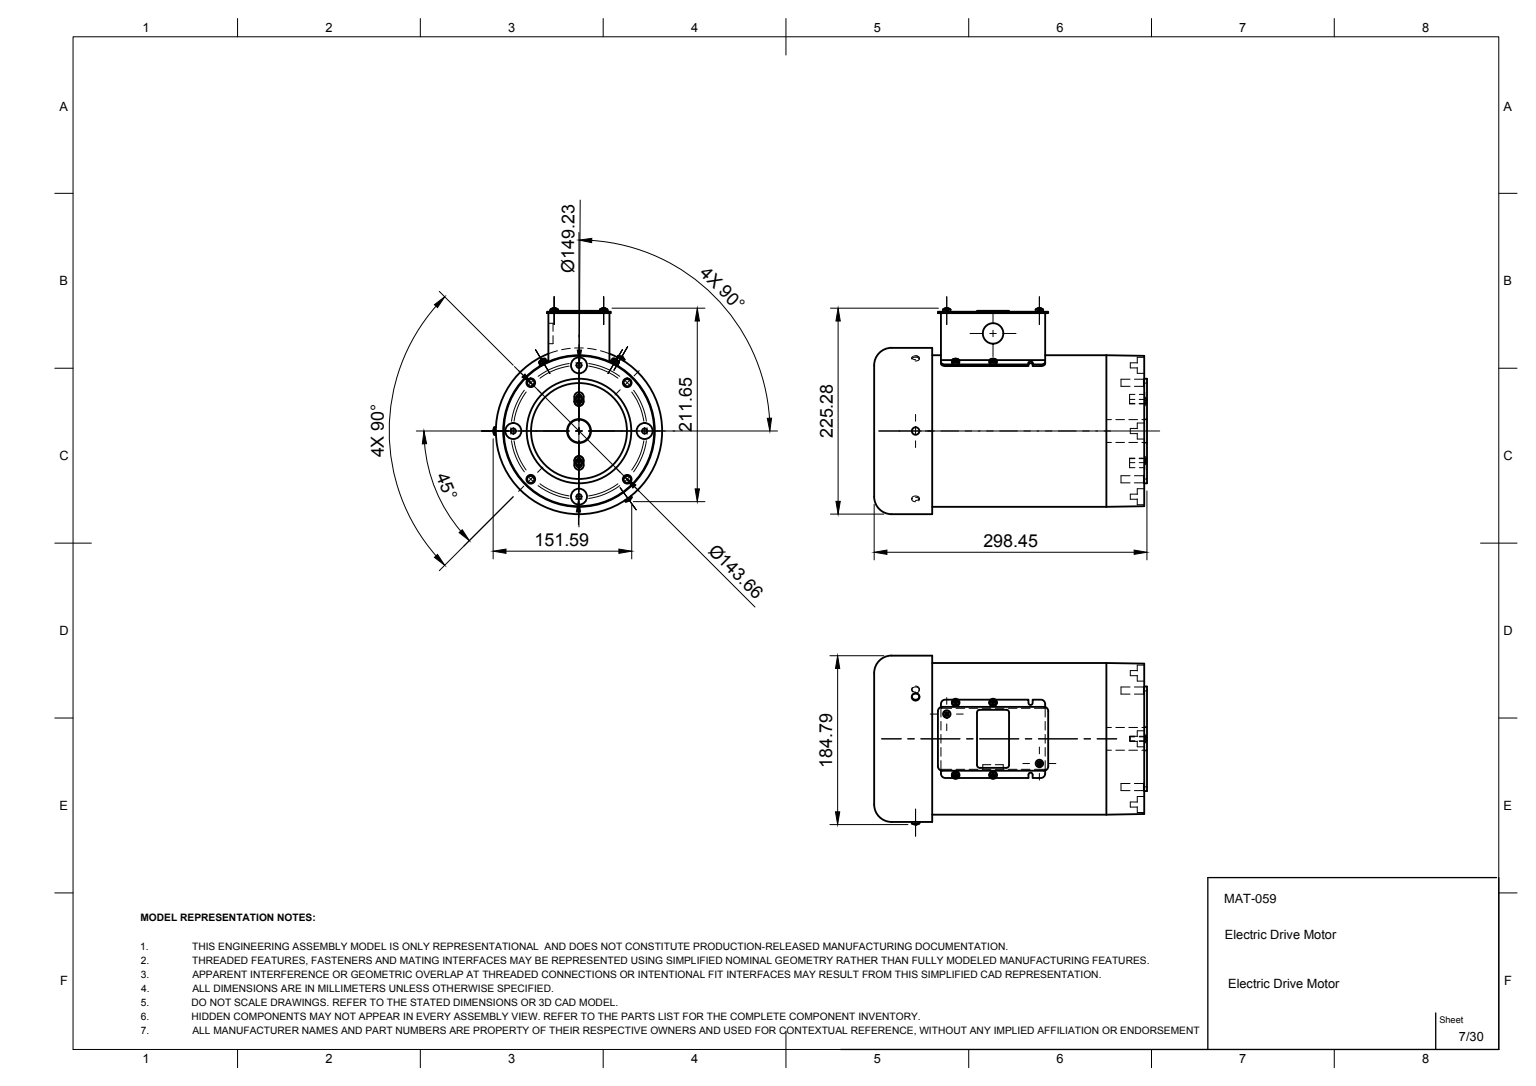
ISO-10303-21;
HEADER;
/* Generated by software containing ST-Developer
 * from STEP Tools, Inc. (www.steptools.com) 
 */

FILE_DESCRIPTION(
/* description */ ('', 'CAx-IF Rec.Pracs.---Representation and Presentation of Product Manufa
cturing Information (PMI)---4.0---2014-10-13'),
/* implementation_level */ '2;1');

FILE_NAME(
/* name */ 'Electric Drive Motor.step',
/* time_stamp */ '2026-10-28T23:00:48+01:00',
/* author */ (''),
/* organization */ (''),
/* preprocessor_version */ 'ST-DEVELOPER v20.2',
/* originating_system */ 'Autodesk Translation Framework v15.17.0.0',
/* authorisation */ '');

FILE_SCHEMA (('AP242_MANAGED_MODEL_BASED_3D_ENGINEERING_MIM_LF { 1 0 10303 442 2 1 4 }'));
ENDSEC;

DATA;
#10=MECHANICAL_DESIGN_GEOMETRIC_PRESENTATION_REPRESENTATION('',(#969),#61811);
#509=(
BOUNDED_CURVE()
B_SPLINE_CURVE(2,(#51599,#51600,#51601),.UNSPECIFIED.,.F.,.F.)
B_SPLINE_CURVE_WITH_KNOTS((3,3),(-1.09670001953998,-0.838836123214499),
 .UNSPECIFIED.)
CURVE()
GEOMETRIC_REPRESENTATION_ITEM()
RATIONAL_B_SPLINE_CURVE((0.975084512183132,0.979302933905043,1.))
REPRESENTATION_ITEM('')
);
#510=(
BOUNDED_CURVE()
B_SPLINE_CURVE(2,(#52725,#52726,#52727,#52728,#52729),.UNSPECIFIED.,.F.,
 .F.)
B_SPLINE_CURVE_WITH_KNOTS((3,2,3),(4.71238779043687,5.49778654880823,6.28318530717959),
 .UNSPECIFIED.)
CURVE()
GEOMETRIC_REPRESENTATION_ITEM()
RATIONAL_B_SPLINE_CURVE((1.,0.923879418659198,1.,0.923879418650411,1.))
REPRESENTATION_ITEM('')
);
#578=CONICAL_SURFACE('',#34877,3.98868900000005,0.78539816339748);
#579=CONICAL_SURFACE('',#34884,3.98868900000002,0.785398163397457);
#580=CONICAL_SURFACE('',#34891,3.98868900000004,0.785398163397464);
#581=CONICAL_SURFACE('',#34898,3.98868900000001,0.785398163397455);
#582=CONICAL_SURFACE('',#34900,82.8587325401841,0.0174532925199438);
#726=SPHERICAL_SURFACE('',#34596,6.41240517241364);
#727=SPHERICAL_SURFACE('',#34645,6.41240517241439);
#728=SPHERICAL_SURFACE('',#34685,6.4992807017556);
#729=SPHERICAL_SURFACE('',#34700,6.49928070175542);
#730=SPHERICAL_SURFACE('',#34786,6.41240517241381);
#731=SPHERICAL_SURFACE('',#34971,5.68734575000013);
#732=SPHERICAL_SURFACE('',#34992,5.68734575000012);
#778=B_SPLINE_CURVE_WITH_KNOTS('',3,(#51594,#51595,#51596,#51597),
 .UNSPECIFIED.,.F.,.F.,(4,4),(3.08084590110894,3.12989709501739),
 .UNSPECIFIED.);
#779=B_SPLINE_CURVE_WITH_KNOTS('',3,(#51606,#51607,#51608,#51609),
 .UNSPECIFIED.,.F.,.F.,(4,4),(3.03179470720155,3.08084590110894),
 .UNSPECIFIED.);
#780=B_SPLINE_CURVE_WITH_KNOTS('',3,(#51611,#51612,#51613,#51614,#51615,
#51616,#51617,#51618),.UNSPECIFIED.,.F.,.F.,(4,2,2,4),(-0.281543316074503,
-0.256347073285161,-0.128173536642581,-0.0492557161192092),
 .UNSPECIFIED.);
#781=B_SPLINE_CURVE_WITH_KNOTS('',3,(#51620,#51621,#51622,#51623,#51624,
#51625,#51626,#51627),.UNSPECIFIED.,.F.,.F.,(4,2,2,4),(-3.44463382971284,
-3.36571600918869,-3.23754247254589,-3.21234622975666),.UNSPECIFIED.);
#782=B_SPLINE_CURVE_WITH_KNOTS('',3,(#51629,#51630,#51631,#51632,#51633,
#51634,#51635),.UNSPECIFIED.,.F.,.F.,(4,3,4),(-0.0490511939078948,0.,0.0490511939079084),
 .UNSPECIFIED.);
#783=B_SPLINE_CURVE_WITH_KNOTS('',3,(#51637,#51638,#51639,#51640,#51641,
#51642,#51643,#51644),.UNSPECIFIED.,.F.,.F.,(4,2,2,4),(-0.281543316073918,
-0.256347073285632,-0.128173536642816,-0.0492557161186468),
 .UNSPECIFIED.);
#784=B_SPLINE_CURVE_WITH_KNOTS('',3,(#51646,#51647,#51648,#51649,#51650,
#51651,#51652,#51653),.UNSPECIFIED.,.F.,.F.,(4,2,2,4),(-3.44463382971226,
-3.36571600918894,-3.23754247254636,-3.21234622975697),.UNSPECIFIED.);
#785=B_SPLINE_CURVE_WITH_KNOTS('',3,(#51655,#51656,#51657,#51658,#51659,
#51660,#51661),.UNSPECIFIED.,.F.,.F.,(4,3,4),(-0.0490511939073931,0.,0.0490511939084528),
 .UNSPECIFIED.);
#786=B_SPLINE_CURVE_WITH_KNOTS('',3,(#51663,#51664,#51665,#51666,#51667,
#51668,#51669,#51670),.UNSPECIFIED.,.F.,.F.,(4,2,2,4),(-0.281543316074568,
-0.256347073286048,-0.128173536643024,-0.0492557161192777),
 .UNSPECIFIED.);
#787=B_SPLINE_CURVE_WITH_KNOTS('',3,(#51672,#51673,#51674,#51675,#51676,
#51677,#51678,#51679),.UNSPECIFIED.,.F.,.F.,(4,2,2,4),(-3.44463382971165,
-3.36571600918866,-3.23754247254584,-3.21234622975546),.UNSPECIFIED.);
#788=B_SPLINE_CURVE_WITH_KNOTS('',3,(#51681,#51682,#51683,#51684,#51685,
#51686,#51687),.UNSPECIFIED.,.F.,.F.,(4,3,4),(-0.0490511939080049,0.,0.0490511939079151),
 .UNSPECIFIED.);
#789=B_SPLINE_CURVE_WITH_KNOTS('',3,(#51689,#51690,#51691,#51692,#51693,
#51694,#51695,#51696),.UNSPECIFIED.,.F.,.F.,(4,2,2,4),(-0.281543316075136,
-0.25634707328559,-0.128173536642795,-0.049255716119827),.UNSPECIFIED.);
#790=B_SPLINE_CURVE_WITH_KNOTS('',3,(#51697,#51698,#51699,#51700,#51701,
#51702,#51703,#51704),.UNSPECIFIED.,.F.,.F.,(4,2,2,4),(-3.44463382971222,
-3.36571600918842,-3.23754247254539,-3.21234622975693),.UNSPECIFIED.);
#791=B_SPLINE_CURVE_WITH_KNOTS('',3,(#51727,#51728,#51729,#51730,#51731,
#51732,#51733,#51734,#51735,#51736),.UNSPECIFIED.,.F.,.F.,(4,2,2,2,4),(-1.23367624376484,
-1.07962569003998,-0.925575136315127,-0.771400514278829,-0.617225892242532),
 .UNSPECIFIED.);
#792=B_SPLINE_CURVE_WITH_KNOTS('',3,(#51737,#51738,#51739,#51740,#51741,
#51742,#51743,#51744,#51745,#51746),.UNSPECIFIED.,.F.,.F.,(4,2,2,2,4),(-1.85012659645245,
-1.69593736206289,-1.54174812767333,-1.38771218571909,-1.23367624376484),
 .UNSPECIFIED.);
#793=B_SPLINE_CURVE_WITH_KNOTS('',3,(#51752,#51753,#51754,#51755,#51756,
#51757,#51758,#51759,#51760,#51761),.UNSPECIFIED.,.F.,.F.,(4,2,2,2,4),(2.30953959739069,
2.51054404549657,2.71154849360245,2.89942800416522,3.08730751472799),
 .UNSPECIFIED.);
#794=B_SPLINE_CURVE_WITH_KNOTS('',3,(#51767,#51768,#51769,#51770,#51771,
#51772,#51773,#51774,#51775,#51776,#51777,#51778,#51779,#51780,#51781,#51782,
#51783,#51784),.UNSPECIFIED.,.F.,.F.,(4,2,2,2,2,2,2,2,4),(0.368633646558617,
0.466000906670528,0.563368166782438,0.648915734055293,0.734463301328148,
0.820010868601003,0.905558435873858,1.00292569598577,1.10029295609768),
 .UNSPECIFIED.);
#795=B_SPLINE_CURVE_WITH_KNOTS('',3,(#51790,#51791,#51792,#51793,#51794,
#51795,#51796,#51797,#51798,#51799),.UNSPECIFIED.,.F.,.F.,(4,2,2,2,4),(-1.77635683940028E-15,
0.181238959345487,0.362477918690977,0.570076776395974,0.777675634100972),
 .UNSPECIFIED.);
#796=B_SPLINE_CURVE_WITH_KNOTS('',3,(#51805,#51806,#51807,#51808,#51809,
#51810,#51811,#51812,#51813,#51814),.UNSPECIFIED.,.F.,.F.,(4,2,2,2,4),(0.617225892242314,
0.771400514278674,0.925575136315034,1.07962569003995,1.23367624376487),
 .UNSPECIFIED.);
#797=B_SPLINE_CURVE_WITH_KNOTS('',3,(#51817,#51818,#51819,#51820,#51821,
#51822,#51823,#51824,#51825,#51826),.UNSPECIFIED.,.F.,.F.,(4,2,2,2,4),(1.23367624376487,
1.38771218571906,1.54174812767325,1.69593736206276,1.85012659645227),
 .UNSPECIFIED.);
#798=B_SPLINE_CURVE_WITH_KNOTS('',3,(#51832,#51833,#51834,#51835,#51836,
#51837,#51838,#51839,#51840,#51841,#51842,#51843,#51844,#51845,#51846,#51847,
#51848,#51849,#51850),.UNSPECIFIED.,.F.,.F.,(4,2,2,2,3,2,2,2,4),(-0.366794796562496,
-0.268922616838031,-0.171050437113567,-0.0855252185567822,2.33146835171283E-15,
0.0855252185567869,0.171050437113571,0.268922616838036,0.366794796562501),
 .UNSPECIFIED.);
#799=B_SPLINE_CURVE_WITH_KNOTS('',3,(#51854,#51855,#51856,#51857,#51858,
#51859,#51860,#51861,#51862,#51863,#51864,#51865,#51866,#51867,#51868,#51869,
#51870,#51871,#51872),.UNSPECIFIED.,.F.,.F.,(4,2,2,2,3,2,2,2,4),(-0.365829654769541,
-0.268462394657629,-0.171095134545717,-0.0855475672728611,-5.21804821573824E-15,
0.0882774493987044,0.176554898797414,0.271203483898993,0.365852069000572),
 .UNSPECIFIED.);
#800=B_SPLINE_CURVE_WITH_KNOTS('',3,(#51876,#51877,#51878,#51879,#51880,
#51881,#51882,#51883,#51884,#51885,#51886,#51887,#51888,#51889,#51890,#51891,
#51892,#51893),.UNSPECIFIED.,.F.,.F.,(4,2,2,2,2,2,2,2,4),(-1.10334360967883,
-1.00547142995437,-0.907599250229903,-0.822074031673119,-0.736548813116335,
-0.651023594559552,-0.565498376002768,-0.467626196278304,-0.369754016553839),
 .UNSPECIFIED.);
#801=B_SPLINE_CURVE_WITH_KNOTS('',3,(#51900,#51901,#51902,#51903,#51904,
#51905,#51906,#51907,#51908,#51909),.UNSPECIFIED.,.F.,.F.,(4,2,2,2,4),(0.,
0.181230618131972,0.362461236263944,0.571238472910728,0.780015709557511),
 .UNSPECIFIED.);
#802=B_SPLINE_CURVE_WITH_KNOTS('',3,(#51912,#51913,#51914,#51915,#51916,
#51917,#51918,#51919,#51920,#51921),.UNSPECIFIED.,.F.,.F.,(4,2,2,2,4),(-2.32129720255586,
-2.11369834485087,-1.90609948714587,-1.72486052780038,-1.54362156845489),
 .UNSPECIFIED.);
#803=B_SPLINE_CURVE_WITH_KNOTS('',3,(#51939,#51940,#51941,#51942,#51943,
#51944,#51945,#51946,#51947,#51948),.UNSPECIFIED.,.F.,.F.,(4,2,2,2,4),(-1.85012659645253,
-1.69593736206296,-1.54174812767339,-1.38771218571914,-1.23367624376489),
 .UNSPECIFIED.);
#804=B_SPLINE_CURVE_WITH_KNOTS('',3,(#51952,#51953,#51954,#51955,#51956,
#51957,#51958,#51959,#51960,#51961),.UNSPECIFIED.,.F.,.F.,(4,2,2,2,4),(-1.23367624376489,
-1.07962569004007,-0.925575136315257,-0.771400514279,-0.617225892242743),
 .UNSPECIFIED.);
#805=B_SPLINE_CURVE_WITH_KNOTS('',3,(#51971,#51972,#51973,#51974,#51975,
#51976,#51977,#51978,#51979,#51980),.UNSPECIFIED.,.F.,.F.,(4,2,2,2,4),(1.54359366303678,
1.73147317359955,1.91935268416232,2.1203571322682,2.32136158037408),
 .UNSPECIFIED.);
#806=B_SPLINE_CURVE_WITH_KNOTS('',3,(#51989,#51990,#51991,#51992,#51993,
#51994,#51995,#51996,#51997,#51998),.UNSPECIFIED.,.F.,.F.,(4,2,2,2,4),(1.23367624376487,
1.38771218571901,1.54174812767315,1.69593736206261,1.85012659645207),
 .UNSPECIFIED.);
#807=B_SPLINE_CURVE_WITH_KNOTS('',3,(#51999,#52000,#52001,#52002,#52003,
#52004,#52005,#52006,#52007,#52008),.UNSPECIFIED.,.F.,.F.,(4,2,2,2,4),(0.617225892242314,
0.771400514278675,0.925575136315035,1.07962569003995,1.23367624376487),
 .UNSPECIFIED.);
#808=B_SPLINE_CURVE_WITH_KNOTS('',3,(#52138,#52139,#52140,#52141,#52142,
#52143,#52144,#52145,#52146,#52147),.UNSPECIFIED.,.F.,.F.,(4,2,2,2,4),(1.54763785217733,
1.73581526281001,1.92399267344269,2.12587396957551,2.32775526570834),
 .UNSPECIFIED.);
#809=B_SPLINE_CURVE_WITH_KNOTS('',3,(#52454,#52455,#52456,#52457,#52458,
#52459,#52460,#52461,#52462,#52463),.UNSPECIFIED.,.F.,.F.,(4,2,2,2,4),(0.767622142619809,
0.976399379266592,1.18517661591337,1.36640723404535,1.54763785217732),
 .UNSPECIFIED.);
#810=B_SPLINE_CURVE_WITH_KNOTS('',3,(#52478,#52479,#52480,#52481,#52482,
#52483,#52484,#52485,#52486,#52487),.UNSPECIFIED.,.F.,.F.,(4,2,2,2,4),(2.31525999479713,
2.52403723144391,2.73281446809069,2.91404508622267,3.09527570435464),
 .UNSPECIFIED.);
#811=B_SPLINE_CURVE_WITH_KNOTS('',3,(#52630,#52631,#52632,#52633,#52634,
#52635,#52636,#52637,#52638,#52639,#52640,#52641,#52642,#52643,#52644,#52645,
#52646,#52647),.UNSPECIFIED.,.F.,.F.,(4,2,2,2,2,2,2,2,4),(-1.24400278846932,
-1.08850242875974,-0.933002069050166,-0.777501731642414,-0.622001394234663,
-0.46650105682691,-0.311000719419158,-0.155500359709579,0.),
 .UNSPECIFIED.);
#812=B_SPLINE_CURVE_WITH_KNOTS('',3,(#52653,#52654,#52655,#52656,#52657,
#52658,#52659,#52660,#52661,#52662,#52663,#52664,#52665,#52666,#52667,#52668,
#52669,#52670),.UNSPECIFIED.,.F.,.F.,(4,2,2,2,2,2,2,2,4),(0.,0.155500359709579,
0.311000719419159,0.46650105682691,0.622001394234662,0.777501731642413,
0.933002069050164,1.08850242875974,1.24400278846933),.UNSPECIFIED.);
#813=B_SPLINE_CURVE_WITH_KNOTS('',3,(#52679,#52680,#52681,#52682,#52683,
#52684,#52685,#52686,#52687,#52688,#52689,#52690,#52691,#52692,#52693,#52694,
#52695,#52696),.UNSPECIFIED.,.F.,.F.,(4,2,2,2,2,2,2,2,4),(-1.24400278846934,
-1.08850242875976,-0.933002069050176,-0.777501731642423,-0.622001394234669,
-0.466501056826915,-0.311000719419162,-0.155500359709581,0.),
 .UNSPECIFIED.);
#814=B_SPLINE_CURVE_WITH_KNOTS('',3,(#52702,#52703,#52704,#52705,#52706,
#52707,#52708,#52709,#52710,#52711,#52712,#52713,#52714,#52715,#52716,#52717,
#52718,#52719),.UNSPECIFIED.,.F.,.F.,(4,2,2,2,2,2,2,2,4),(0.,0.155500359709582,
0.311000719419163,0.466501056826916,0.622001394234669,0.777501731642423,
0.933002069050176,1.08850242875976,1.24400278846934),.UNSPECIFIED.);
#815=B_SPLINE_CURVE_WITH_KNOTS('',3,(#52734,#52735,#52736,#52737,#52738,
#52739,#52740,#52741,#52742,#52743,#52744,#52745,#52746,#52747,#52748,#52749,
#52750,#52751),.UNSPECIFIED.,.F.,.F.,(4,2,2,2,2,2,2,2,4),(-1.24400278846932,
-1.08850242875974,-0.933002069050164,-0.777501731642413,-0.622001394234661,
-0.46650105682691,-0.311000719419158,-0.155500359709579,0.),
 .UNSPECIFIED.);
#816=B_SPLINE_CURVE_WITH_KNOTS('',3,(#52755,#52756,#52757,#52758,#52759,
#52760,#52761,#52762,#52763,#52764,#52765,#52766,#52767,#52768,#52769,#52770,
#52771,#52772),.UNSPECIFIED.,.F.,.F.,(4,2,2,2,2,2,2,2,4),(0.,0.15550035970958,
0.311000719419159,0.466501056826911,0.622001394234662,0.777501731642413,
0.933002069050165,1.08850242875974,1.24400278846932),.UNSPECIFIED.);
#870=(
BOUNDED_SURFACE()
B_SPLINE_SURFACE(2,2,((#51565,#51566,#51567,#51568,#51569,#51570,#51571,
#51572,#51573),(#51574,#51575,#51576,#51577,#51578,#51579,#51580,#51581,
#51582),(#51583,#51584,#51585,#51586,#51587,#51588,#51589,#51590,#51591)),
 .UNSPECIFIED.,.F.,.T.,.F.)
B_SPLINE_SURFACE_WITH_KNOTS((3,3),(3,2,2,2,3),(-1.48658674941058,-0.838836123214499),
(-3.14159265358979,-1.5707963267949,0.,1.5707963267949,3.14159265358979),
 .UNSPECIFIED.)
GEOMETRIC_REPRESENTATION_ITEM()
RATIONAL_B_SPLINE_SURFACE(((1.,0.707106781186548,1.,0.707106781186548,1.,
0.707106781186548,1.,0.707106781186548,1.),(0.948009249396791,0.67034376887604,
0.948009249396791,0.67034376887604,0.948009249396791,0.67034376887604,0.948009249396791,
0.67034376887604,0.948009249396791),(1.,0.707106781186548,1.,0.707106781186548,
1.,0.707106781186548,1.,0.707106781186548,1.)))
REPRESENTATION_ITEM('')
SURFACE()
);
#871=(
BOUNDED_SURFACE()
B_SPLINE_SURFACE(2,2,((#52773,#52774,#52775,#52776,#52777,#52778,#52779,
#52780,#52781),(#52782,#52783,#52784,#52785,#52786,#52787,#52788,#52789,
#52790),(#52791,#52792,#52793,#52794,#52795,#52796,#52797,#52798,#52799)),
 .UNSPECIFIED.,.F.,.T.,.F.)
B_SPLINE_SURFACE_WITH_KNOTS((3,3),(3,2,2,2,3),(-1.57079634483717,-0.955666854650568),
(-3.14159265358979,-1.5707963267949,0.,1.5707963267949,3.14159265358979),
 .UNSPECIFIED.)
GEOMETRIC_REPRESENTATION_ITEM()
RATIONAL_B_SPLINE_SURFACE(((1.,0.707106781186548,1.,0.707106781186548,1.,
0.707106781186548,1.,0.707106781186548,1.),(0.953073640802859,0.673924834381854,
0.953073640802859,0.673924834381854,0.953073640802859,0.673924834381854,
0.953073640802859,0.673924834381854,0.953073640802859),(1.,0.707106781186548,
1.,0.707106781186548,1.,0.707106781186548,1.,0.707106781186548,1.)))
REPRESENTATION_ITEM('')
SURFACE()
);
#872=(
BOUNDED_SURFACE()
B_SPLINE_SURFACE(2,2,((#52806,#52807,#52808,#52809,#52810,#52811,#52812,
#52813,#52814),(#52815,#52816,#52817,#52818,#52819,#52820,#52821,#52822,
#52823),(#52824,#52825,#52826,#52827,#52828,#52829,#52830,#52831,#52832)),
 .UNSPECIFIED.,.F.,.T.,.F.)
B_SPLINE_SURFACE_WITH_KNOTS((3,3),(3,2,2,2,3),(-1.57079630698122,-0.955666850767325),
(-3.14159265358979,-1.5707963267949,0.,1.5707963267949,3.14159265358979),
 .UNSPECIFIED.)
GEOMETRIC_REPRESENTATION_ITEM()
RATIONAL_B_SPLINE_SURFACE(((1.,0.707106781186548,1.,0.707106781186548,1.,
0.707106781186548,1.,0.707106781186548,1.),(0.953073645945215,0.673924838018048,
0.953073645945215,0.673924838018048,0.953073645945215,0.673924838018048,
0.953073645945215,0.673924838018048,0.953073645945215),(1.,0.707106781186548,
1.,0.707106781186548,1.,0.707106781186548,1.,0.707106781186548,1.)))
REPRESENTATION_ITEM('')
SURFACE()
);
#873=(
BOUNDED_SURFACE()
B_SPLINE_SURFACE(2,2,((#52834,#52835,#52836,#52837,#52838,#52839,#52840,
#52841,#52842),(#52843,#52844,#52845,#52846,#52847,#52848,#52849,#52850,
#52851),(#52852,#52853,#52854,#52855,#52856,#52857,#52858,#52859,#52860)),
 .UNSPECIFIED.,.F.,.T.,.F.)
B_SPLINE_SURFACE_WITH_KNOTS((3,3),(3,2,2,2,3),(-1.57079632708437,-0.955666871754965),
(-3.14159265358979,-1.5707963267949,0.,1.5707963267949,3.14159265358979),
 .UNSPECIFIED.)
GEOMETRIC_REPRESENTATION_ITEM()
RATIONAL_B_SPLINE_SURFACE(((1.,0.707106781186548,1.,0.707106781186548,1.,
0.707106781186548,1.,0.707106781186548,1.),(0.953073646079135,0.673924838112744,
0.953073646079135,0.673924838112744,0.953073646079135,0.673924838112744,
0.953073646079135,0.673924838112744,0.953073646079135),(1.,0.707106781186548,
1.,0.707106781186548,1.,0.707106781186548,1.,0.707106781186548,1.)))
REPRESENTATION_ITEM('')
SURFACE()
);
#895=TOROIDAL_SURFACE('',#34831,71.8820000000001,19.0499999999999);
#919=SHAPE_REPRESENTATION_RELATIONSHIP('SRR','None',#61977,#944);
#944=ADVANCED_BREP_SHAPE_REPRESENTATION('',(#1008),#61790);
#969=STYLED_ITEM('',(#62142),#1008);
#1008=MANIFOLD_SOLID_BREP('Body1',#33799);
#1107=CYLINDRICAL_SURFACE('',#34576,4.08939999999975);
#1108=CYLINDRICAL_SURFACE('',#34577,84.4550000000046);
#1109=CYLINDRICAL_SURFACE('',#34582,2.286);
#1110=CYLINDRICAL_SURFACE('',#34583,2.286);
#1111=CYLINDRICAL_SURFACE('',#34584,4.82600000000001);
#1112=CYLINDRICAL_SURFACE('',#34587,4.08939999999991);
#1113=CYLINDRICAL_SURFACE('',#34590,84.455000000012);
#1114=CYLINDRICAL_SURFACE('',#34615,4.08939999999986);
#1115=CYLINDRICAL_SURFACE('',#34617,4.08939999999985);
#1116=CYLINDRICAL_SURFACE('',#34647,4.82600000000001);
#1117=CYLINDRICAL_SURFACE('',#34648,4.826);
#1118=CYLINDRICAL_SURFACE('',#34652,4.82599999999999);
#1119=CYLINDRICAL_SURFACE('',#34656,4.82600000000005);
#1120=CYLINDRICAL_SURFACE('',#34660,4.82600000000005);
#1121=CYLINDRICAL_SURFACE('',#34672,3.04799999999982);
#1122=CYLINDRICAL_SURFACE('',#34675,3.04799999999992);
#1123=CYLINDRICAL_SURFACE('',#34678,3.048);
#1124=CYLINDRICAL_SURFACE('',#34681,3.04800000000001);
#1125=CYLINDRICAL_SURFACE('',#34699,4.08940000000001);
#1126=CYLINDRICAL_SURFACE('',#34714,4.0894);
#1127=CYLINDRICAL_SURFACE('',#34751,4.826);
#1128=CYLINDRICAL_SURFACE('',#34757,4.826);
#1129=CYLINDRICAL_SURFACE('',#34781,11.1759999999998);
#1130=CYLINDRICAL_SURFACE('',#34811,4.12749999999997);
#1131=CYLINDRICAL_SURFACE('',#34817,4.12750000000001);
#1132=CYLINDRICAL_SURFACE('',#34823,4.12749999999996);
#1133=CYLINDRICAL_SURFACE('',#34836,90.9319999999999);
#1134=CYLINDRICAL_SURFACE('',#34840,82.931);
#1135=CYLINDRICAL_SURFACE('',#34855,5.08000000000016);
#1136=CYLINDRICAL_SURFACE('',#34858,5.08000000000021);
#1137=CYLINDRICAL_SURFACE('',#34866,5.08);
#1138=CYLINDRICAL_SURFACE('',#34869,5.08000000000001);
#1139=CYLINDRICAL_SURFACE('',#34874,3.90270999999991);
#1140=CYLINDRICAL_SURFACE('',#34881,3.90270999999999);
#1141=CYLINDRICAL_SURFACE('',#34888,3.90271000000012);
#1142=CYLINDRICAL_SURFACE('',#34895,3.90271);
#1143=CYLINDRICAL_SURFACE('',#34908,57.15);
#1144=CYLINDRICAL_SURFACE('',#34912,52.451);
#1145=CYLINDRICAL_SURFACE('',#34916,13.081);
#1146=CYLINDRICAL_SURFACE('',#34920,12.446);
#1147=CYLINDRICAL_SURFACE('',#34924,8.76299999999995);
#1148=CYLINDRICAL_SURFACE('',#34925,2.794);
#1149=CYLINDRICAL_SURFACE('',#34928,8.76299999999997);
#1150=CYLINDRICAL_SURFACE('',#34932,2.794);
#1151=CYLINDRICAL_SURFACE('',#34937,2.79400000000002);
#1152=CYLINDRICAL_SURFACE('',#34941,8.76300000000001);
#1153=CYLINDRICAL_SURFACE('',#34942,8.763);
#1154=CYLINDRICAL_SURFACE('',#34946,2.79399999999998);
#1155=CYLINDRICAL_SURFACE('',#34950,2.76860000000046);
#1156=CYLINDRICAL_SURFACE('',#34958,2.7686);
#1157=CYLINDRICAL_SURFACE('',#34960,2.76860000000001);
#1158=CYLINDRICAL_SURFACE('',#34961,2.76860000000061);
#1159=CYLINDRICAL_SURFACE('',#34965,4.73709999999997);
#1160=CYLINDRICAL_SURFACE('',#34968,2.18439999999999);
#1161=CYLINDRICAL_SURFACE('',#34989,2.18440000000006);
#1162=CYLINDRICAL_SURFACE('',#34990,4.73710000000002);
#1923=FACE_BOUND('',#6409,.T.);
#1924=FACE_BOUND('',#6410,.T.);
#1925=FACE_BOUND('',#6418,.T.);
#1926=FACE_BOUND('',#6419,.T.);
#1927=FACE_BOUND('',#6422,.T.);
#1928=FACE_BOUND('',#6442,.T.);
#1929=FACE_BOUND('',#6454,.T.);
#1930=FACE_BOUND('',#6456,.T.);
#1931=FACE_BOUND('',#6457,.T.);
#1932=FACE_BOUND('',#6458,.T.);
#1933=FACE_BOUND('',#6469,.T.);
#1934=FACE_BOUND('',#6472,.T.);
#1935=FACE_BOUND('',#6521,.T.);
#1936=FACE_BOUND('',#6539,.T.);
#1937=FACE_BOUND('',#6552,.T.);
#1938=FACE_BOUND('',#6564,.T.);
#1939=FACE_BOUND('',#6565,.T.);
#1940=FACE_BOUND('',#6566,.T.);
#1941=FACE_BOUND('',#6570,.T.);
#1942=FACE_BOUND('',#6577,.T.);
#1943=FACE_BOUND('',#6583,.T.);
#1944=FACE_BOUND('',#6602,.T.);
#1945=FACE_BOUND('',#6603,.T.);
#1946=FACE_BOUND('',#6604,.T.);
#1947=FACE_BOUND('',#6605,.T.);
#1948=FACE_BOUND('',#6606,.T.);
#1949=FACE_BOUND('',#6607,.T.);
#1950=FACE_BOUND('',#6608,.T.);
#1951=FACE_BOUND('',#6609,.T.);
#1952=FACE_BOUND('',#6610,.T.);
#1953=FACE_BOUND('',#6613,.T.);
#1954=FACE_BOUND('',#6616,.T.);
#1955=FACE_BOUND('',#6617,.T.);
#1956=FACE_BOUND('',#6618,.T.);
#1957=FACE_BOUND('',#6621,.T.);
#1958=FACE_BOUND('',#6624,.T.);
#1959=FACE_BOUND('',#6630,.T.);
#1960=FACE_BOUND('',#6636,.T.);
#1961=FACE_BOUND('',#6640,.T.);
#1962=FACE_BOUND('',#6647,.T.);
#1963=FACE_BOUND('',#6652,.T.);
#1964=FACE_BOUND('',#6656,.T.);
#1965=FACE_BOUND('',#6658,.T.);
#1966=FACE_BOUND('',#6660,.T.);
#1967=FACE_BOUND('',#6664,.T.);
#2448=CIRCLE('',#34569,4.08939999999988);
#2449=CIRCLE('',#34570,4.08939999999988);
#2450=CIRCLE('',#34575,4.0893999999995);
#2451=CIRCLE('',#34578,84.4550000000159);
#2452=CIRCLE('',#34579,84.4549999999612);
#2453=CIRCLE('',#34580,84.4549999999434);
#2454=CIRCLE('',#34581,84.4550000000244);
#2455=CIRCLE('',#34588,4.08940000000003);
#2456=CIRCLE('',#34589,4.08939999999987);
#2457=CIRCLE('',#34591,84.4549999999862);
#2458=CIRCLE('',#34592,84.4550000001664);
#2459=CIRCLE('',#34593,84.4550000000658);
#2460=CIRCLE('',#34594,84.4549999999639);
#2461=CIRCLE('',#34597,5.73418625921224);
#2462=CIRCLE('',#34598,6.39225125407266);
#2463=CIRCLE('',#34599,6.39225125407329);
#2464=CIRCLE('',#34600,5.73418625920595);
#2465=CIRCLE('',#34601,6.39225125407447);
#2466=CIRCLE('',#34602,6.39225125407165);
#2467=CIRCLE('',#34603,5.73418625919979);
#2468=CIRCLE('',#34604,6.39225125407114);
#2469=CIRCLE('',#34605,6.39225125407334);
#2470=CIRCLE('',#34606,5.73418625920593);
#2471=CIRCLE('',#34607,6.3922512540724);
#2472=CIRCLE('',#34608,6.39225125407298);
#2473=CIRCLE('',#34610,6.3922512540739);
#2474=CIRCLE('',#34612,5.73418625919449);
#2475=CIRCLE('',#34614,4.08939999999995);
#2476=CIRCLE('',#34616,4.08939999999987);
#2477=CIRCLE('',#34618,4.08939999999931);
#2478=CIRCLE('',#34619,4.08939999999987);
#2479=CIRCLE('',#34621,6.39225125406976);
#2480=CIRCLE('',#34623,5.7341862591997);
#2481=CIRCLE('',#34625,6.39225125407312);
#2482=CIRCLE('',#34627,6.39225125407987);
#2483=CIRCLE('',#34629,5.73418625919762);
#2484=CIRCLE('',#34631,6.39225125407758);
#2485=CIRCLE('',#34633,6.39225125407361);
#2486=CIRCLE('',#34635,5.73418625916851);
#2487=CIRCLE('',#34637,6.39225125407298);
#2488=CIRCLE('',#34639,6.39225125407049);
#2489=CIRCLE('',#34641,5.73418625919762);
#2490=CIRCLE('',#34643,6.3922512540717);
#2491=CIRCLE('',#34649,4.82600000000001);
#2492=CIRCLE('',#34650,4.82600000000001);
#2493=CIRCLE('',#34653,4.82600000000004);
#2494=CIRCLE('',#34654,4.82599999999999);
#2495=CIRCLE('',#34657,4.82600000000005);
#2496=CIRCLE('',#34658,4.82600000000005);
#2497=CIRCLE('',#34661,4.82600000000003);
#2498=CIRCLE('',#34662,4.82599999999998);
#2499=CIRCLE('',#34666,4.0894);
#2500=CIRCLE('',#34667,4.08940000000001);
#2501=CIRCLE('',#34668,3.04799999999999);
#2502=CIRCLE('',#34669,3.04799999999999);
#2503=CIRCLE('',#34670,3.04800000000004);
#2504=CIRCLE('',#34671,3.04800000000004);
#2505=CIRCLE('',#34673,3.04799999999999);
#2506=CIRCLE('',#34676,3.04799999999999);
#2507=CIRCLE('',#34679,3.04800000000004);
#2508=CIRCLE('',#34682,3.04800000000004);
#2509=CIRCLE('',#34686,4.08940000000001);
#2510=CIRCLE('',#34687,6.47939701209842);
#2511=CIRCLE('',#34688,5.83117497592219);
#2512=CIRCLE('',#34689,6.47939701210061);
#2513=CIRCLE('',#34690,6.47939701209921);
#2514=CIRCLE('',#34691,5.83117497591494);
#2515=CIRCLE('',#34692,6.4793970120992);
#2516=CIRCLE('',#34693,6.47939701210015);
#2517=CIRCLE('',#34694,5.83117497591959);
#2518=CIRCLE('',#34695,6.47939701209921);
#2519=CIRCLE('',#34696,6.47939701209916);
#2520=CIRCLE('',#34697,5.83117497592765);
#2521=CIRCLE('',#34698,6.479397012098);
#2522=CIRCLE('',#34701,4.0894);
#2523=CIRCLE('',#34702,6.47939701209688);
#2524=CIRCLE('',#34703,5.83117497592362);
#2525=CIRCLE('',#34704,6.47939701209502);
#2526=CIRCLE('',#34705,6.47939701209653);
#2527=CIRCLE('',#34706,5.83117497590882);
#2528=CIRCLE('',#34707,6.47939701209738);
#2529=CIRCLE('',#34708,6.47939701209747);
#2530=CIRCLE('',#34709,5.83117497591427);
#2531=CIRCLE('',#34710,6.47939701209745);
#2532=CIRCLE('',#34711,6.47939701209746);
#2533=CIRCLE('',#34712,5.83117497591896);
#2534=CIRCLE('',#34713,6.47939701209731);
#2535=CIRCLE('',#34754,82.9309999999989);
#2536=CIRCLE('',#34756,82.9310000000032);
#2537=CIRCLE('',#34759,82.931);
#2538=CIRCLE('',#34761,82.9309999999999);
#2539=CIRCLE('',#34763,82.931000000047);
#2540=CIRCLE('',#34765,82.9310000000546);
#2541=CIRCLE('',#34768,11.1760000000001);
#2542=CIRCLE('',#34782,11.1760000000001);
#2543=CIRCLE('',#34787,6.39225125407378);
#2544=CIRCLE('',#34788,5.73418625920022);
#2545=CIRCLE('',#34789,6.39225125407387);
#2546=CIRCLE('',#34790,6.39225125407349);
#2547=CIRCLE('',#34791,5.73418625919864);
#2548=CIRCLE('',#34792,6.39225125407317);
#2549=CIRCLE('',#34793,6.39225125407526);
#2550=CIRCLE('',#34794,5.73418625919519);
#2551=CIRCLE('',#34795,6.39225125407178);
#2552=CIRCLE('',#34796,6.39225125407384);
#2553=CIRCLE('',#34809,90.932);
#2554=CIRCLE('',#34810,82.931);
#2555=CIRCLE('',#34812,4.12750000000046);
#2556=CIRCLE('',#34813,4.12750000000046);
#2557=CIRCLE('',#34815,0.0083587400462651);
#2558=CIRCLE('',#34816,0.0083587400462651);
#2559=CIRCLE('',#34818,4.1275);
#2560=CIRCLE('',#34819,4.1275);
#2561=CIRCLE('',#34821,0.00835874004620744);
#2562=CIRCLE('',#34822,0.00835874004620744);
#2563=CIRCLE('',#34824,4.12750000000005);
#2564=CIRCLE('',#34825,7.13809812492437);
#2565=CIRCLE('',#34827,0.00835888222172394);
#2566=CIRCLE('',#34828,0.00835888222172394);
#2567=CIRCLE('',#34829,7.13809812641026);
#2568=CIRCLE('',#34830,7.13809812562023);
#2569=CIRCLE('',#34832,90.932);
#2570=CIRCLE('',#34833,90.932);
#2571=CIRCLE('',#34834,19.0499999999999);
#2572=CIRCLE('',#34835,71.882);
#2573=CIRCLE('',#34839,12.446);
#2574=CIRCLE('',#34841,82.931);
#2575=CIRCLE('',#34842,82.931);
#2576=CIRCLE('',#34844,5.64270291970328);
#2577=CIRCLE('',#34847,5.47861854669138);
#2578=CIRCLE('',#34851,5.08000000000016);
#2579=CIRCLE('',#34852,5.08000000000016);
#2580=CIRCLE('',#34853,4.7371);
#2581=CIRCLE('',#34854,2.76860000000045);
#2582=CIRCLE('',#34856,5.08000000000016);
#2583=CIRCLE('',#34859,5.08000000000016);
#2584=CIRCLE('',#34862,5.08);
#2585=CIRCLE('',#34863,5.08);
#2586=CIRCLE('',#34864,4.73709999999994);
#2587=CIRCLE('',#34865,2.7686);
#2588=CIRCLE('',#34867,5.08);
#2589=CIRCLE('',#34870,5.08);
#2590=CIRCLE('',#34873,3.90271);
#2591=CIRCLE('',#34875,3.90271);
#2592=CIRCLE('',#34876,3.90271);
#2593=CIRCLE('',#34878,4.7625);
#2594=CIRCLE('',#34880,3.90271);
#2595=CIRCLE('',#34882,3.90271);
#2596=CIRCLE('',#34883,3.90271);
#2597=CIRCLE('',#34885,4.7625);
#2598=CIRCLE('',#34887,3.90271000000005);
#2599=CIRCLE('',#34889,3.90271000000005);
#2600=CIRCLE('',#34890,3.90271000000005);
#2601=CIRCLE('',#34892,4.7625);
#2602=CIRCLE('',#34894,3.90271);
#2603=CIRCLE('',#34896,3.90271);
#2604=CIRCLE('',#34897,3.90271);
#2605=CIRCLE('',#34899,4.7625);
#2606=CIRCLE('',#34901,82.2083254018421);
#2607=CIRCLE('',#34903,8.76300000000001);
#2608=CIRCLE('',#34904,8.76300000000001);
#2609=CIRCLE('',#34905,8.76300000000001);
#2610=CIRCLE('',#34906,8.76299999999998);
#2611=CIRCLE('',#34907,57.15);
#2612=CIRCLE('',#34909,57.15);
#2613=CIRCLE('',#34911,52.451);
#2614=CIRCLE('',#34913,52.451);
#2615=CIRCLE('',#34915,13.081);
#2616=CIRCLE('',#34917,13.081);
#2617=CIRCLE('',#34919,12.446);
#2618=CIRCLE('',#34922,8.76300000000001);
#2619=CIRCLE('',#34923,2.794);
#2620=CIRCLE('',#34926,2.794);
#2621=CIRCLE('',#34929,8.76299999999998);
#2622=CIRCLE('',#34931,2.794);
#2623=CIRCLE('',#34933,2.794);
#2624=CIRCLE('',#34936,2.79400000000001);
#2625=CIRCLE('',#34938,2.79400000000001);
#2626=CIRCLE('',#34940,8.76300000000001);
#2627=CIRCLE('',#34943,8.76300000000001);
#2628=CIRCLE('',#34945,2.794);
#2629=CIRCLE('',#34947,2.794);
#2630=CIRCLE('',#34951,2.76860000000046);
#2631=CIRCLE('',#34952,2.76860000000045);
#2632=CIRCLE('',#34955,2.7686);
#2633=CIRCLE('',#34956,2.7686);
#2634=CIRCLE('',#34957,2.18440000000005);
#2635=CIRCLE('',#34959,2.7686);
#2636=CIRCLE('',#34962,2.76860000000046);
#2637=CIRCLE('',#34964,2.1844);
#2638=CIRCLE('',#34966,4.73709999999989);
#2639=CIRCLE('',#34967,4.73709999999993);
#2640=CIRCLE('',#34969,2.1844);
#2641=CIRCLE('',#34972,4.9247349817135);
#2642=CIRCLE('',#34973,5.64270291970351);
#2643=CIRCLE('',#34974,5.47861854669129);
#2644=CIRCLE('',#34975,5.64270291970121);
#2645=CIRCLE('',#34976,4.92473498170593);
#2646=CIRCLE('',#34977,5.64270291970139);
#2647=CIRCLE('',#34978,5.47861854669133);
#2648=CIRCLE('',#34979,5.64270291970326);
#2649=CIRCLE('',#34980,4.92473498170479);
#2650=CIRCLE('',#34981,5.64270291970299);
#2651=CIRCLE('',#34982,4.92473498170593);
#2652=CIRCLE('',#34983,5.64270291970284);
#2653=CIRCLE('',#34984,5.47861854669129);
#2654=CIRCLE('',#34985,5.64270291970352);
#2655=CIRCLE('',#34987,4.73710000000003);
#2656=CIRCLE('',#34988,2.1844);
#2657=CIRCLE('',#34991,4.73710000000006);
#2658=CIRCLE('',#34993,4.92473498170677);
#2659=CIRCLE('',#34994,5.64270291970129);
#2660=CIRCLE('',#34995,5.47861854668747);
#2661=CIRCLE('',#34996,5.64270291969926);
#2662=CIRCLE('',#34997,4.9247349817059);
#2663=CIRCLE('',#34998,5.64270291970433);
#2664=CIRCLE('',#34999,5.47861854667958);
#2665=CIRCLE('',#35000,5.64270291970706);
#2666=CIRCLE('',#35001,4.92473498170641);
#2667=CIRCLE('',#35002,5.64270291970507);
#2668=CIRCLE('',#35003,5.47861854667962);
#2669=CIRCLE('',#35004,5.64270291970448);
#2670=CIRCLE('',#35005,4.9247349817059);
#2671=CIRCLE('',#35006,5.64270291970619);
#2672=CIRCLE('',#35007,5.47861854669134);
#2673=CIRCLE('',#35008,5.64270291969768);
#4479=FACE_OUTER_BOUND('',#6402,.T.);
#4480=FACE_OUTER_BOUND('',#6403,.T.);
#4481=FACE_OUTER_BOUND('',#6404,.T.);
#4482=FACE_OUTER_BOUND('',#6405,.T.);
#4483=FACE_OUTER_BOUND('',#6406,.T.);
#4484=FACE_OUTER_BOUND('',#6407,.T.);
#4485=FACE_OUTER_BOUND('',#6408,.T.);
#4486=FACE_OUTER_BOUND('',#6411,.T.);
#4487=FACE_OUTER_BOUND('',#6412,.T.);
#4488=FACE_OUTER_BOUND('',#6413,.T.);
#4489=FACE_OUTER_BOUND('',#6414,.T.);
#4490=FACE_OUTER_BOUND('',#6415,.T.);
#4491=FACE_OUTER_BOUND('',#6416,.T.);
#4492=FACE_OUTER_BOUND('',#6417,.T.);
#4493=FACE_OUTER_BOUND('',#6420,.T.);
#4494=FACE_OUTER_BOUND('',#6421,.T.);
#4495=FACE_OUTER_BOUND('',#6423,.T.);
#4496=FACE_OUTER_BOUND('',#6424,.T.);
#4497=FACE_OUTER_BOUND('',#6425,.T.);
#4498=FACE_OUTER_BOUND('',#6426,.T.);
#4499=FACE_OUTER_BOUND('',#6427,.T.);
#4500=FACE_OUTER_BOUND('',#6428,.T.);
#4501=FACE_OUTER_BOUND('',#6429,.T.);
#4502=FACE_OUTER_BOUND('',#6430,.T.);
#4503=FACE_OUTER_BOUND('',#6431,.T.);
#4504=FACE_OUTER_BOUND('',#6432,.T.);
#4505=FACE_OUTER_BOUND('',#6433,.T.);
#4506=FACE_OUTER_BOUND('',#6434,.T.);
#4507=FACE_OUTER_BOUND('',#6435,.T.);
#4508=FACE_OUTER_BOUND('',#6436,.T.);
#4509=FACE_OUTER_BOUND('',#6437,.T.);
#4510=FACE_OUTER_BOUND('',#6438,.T.);
#4511=FACE_OUTER_BOUND('',#6439,.T.);
#4512=FACE_OUTER_BOUND('',#6440,.T.);
#4513=FACE_OUTER_BOUND('',#6441,.T.);
#4514=FACE_OUTER_BOUND('',#6443,.T.);
#4515=FACE_OUTER_BOUND('',#6444,.T.);
#4516=FACE_OUTER_BOUND('',#6445,.T.);
#4517=FACE_OUTER_BOUND('',#6446,.T.);
#4518=FACE_OUTER_BOUND('',#6447,.T.);
#4519=FACE_OUTER_BOUND('',#6448,.T.);
#4520=FACE_OUTER_BOUND('',#6449,.T.);
#4521=FACE_OUTER_BOUND('',#6450,.T.);
#4522=FACE_OUTER_BOUND('',#6451,.T.);
#4523=FACE_OUTER_BOUND('',#6452,.T.);
#4524=FACE_OUTER_BOUND('',#6453,.T.);
#4525=FACE_OUTER_BOUND('',#6455,.T.);
#4526=FACE_OUTER_BOUND('',#6459,.T.);
#4527=FACE_OUTER_BOUND('',#6460,.T.);
#4528=FACE_OUTER_BOUND('',#6461,.T.);
#4529=FACE_OUTER_BOUND('',#6462,.T.);
#4530=FACE_OUTER_BOUND('',#6463,.T.);
#4531=FACE_OUTER_BOUND('',#6464,.T.);
#4532=FACE_OUTER_BOUND('',#6465,.T.);
#4533=FACE_OUTER_BOUND('',#6466,.T.);
#4534=FACE_OUTER_BOUND('',#6467,.T.);
#4535=FACE_OUTER_BOUND('',#6468,.T.);
#4536=FACE_OUTER_BOUND('',#6470,.T.);
#4537=FACE_OUTER_BOUND('',#6471,.T.);
#4538=FACE_OUTER_BOUND('',#6473,.T.);
#4539=FACE_OUTER_BOUND('',#6474,.T.);
#4540=FACE_OUTER_BOUND('',#6475,.T.);
#4541=FACE_OUTER_BOUND('',#6476,.T.);
#4542=FACE_OUTER_BOUND('',#6477,.T.);
#4543=FACE_OUTER_BOUND('',#6478,.T.);
#4544=FACE_OUTER_BOUND('',#6479,.T.);
#4545=FACE_OUTER_BOUND('',#6480,.T.);
#4546=FACE_OUTER_BOUND('',#6481,.T.);
#4547=FACE_OUTER_BOUND('',#6482,.T.);
#4548=FACE_OUTER_BOUND('',#6483,.T.);
#4549=FACE_OUTER_BOUND('',#6484,.T.);
#4550=FACE_OUTER_BOUND('',#6485,.T.);
#4551=FACE_OUTER_BOUND('',#6486,.T.);
#4552=FACE_OUTER_BOUND('',#6487,.T.);
#4553=FACE_OUTER_BOUND('',#6488,.T.);
#4554=FACE_OUTER_BOUND('',#6489,.T.);
#4555=FACE_OUTER_BOUND('',#6490,.T.);
#4556=FACE_OUTER_BOUND('',#6491,.T.);
#4557=FACE_OUTER_BOUND('',#6492,.T.);
#4558=FACE_OUTER_BOUND('',#6493,.T.);
#4559=FACE_OUTER_BOUND('',#6494,.T.);
#4560=FACE_OUTER_BOUND('',#6495,.T.);
#4561=FACE_OUTER_BOUND('',#6496,.T.);
#4562=FACE_OUTER_BOUND('',#6497,.T.);
#4563=FACE_OUTER_BOUND('',#6498,.T.);
#4564=FACE_OUTER_BOUND('',#6499,.T.);
#4565=FACE_OUTER_BOUND('',#6500,.T.);
#4566=FACE_OUTER_BOUND('',#6501,.T.);
#4567=FACE_OUTER_BOUND('',#6502,.T.);
#4568=FACE_OUTER_BOUND('',#6503,.T.);
#4569=FACE_OUTER_BOUND('',#6504,.T.);
#4570=FACE_OUTER_BOUND('',#6505,.T.);
#4571=FACE_OUTER_BOUND('',#6506,.T.);
#4572=FACE_OUTER_BOUND('',#6507,.T.);
#4573=FACE_OUTER_BOUND('',#6508,.T.);
#4574=FACE_OUTER_BOUND('',#6509,.T.);
#4575=FACE_OUTER_BOUND('',#6510,.T.);
#4576=FACE_OUTER_BOUND('',#6511,.T.);
#4577=FACE_OUTER_BOUND('',#6512,.T.);
#4578=FACE_OUTER_BOUND('',#6513,.T.);
#4579=FACE_OUTER_BOUND('',#6514,.T.);
#4580=FACE_OUTER_BOUND('',#6515,.T.);
#4581=FACE_OUTER_BOUND('',#6516,.T.);
#4582=FACE_OUTER_BOUND('',#6517,.T.);
#4583=FACE_OUTER_BOUND('',#6518,.T.);
#4584=FACE_OUTER_BOUND('',#6519,.T.);
#4585=FACE_OUTER_BOUND('',#6520,.T.);
#4586=FACE_OUTER_BOUND('',#6522,.T.);
#4587=FACE_OUTER_BOUND('',#6523,.T.);
#4588=FACE_OUTER_BOUND('',#6524,.T.);
#4589=FACE_OUTER_BOUND('',#6525,.T.);
#4590=FACE_OUTER_BOUND('',#6526,.T.);
#4591=FACE_OUTER_BOUND('',#6527,.T.);
#4592=FACE_OUTER_BOUND('',#6528,.T.);
#4593=FACE_OUTER_BOUND('',#6529,.T.);
#4594=FACE_OUTER_BOUND('',#6530,.T.);
#4595=FACE_OUTER_BOUND('',#6531,.T.);
#4596=FACE_OUTER_BOUND('',#6532,.T.);
#4597=FACE_OUTER_BOUND('',#6533,.T.);
#4598=FACE_OUTER_BOUND('',#6534,.T.);
#4599=FACE_OUTER_BOUND('',#6535,.T.);
#4600=FACE_OUTER_BOUND('',#6536,.T.);
#4601=FACE_OUTER_BOUND('',#6537,.T.);
#4602=FACE_OUTER_BOUND('',#6538,.T.);
#4603=FACE_OUTER_BOUND('',#6540,.T.);
#4604=FACE_OUTER_BOUND('',#6541,.T.);
#4605=FACE_OUTER_BOUND('',#6542,.T.);
#4606=FACE_OUTER_BOUND('',#6543,.T.);
#4607=FACE_OUTER_BOUND('',#6544,.T.);
#4608=FACE_OUTER_BOUND('',#6545,.T.);
#4609=FACE_OUTER_BOUND('',#6546,.T.);
#4610=FACE_OUTER_BOUND('',#6547,.T.);
#4611=FACE_OUTER_BOUND('',#6548,.T.);
#4612=FACE_OUTER_BOUND('',#6549,.T.);
#4613=FACE_OUTER_BOUND('',#6550,.T.);
#4614=FACE_OUTER_BOUND('',#6551,.T.);
#4615=FACE_OUTER_BOUND('',#6553,.T.);
#4616=FACE_OUTER_BOUND('',#6554,.T.);
#4617=FACE_OUTER_BOUND('',#6555,.T.);
#4618=FACE_OUTER_BOUND('',#6556,.T.);
#4619=FACE_OUTER_BOUND('',#6557,.T.);
#4620=FACE_OUTER_BOUND('',#6558,.T.);
#4621=FACE_OUTER_BOUND('',#6559,.T.);
#4622=FACE_OUTER_BOUND('',#6560,.T.);
#4623=FACE_OUTER_BOUND('',#6561,.T.);
#4624=FACE_OUTER_BOUND('',#6562,.T.);
#4625=FACE_OUTER_BOUND('',#6563,.T.);
#4626=FACE_OUTER_BOUND('',#6567,.T.);
#4627=FACE_OUTER_BOUND('',#6568,.T.);
#4628=FACE_OUTER_BOUND('',#6569,.T.);
#4629=FACE_OUTER_BOUND('',#6571,.T.);
#4630=FACE_OUTER_BOUND('',#6572,.T.);
#4631=FACE_OUTER_BOUND('',#6573,.T.);
#4632=FACE_OUTER_BOUND('',#6574,.T.);
#4633=FACE_OUTER_BOUND('',#6575,.T.);
#4634=FACE_OUTER_BOUND('',#6576,.T.);
#4635=FACE_OUTER_BOUND('',#6578,.T.);
#4636=FACE_OUTER_BOUND('',#6579,.T.);
#4637=FACE_OUTER_BOUND('',#6580,.T.);
#4638=FACE_OUTER_BOUND('',#6581,.T.);
#4639=FACE_OUTER_BOUND('',#6582,.T.);
#4640=FACE_OUTER_BOUND('',#6584,.T.);
#4641=FACE_OUTER_BOUND('',#6585,.T.);
#4642=FACE_OUTER_BOUND('',#6586,.T.);
#4643=FACE_OUTER_BOUND('',#6587,.T.);
#4644=FACE_OUTER_BOUND('',#6588,.T.);
#4645=FACE_OUTER_BOUND('',#6589,.T.);
#4646=FACE_OUTER_BOUND('',#6590,.T.);
#4647=FACE_OUTER_BOUND('',#6591,.T.);
#4648=FACE_OUTER_BOUND('',#6592,.T.);
#4649=FACE_OUTER_BOUND('',#6593,.T.);
#4650=FACE_OUTER_BOUND('',#6594,.T.);
#4651=FACE_OUTER_BOUND('',#6595,.T.);
#4652=FACE_OUTER_BOUND('',#6596,.T.);
#4653=FACE_OUTER_BOUND('',#6597,.T.);
#4654=FACE_OUTER_BOUND('',#6598,.T.);
#4655=FACE_OUTER_BOUND('',#6599,.T.);
#4656=FACE_OUTER_BOUND('',#6600,.T.);
#4657=FACE_OUTER_BOUND('',#6601,.T.);
#4658=FACE_OUTER_BOUND('',#6611,.T.);
#4659=FACE_OUTER_BOUND('',#6612,.T.);
#4660=FACE_OUTER_BOUND('',#6614,.T.);
#4661=FACE_OUTER_BOUND('',#6615,.T.);
#4662=FACE_OUTER_BOUND('',#6619,.T.);
#4663=FACE_OUTER_BOUND('',#6620,.T.);
#4664=FACE_OUTER_BOUND('',#6622,.T.);
#4665=FACE_OUTER_BOUND('',#6623,.T.);
#4666=FACE_OUTER_BOUND('',#6625,.T.);
#4667=FACE_OUTER_BOUND('',#6626,.T.);
#4668=FACE_OUTER_BOUND('',#6627,.T.);
#4669=FACE_OUTER_BOUND('',#6628,.T.);
#4670=FACE_OUTER_BOUND('',#6629,.T.);
#4671=FACE_OUTER_BOUND('',#6631,.T.);
#4672=FACE_OUTER_BOUND('',#6632,.T.);
#4673=FACE_OUTER_BOUND('',#6633,.T.);
#4674=FACE_OUTER_BOUND('',#6634,.T.);
#4675=FACE_OUTER_BOUND('',#6635,.T.);
#4676=FACE_OUTER_BOUND('',#6637,.T.);
#4677=FACE_OUTER_BOUND('',#6638,.T.);
#4678=FACE_OUTER_BOUND('',#6639,.T.);
#4679=FACE_OUTER_BOUND('',#6641,.T.);
#4680=FACE_OUTER_BOUND('',#6642,.T.);
#4681=FACE_OUTER_BOUND('',#6643,.T.);
#4682=FACE_OUTER_BOUND('',#6644,.T.);
#4683=FACE_OUTER_BOUND('',#6645,.T.);
#4684=FACE_OUTER_BOUND('',#6646,.T.);
#4685=FACE_OUTER_BOUND('',#6648,.T.);
#4686=FACE_OUTER_BOUND('',#6649,.T.);
#4687=FACE_OUTER_BOUND('',#6650,.T.);
#4688=FACE_OUTER_BOUND('',#6651,.T.);
#4689=FACE_OUTER_BOUND('',#6653,.T.);
#4690=FACE_OUTER_BOUND('',#6654,.T.);
#4691=FACE_OUTER_BOUND('',#6655,.T.);
#4692=FACE_OUTER_BOUND('',#6657,.T.);
#4693=FACE_OUTER_BOUND('',#6659,.T.);
#4694=FACE_OUTER_BOUND('',#6661,.T.);
#4695=FACE_OUTER_BOUND('',#6662,.T.);
#4696=FACE_OUTER_BOUND('',#6663,.T.);
#4697=FACE_OUTER_BOUND('',#6665,.T.);
#4698=FACE_OUTER_BOUND('',#6666,.T.);
#4699=FACE_OUTER_BOUND('',#6667,.T.);
#4700=FACE_OUTER_BOUND('',#6668,.T.);
#4701=FACE_OUTER_BOUND('',#6669,.T.);
#4702=FACE_OUTER_BOUND('',#6670,.T.);
#4703=FACE_OUTER_BOUND('',#6671,.T.);
#4704=FACE_OUTER_BOUND('',#6672,.T.);
#4705=FACE_OUTER_BOUND('',#6673,.T.);
#4706=FACE_OUTER_BOUND('',#6674,.T.);
#4707=FACE_OUTER_BOUND('',#6675,.T.);
#4708=FACE_OUTER_BOUND('',#6676,.T.);
#4709=FACE_OUTER_BOUND('',#6677,.T.);
#4710=FACE_OUTER_BOUND('',#6678,.T.);
#4711=FACE_OUTER_BOUND('',#6679,.T.);
#4712=FACE_OUTER_BOUND('',#6680,.T.);
#4713=FACE_OUTER_BOUND('',#6681,.T.);
#4714=FACE_OUTER_BOUND('',#6682,.T.);
#4715=FACE_OUTER_BOUND('',#6683,.T.);
#4716=FACE_OUTER_BOUND('',#6684,.T.);
#4717=FACE_OUTER_BOUND('',#6685,.T.);
#4718=FACE_OUTER_BOUND('',#6686,.T.);
#4719=FACE_OUTER_BOUND('',#6687,.T.);
#4720=FACE_OUTER_BOUND('',#6688,.T.);
#4721=FACE_OUTER_BOUND('',#6689,.T.);
#4722=FACE_OUTER_BOUND('',#6690,.T.);
#4723=FACE_OUTER_BOUND('',#6691,.T.);
#4724=FACE_OUTER_BOUND('',#6692,.T.);
#4725=FACE_OUTER_BOUND('',#6693,.T.);
#4726=FACE_OUTER_BOUND('',#6694,.T.);
#4727=FACE_OUTER_BOUND('',#6695,.T.);
#6402=EDGE_LOOP('',(#22598,#22599,#22600,#22601,#22602,#22603,#22604,#22605,
#22606,#22607,#22608,#22609,#22610,#22611,#22612,#22613,#22614));
#6403=EDGE_LOOP('',(#22615,#22616,#22617,#22618));
#6404=EDGE_LOOP('',(#22619,#22620,#22621,#22622));
#6405=EDGE_LOOP('',(#22623,#22624,#22625,#22626));
#6406=EDGE_LOOP('',(#22627,#22628));
#6407=EDGE_LOOP('',(#22629,#22630,#22631,#22632,#22633,#22634,#22635));
#6408=EDGE_LOOP('',(#22636,#22637,#22638,#22639,#22640,#22641,#22642,#22643,
#22644,#22645));
#6409=EDGE_LOOP('',(#22646,#22647,#22648));
#6410=EDGE_LOOP('',(#22649,#22650,#22651));
#6411=EDGE_LOOP('',(#22652,#22653,#22654,#22655));
#6412=EDGE_LOOP('',(#22656,#22657,#22658,#22659));
#6413=EDGE_LOOP('',(#22660,#22661,#22662,#22663));
#6414=EDGE_LOOP('',(#22664,#22665,#22666,#22667));
#6415=EDGE_LOOP('',(#22668,#22669,#22670,#22671));
#6416=EDGE_LOOP('',(#22672,#22673,#22674,#22675,#22676,#22677));
#6417=EDGE_LOOP('',(#22678,#22679,#22680,#22681,#22682,#22683,#22684,#22685,
#22686,#22687));
#6418=EDGE_LOOP('',(#22688,#22689,#22690));
#6419=EDGE_LOOP('',(#22691,#22692,#22693));
#6420=EDGE_LOOP('',(#22694,#22695));
#6421=EDGE_LOOP('',(#22696));
#6422=EDGE_LOOP('',(#22697,#22698,#22699,#22700,#22701,#22702,#22703,#22704,
#22705,#22706,#22707,#22708));
#6423=EDGE_LOOP('',(#22709,#22710,#22711,#22712));
#6424=EDGE_LOOP('',(#22713,#22714,#22715,#22716));
#6425=EDGE_LOOP('',(#22717,#22718));
#6426=EDGE_LOOP('',(#22719,#22720,#22721,#22722,#22723,#22724));
#6427=EDGE_LOOP('',(#22725,#22726,#22727,#22728,#22729,#22730));
#6428=EDGE_LOOP('',(#22731,#22732,#22733,#22734));
#6429=EDGE_LOOP('',(#22735,#22736,#22737,#22738));
#6430=EDGE_LOOP('',(#22739,#22740,#22741,#22742));
#6431=EDGE_LOOP('',(#22743,#22744,#22745,#22746));
#6432=EDGE_LOOP('',(#22747,#22748,#22749,#22750));
#6433=EDGE_LOOP('',(#22751,#22752,#22753,#22754));
#6434=EDGE_LOOP('',(#22755,#22756,#22757,#22758));
#6435=EDGE_LOOP('',(#22759,#22760,#22761,#22762));
#6436=EDGE_LOOP('',(#22763,#22764,#22765,#22766));
#6437=EDGE_LOOP('',(#22767,#22768,#22769,#22770));
#6438=EDGE_LOOP('',(#22771,#22772,#22773,#22774));
#6439=EDGE_LOOP('',(#22775,#22776,#22777,#22778));
#6440=EDGE_LOOP('',(#22779,#22780,#22781,#22782,#22783,#22784,#22785,#22786,
#22787,#22788,#22789,#22790));
#6441=EDGE_LOOP('',(#22791));
#6442=EDGE_LOOP('',(#22792,#22793,#22794,#22795,#22796,#22797,#22798,#22799,
#22800,#22801,#22802,#22803));
#6443=EDGE_LOOP('',(#22804,#22805));
#6444=EDGE_LOOP('',(#22806,#22807,#22808,#22809));
#6445=EDGE_LOOP('',(#22810,#22811,#22812,#22813));
#6446=EDGE_LOOP('',(#22814,#22815,#22816,#22817));
#6447=EDGE_LOOP('',(#22818,#22819,#22820,#22821));
#6448=EDGE_LOOP('',(#22822,#22823,#22824,#22825));
#6449=EDGE_LOOP('',(#22826,#22827,#22828,#22829));
#6450=EDGE_LOOP('',(#22830,#22831,#22832,#22833));
#6451=EDGE_LOOP('',(#22834,#22835,#22836,#22837));
#6452=EDGE_LOOP('',(#22838,#22839,#22840,#22841));
#6453=EDGE_LOOP('',(#22842,#22843,#22844,#22845,#22846,#22847,#22848,#22849));
#6454=EDGE_LOOP('',(#22850,#22851,#22852,#22853));
#6455=EDGE_LOOP('',(#22854,#22855,#22856,#22857,#22858,#22859,#22860,#22861));
#6456=EDGE_LOOP('',(#22862));
#6457=EDGE_LOOP('',(#22863));
#6458=EDGE_LOOP('',(#22864,#22865,#22866,#22867,#22868,#22869,#22870,#22871));
#6459=EDGE_LOOP('',(#22872,#22873,#22874,#22875));
#6460=EDGE_LOOP('',(#22876,#22877,#22878,#22879));
#6461=EDGE_LOOP('',(#22880,#22881,#22882,#22883));
#6462=EDGE_LOOP('',(#22884,#22885,#22886,#22887));
#6463=EDGE_LOOP('',(#22888,#22889,#22890,#22891));
#6464=EDGE_LOOP('',(#22892,#22893,#22894,#22895));
#6465=EDGE_LOOP('',(#22896,#22897,#22898,#22899));
#6466=EDGE_LOOP('',(#22900,#22901,#22902,#22903));
#6467=EDGE_LOOP('',(#22904,#22905,#22906,#22907,#22908,#22909,#22910,#22911));
#6468=EDGE_LOOP('',(#22912));
#6469=EDGE_LOOP('',(#22913,#22914,#22915,#22916,#22917,#22918,#22919,#22920,
#22921,#22922,#22923,#22924));
#6470=EDGE_LOOP('',(#22925,#22926,#22927,#22928));
#6471=EDGE_LOOP('',(#22929));
#6472=EDGE_LOOP('',(#22930,#22931,#22932,#22933,#22934,#22935,#22936,#22937,
#22938,#22939,#22940,#22941));
#6473=EDGE_LOOP('',(#22942,#22943,#22944,#22945));
#6474=EDGE_LOOP('',(#22946,#22947,#22948,#22949));
#6475=EDGE_LOOP('',(#22950,#22951,#22952,#22953));
#6476=EDGE_LOOP('',(#22954,#22955,#22956,#22957));
#6477=EDGE_LOOP('',(#22958,#22959,#22960,#22961));
#6478=EDGE_LOOP('',(#22962,#22963,#22964,#22965));
#6479=EDGE_LOOP('',(#22966,#22967,#22968,#22969));
#6480=EDGE_LOOP('',(#22970,#22971,#22972,#22973));
#6481=EDGE_LOOP('',(#22974,#22975,#22976,#22977));
#6482=EDGE_LOOP('',(#22978,#22979,#22980,#22981));
#6483=EDGE_LOOP('',(#22982,#22983,#22984,#22985));
#6484=EDGE_LOOP('',(#22986,#22987,#22988,#22989));
#6485=EDGE_LOOP('',(#22990,#22991,#22992,#22993));
#6486=EDGE_LOOP('',(#22994,#22995,#22996,#22997,#22998,#22999,#23000,#23001,
#23002,#23003,#23004,#23005));
#6487=EDGE_LOOP('',(#23006,#23007,#23008,#23009));
#6488=EDGE_LOOP('',(#23010,#23011,#23012,#23013));
#6489=EDGE_LOOP('',(#23014,#23015,#23016,#23017));
#6490=EDGE_LOOP('',(#23018,#23019,#23020,#23021));
#6491=EDGE_LOOP('',(#23022,#23023,#23024,#23025));
#6492=EDGE_LOOP('',(#23026,#23027,#23028,#23029));
#6493=EDGE_LOOP('',(#23030,#23031,#23032,#23033));
#6494=EDGE_LOOP('',(#23034,#23035,#23036,#23037));
#6495=EDGE_LOOP('',(#23038,#23039,#23040,#23041));
#6496=EDGE_LOOP('',(#23042,#23043,#23044,#23045));
#6497=EDGE_LOOP('',(#23046,#23047,#23048,#23049));
#6498=EDGE_LOOP('',(#23050,#23051,#23052,#23053));
#6499=EDGE_LOOP('',(#23054,#23055,#23056,#23057,#23058,#23059,#23060,#23061,
#23062,#23063,#23064,#23065));
#6500=EDGE_LOOP('',(#23066,#23067,#23068,#23069,#23070,#23071,#23072,#23073,
#23074,#23075,#23076,#23077));
#6501=EDGE_LOOP('',(#23078,#23079,#23080,#23081));
#6502=EDGE_LOOP('',(#23082,#23083,#23084,#23085));
#6503=EDGE_LOOP('',(#23086,#23087,#23088,#23089));
#6504=EDGE_LOOP('',(#23090,#23091,#23092,#23093));
#6505=EDGE_LOOP('',(#23094,#23095,#23096,#23097));
#6506=EDGE_LOOP('',(#23098,#23099,#23100,#23101));
#6507=EDGE_LOOP('',(#23102,#23103,#23104,#23105));
#6508=EDGE_LOOP('',(#23106,#23107,#23108,#23109,#23110));
#6509=EDGE_LOOP('',(#23111,#23112,#23113,#23114));
#6510=EDGE_LOOP('',(#23115,#23116,#23117,#23118));
#6511=EDGE_LOOP('',(#23119,#23120,#23121,#23122));
#6512=EDGE_LOOP('',(#23123,#23124,#23125,#23126));
#6513=EDGE_LOOP('',(#23127,#23128,#23129,#23130));
#6514=EDGE_LOOP('',(#23131,#23132,#23133,#23134));
#6515=EDGE_LOOP('',(#23135,#23136,#23137,#23138,#23139,#23140,#23141,#23142));
#6516=EDGE_LOOP('',(#23143,#23144,#23145,#23146,#23147,#23148,#23149,#23150));
#6517=EDGE_LOOP('',(#23151,#23152,#23153,#23154));
#6518=EDGE_LOOP('',(#23155,#23156,#23157,#23158));
#6519=EDGE_LOOP('',(#23159,#23160,#23161,#23162));
#6520=EDGE_LOOP('',(#23163,#23164,#23165,#23166));
#6521=EDGE_LOOP('',(#23167));
#6522=EDGE_LOOP('',(#23168,#23169,#23170,#23171));
#6523=EDGE_LOOP('',(#23172,#23173,#23174,#23175));
#6524=EDGE_LOOP('',(#23176,#23177,#23178,#23179));
#6525=EDGE_LOOP('',(#23180,#23181,#23182,#23183));
#6526=EDGE_LOOP('',(#23184,#23185,#23186,#23187));
#6527=EDGE_LOOP('',(#23188,#23189,#23190,#23191));
#6528=EDGE_LOOP('',(#23192,#23193,#23194,#23195));
#6529=EDGE_LOOP('',(#23196,#23197,#23198,#23199));
#6530=EDGE_LOOP('',(#23200,#23201,#23202,#23203));
#6531=EDGE_LOOP('',(#23204,#23205,#23206,#23207));
#6532=EDGE_LOOP('',(#23208,#23209,#23210,#23211));
#6533=EDGE_LOOP('',(#23212,#23213,#23214,#23215));
#6534=EDGE_LOOP('',(#23216,#23217,#23218,#23219));
#6535=EDGE_LOOP('',(#23220));
#6536=EDGE_LOOP('',(#23221,#23222,#23223,#23224,#23225,#23226,#23227,#23228,
#23229,#23230,#23231,#23232));
#6537=EDGE_LOOP('',(#23233,#23234,#23235,#23236));
#6538=EDGE_LOOP('',(#23237));
#6539=EDGE_LOOP('',(#23238,#23239,#23240,#23241,#23242,#23243,#23244,#23245,
#23246,#23247,#23248,#23249));
#6540=EDGE_LOOP('',(#23250,#23251,#23252,#23253,#23254,#23255,#23256,#23257,
#23258,#23259,#23260,#23261));
#6541=EDGE_LOOP('',(#23262,#23263,#23264,#23265));
#6542=EDGE_LOOP('',(#23266,#23267,#23268,#23269));
#6543=EDGE_LOOP('',(#23270,#23271,#23272,#23273));
#6544=EDGE_LOOP('',(#23274,#23275,#23276,#23277));
#6545=EDGE_LOOP('',(#23278,#23279,#23280,#23281));
#6546=EDGE_LOOP('',(#23282,#23283,#23284,#23285));
#6547=EDGE_LOOP('',(#23286,#23287,#23288,#23289));
#6548=EDGE_LOOP('',(#23290,#23291,#23292,#23293));
#6549=EDGE_LOOP('',(#23294,#23295,#23296,#23297));
#6550=EDGE_LOOP('',(#23298,#23299,#23300,#23301));
#6551=EDGE_LOOP('',(#23302));
#6552=EDGE_LOOP('',(#23303));
#6553=EDGE_LOOP('',(#23304,#23305,#23306,#23307,#23308,#23309));
#6554=EDGE_LOOP('',(#23310,#23311));
#6555=EDGE_LOOP('',(#23312,#23313,#23314,#23315,#23316,#23317));
#6556=EDGE_LOOP('',(#23318,#23319,#23320));
#6557=EDGE_LOOP('',(#23321,#23322,#23323,#23324,#23325));
#6558=EDGE_LOOP('',(#23326,#23327,#23328,#23329,#23330,#23331));
#6559=EDGE_LOOP('',(#23332,#23333));
#6560=EDGE_LOOP('',(#23334,#23335,#23336,#23337,#23338,#23339));
#6561=EDGE_LOOP('',(#23340,#23341,#23342,#23343,#23344,#23345));
#6562=EDGE_LOOP('',(#23346,#23347,#23348,#23349,#23350));
#6563=EDGE_LOOP('',(#23351,#23352,#23353,#23354,#23355));
#6564=EDGE_LOOP('',(#23356,#23357));
#6565=EDGE_LOOP('',(#23358,#23359));
#6566=EDGE_LOOP('',(#23360,#23361));
#6567=EDGE_LOOP('',(#23362));
#6568=EDGE_LOOP('',(#23363));
#6569=EDGE_LOOP('',(#23364,#23365,#23366,#23367,#23368));
#6570=EDGE_LOOP('',(#23369,#23370,#23371,#23372,#23373,#23374,#23375,#23376,
#23377,#23378,#23379,#23380,#23381,#23382,#23383,#23384));
#6571=EDGE_LOOP('',(#23385,#23386,#23387,#23388));
#6572=EDGE_LOOP('',(#23389,#23390,#23391,#23392,#23393,#23394,#23395,#23396,
#23397,#23398,#23399,#23400,#23401,#23402,#23403,#23404));
#6573=EDGE_LOOP('',(#23405,#23406,#23407,#23408));
#6574=EDGE_LOOP('',(#23409,#23410,#23411,#23412,#23413,#23414));
#6575=EDGE_LOOP('',(#23415,#23416,#23417,#23418,#23419,#23420));
#6576=EDGE_LOOP('',(#23421,#23422,#23423,#23424));
#6577=EDGE_LOOP('',(#23425,#23426,#23427,#23428));
#6578=EDGE_LOOP('',(#23429,#23430,#23431,#23432));
#6579=EDGE_LOOP('',(#23433,#23434,#23435,#23436));
#6580=EDGE_LOOP('',(#23437,#23438,#23439,#23440));
#6581=EDGE_LOOP('',(#23441,#23442,#23443,#23444));
#6582=EDGE_LOOP('',(#23445,#23446,#23447,#23448));
#6583=EDGE_LOOP('',(#23449,#23450,#23451,#23452));
#6584=EDGE_LOOP('',(#23453,#23454,#23455,#23456));
#6585=EDGE_LOOP('',(#23457,#23458,#23459,#23460));
#6586=EDGE_LOOP('',(#23461,#23462,#23463,#23464));
#6587=EDGE_LOOP('',(#23465,#23466,#23467,#23468));
#6588=EDGE_LOOP('',(#23469));
#6589=EDGE_LOOP('',(#23470,#23471,#23472,#23473,#23474));
#6590=EDGE_LOOP('',(#23475,#23476,#23477,#23478,#23479));
#6591=EDGE_LOOP('',(#23480));
#6592=EDGE_LOOP('',(#23481,#23482,#23483,#23484,#23485));
#6593=EDGE_LOOP('',(#23486,#23487,#23488,#23489,#23490));
#6594=EDGE_LOOP('',(#23491));
#6595=EDGE_LOOP('',(#23492,#23493,#23494,#23495,#23496));
#6596=EDGE_LOOP('',(#23497,#23498,#23499,#23500,#23501));
#6597=EDGE_LOOP('',(#23502));
#6598=EDGE_LOOP('',(#23503,#23504,#23505,#23506,#23507));
#6599=EDGE_LOOP('',(#23508,#23509,#23510,#23511,#23512));
#6600=EDGE_LOOP('',(#23513,#23514,#23515,#23516,#23517));
#6601=EDGE_LOOP('',(#23518));
#6602=EDGE_LOOP('',(#23519));
#6603=EDGE_LOOP('',(#23520));
#6604=EDGE_LOOP('',(#23521));
#6605=EDGE_LOOP('',(#23522));
#6606=EDGE_LOOP('',(#23523));
#6607=EDGE_LOOP('',(#23524));
#6608=EDGE_LOOP('',(#23525));
#6609=EDGE_LOOP('',(#23526));
#6610=EDGE_LOOP('',(#23527));
#6611=EDGE_LOOP('',(#23528,#23529,#23530,#23531));
#6612=EDGE_LOOP('',(#23532));
#6613=EDGE_LOOP('',(#23533));
#6614=EDGE_LOOP('',(#23534,#23535,#23536,#23537));
#6615=EDGE_LOOP('',(#23538));
#6616=EDGE_LOOP('',(#23539,#23540,#23541,#23542));
#6617=EDGE_LOOP('',(#23543,#23544,#23545,#23546));
#6618=EDGE_LOOP('',(#23547));
#6619=EDGE_LOOP('',(#23548,#23549,#23550,#23551));
#6620=EDGE_LOOP('',(#23552));
#6621=EDGE_LOOP('',(#23553));
#6622=EDGE_LOOP('',(#23554,#23555,#23556,#23557));
#6623=EDGE_LOOP('',(#23558));
#6624=EDGE_LOOP('',(#23559));
#6625=EDGE_LOOP('',(#23560,#23561,#23562,#23563));
#6626=EDGE_LOOP('',(#23564,#23565,#23566,#23567));
#6627=EDGE_LOOP('',(#23568));
#6628=EDGE_LOOP('',(#23569,#23570,#23571,#23572));
#6629=EDGE_LOOP('',(#23573));
#6630=EDGE_LOOP('',(#23574));
#6631=EDGE_LOOP('',(#23575,#23576,#23577,#23578));
#6632=EDGE_LOOP('',(#23579));
#6633=EDGE_LOOP('',(#23580));
#6634=EDGE_LOOP('',(#23581,#23582,#23583,#23584));
#6635=EDGE_LOOP('',(#23585));
#6636=EDGE_LOOP('',(#23586));
#6637=EDGE_LOOP('',(#23587,#23588,#23589,#23590));
#6638=EDGE_LOOP('',(#23591,#23592,#23593,#23594));
#6639=EDGE_LOOP('',(#23595));
#6640=EDGE_LOOP('',(#23596));
#6641=EDGE_LOOP('',(#23597,#23598,#23599,#23600));
#6642=EDGE_LOOP('',(#23601));
#6643=EDGE_LOOP('',(#23602,#23603,#23604,#23605,#23606,#23607));
#6644=EDGE_LOOP('',(#23608,#23609,#23610,#23611));
#6645=EDGE_LOOP('',(#23612,#23613,#23614,#23615,#23616,#23617));
#6646=EDGE_LOOP('',(#23618,#23619,#23620,#23621));
#6647=EDGE_LOOP('',(#23622));
#6648=EDGE_LOOP('',(#23623,#23624,#23625,#23626));
#6649=EDGE_LOOP('',(#23627,#23628,#23629,#23630));
#6650=EDGE_LOOP('',(#23631,#23632,#23633,#23634));
#6651=EDGE_LOOP('',(#23635,#23636,#23637,#23638));
#6652=EDGE_LOOP('',(#23639));
#6653=EDGE_LOOP('',(#23640,#23641,#23642,#23643));
#6654=EDGE_LOOP('',(#23644,#23645,#23646,#23647));
#6655=EDGE_LOOP('',(#23648,#23649,#23650,#23651));
#6656=EDGE_LOOP('',(#23652));
#6657=EDGE_LOOP('',(#23653,#23654));
#6658=EDGE_LOOP('',(#23655,#23656,#23657,#23658,#23659,#23660,#23661,#23662,
#23663,#23664,#23665,#23666,#23667,#23668,#23669,#23670));
#6659=EDGE_LOOP('',(#23671,#23672,#23673,#23674));
#6660=EDGE_LOOP('',(#23675));
#6661=EDGE_LOOP('',(#23676,#23677,#23678,#23679));
#6662=EDGE_LOOP('',(#23680,#23681,#23682,#23683));
#6663=EDGE_LOOP('',(#23684,#23685));
#6664=EDGE_LOOP('',(#23686,#23687,#23688,#23689,#23690,#23691,#23692,#23693,
#23694,#23695,#23696,#23697,#23698,#23699,#23700,#23701));
#6665=EDGE_LOOP('',(#23702,#23703,#23704,#23705));
#6666=EDGE_LOOP('',(#23706,#23707,#23708,#23709));
#6667=EDGE_LOOP('',(#23710,#23711,#23712,#23713));
#6668=EDGE_LOOP('',(#23714,#23715,#23716,#23717));
#6669=EDGE_LOOP('',(#23718,#23719,#23720,#23721));
#6670=EDGE_LOOP('',(#23722,#23723,#23724,#23725));
#6671=EDGE_LOOP('',(#23726,#23727,#23728,#23729));
#6672=EDGE_LOOP('',(#23730,#23731,#23732,#23733));
#6673=EDGE_LOOP('',(#23734,#23735,#23736,#23737));
#6674=EDGE_LOOP('',(#23738,#23739,#23740,#23741));
#6675=EDGE_LOOP('',(#23742,#23743,#23744,#23745));
#6676=EDGE_LOOP('',(#23746,#23747,#23748,#23749));
#6677=EDGE_LOOP('',(#23750,#23751,#23752,#23753));
#6678=EDGE_LOOP('',(#23754,#23755,#23756,#23757));
#6679=EDGE_LOOP('',(#23758,#23759,#23760,#23761));
#6680=EDGE_LOOP('',(#23762,#23763,#23764,#23765));
#6681=EDGE_LOOP('',(#23766,#23767,#23768,#23769,#23770,#23771,#23772,#23773,
#23774,#23775,#23776,#23777,#23778,#23779,#23780,#23781));
#6682=EDGE_LOOP('',(#23782,#23783,#23784,#23785));
#6683=EDGE_LOOP('',(#23786,#23787,#23788,#23789));
#6684=EDGE_LOOP('',(#23790,#23791,#23792,#23793));
#6685=EDGE_LOOP('',(#23794,#23795,#23796,#23797));
#6686=EDGE_LOOP('',(#23798,#23799,#23800,#23801));
#6687=EDGE_LOOP('',(#23802,#23803,#23804,#23805));
#6688=EDGE_LOOP('',(#23806,#23807,#23808,#23809));
#6689=EDGE_LOOP('',(#23810,#23811,#23812,#23813));
#6690=EDGE_LOOP('',(#23814,#23815,#23816,#23817));
#6691=EDGE_LOOP('',(#23818,#23819,#23820,#23821));
#6692=EDGE_LOOP('',(#23822,#23823,#23824,#23825));
#6693=EDGE_LOOP('',(#23826,#23827,#23828,#23829));
#6694=EDGE_LOOP('',(#23830,#23831,#23832,#23833));
#6695=EDGE_LOOP('',(#23834,#23835,#23836,#23837));
#8636=LINE('',#51707,#11183);
#8637=LINE('',#51709,#11184);
#8638=LINE('',#51710,#11185);
#8639=LINE('',#51713,#11186);
#8640=LINE('',#51714,#11187);
#8641=LINE('',#51717,#11188);
#8642=LINE('',#51718,#11189);
#8643=LINE('',#51723,#11190);
#8644=LINE('',#51726,#11191);
#8645=LINE('',#51763,#11192);
#8646=LINE('',#51788,#11193);
#8647=LINE('',#51802,#11194);
#8648=LINE('',#51816,#11195);
#8649=LINE('',#51829,#11196);
#8650=LINE('',#51831,#11197);
#8651=LINE('',#51874,#11198);
#8652=LINE('',#51894,#11199);
#8653=LINE('',#51898,#11200);
#8654=LINE('',#51911,#11201);
#8655=LINE('',#51924,#11202);
#8656=LINE('',#51926,#11203);
#8657=LINE('',#51927,#11204);
#8658=LINE('',#51930,#11205);
#8659=LINE('',#51932,#11206);
#8660=LINE('',#51933,#11207);
#8661=LINE('',#51950,#11208);
#8662=LINE('',#51969,#11209);
#8663=LINE('',#51983,#11210);
#8664=LINE('',#51984,#11211);
#8665=LINE('',#51987,#11212);
#8666=LINE('',#52040,#11213);
#8667=LINE('',#52042,#11214);
#8668=LINE('',#52043,#11215);
#8669=LINE('',#52048,#11216);
#8670=LINE('',#52049,#11217);
#8671=LINE('',#52055,#11218);
#8672=LINE('',#52059,#11219);
#8673=LINE('',#52066,#11220);
#8674=LINE('',#52068,#11221);
#8675=LINE('',#52069,#11222);
#8676=LINE('',#52074,#11223);
#8677=LINE('',#52075,#11224);
#8678=LINE('',#52080,#11225);
#8679=LINE('',#52081,#11226);
#8680=LINE('',#52086,#11227);
#8681=LINE('',#52087,#11228);
#8682=LINE('',#52092,#11229);
#8683=LINE('',#52093,#11230);
#8684=LINE('',#52098,#11231);
#8685=LINE('',#52099,#11232);
#8686=LINE('',#52104,#11233);
#8687=LINE('',#52105,#11234);
#8688=LINE('',#52110,#11235);
#8689=LINE('',#52111,#11236);
#8690=LINE('',#52116,#11237);
#8691=LINE('',#52117,#11238);
#8692=LINE('',#52122,#11239);
#8693=LINE('',#52123,#11240);
#8694=LINE('',#52128,#11241);
#8695=LINE('',#52129,#11242);
#8696=LINE('',#52132,#11243);
#8697=LINE('',#52148,#11244);
#8698=LINE('',#52154,#11245);
#8699=LINE('',#52157,#11246);
#8700=LINE('',#52160,#11247);
#8701=LINE('',#52162,#11248);
#8702=LINE('',#52163,#11249);
#8703=LINE('',#52169,#11250);
#8704=LINE('',#52172,#11251);
#8705=LINE('',#52174,#11252);
#8706=LINE('',#52175,#11253);
#8707=LINE('',#52181,#11254);
#8708=LINE('',#52184,#11255);
#8709=LINE('',#52186,#11256);
#8710=LINE('',#52187,#11257);
#8711=LINE('',#52193,#11258);
#8712=LINE('',#52195,#11259);
#8713=LINE('',#52196,#11260);
#8714=LINE('',#52200,#11261);
#8715=LINE('',#52202,#11262);
#8716=LINE('',#52204,#11263);
#8717=LINE('',#52205,#11264);
#8718=LINE('',#52213,#11265);
#8719=LINE('',#52217,#11266);
#8720=LINE('',#52221,#11267);
#8721=LINE('',#52225,#11268);
#8722=LINE('',#52229,#11269);
#8723=LINE('',#52232,#11270);
#8724=LINE('',#52235,#11271);
#8725=LINE('',#52236,#11272);
#8726=LINE('',#52240,#11273);
#8727=LINE('',#52243,#11274);
#8728=LINE('',#52244,#11275);
#8729=LINE('',#52248,#11276);
#8730=LINE('',#52251,#11277);
#8731=LINE('',#52252,#11278);
#8732=LINE('',#52256,#11279);
#8733=LINE('',#52258,#11280);
#8734=LINE('',#52288,#11281);
#8735=LINE('',#52317,#11282);
#8736=LINE('',#52320,#11283);
#8737=LINE('',#52322,#11284);
#8738=LINE('',#52323,#11285);
#8739=LINE('',#52326,#11286);
#8740=LINE('',#52327,#11287);
#8741=LINE('',#52330,#11288);
#8742=LINE('',#52331,#11289);
#8743=LINE('',#52334,#11290);
#8744=LINE('',#52335,#11291);
#8745=LINE('',#52338,#11292);
#8746=LINE('',#52339,#11293);
#8747=LINE('',#52342,#11294);
#8748=LINE('',#52343,#11295);
#8749=LINE('',#52346,#11296);
#8750=LINE('',#52347,#11297);
#8751=LINE('',#52350,#11298);
#8752=LINE('',#52351,#11299);
#8753=LINE('',#52354,#11300);
#8754=LINE('',#52355,#11301);
#8755=LINE('',#52358,#11302);
#8756=LINE('',#52359,#11303);
#8757=LINE('',#52362,#11304);
#8758=LINE('',#52363,#11305);
#8759=LINE('',#52365,#11306);
#8760=LINE('',#52369,#11307);
#8761=LINE('',#52371,#11308);
#8762=LINE('',#52372,#11309);
#8763=LINE('',#52375,#11310);
#8764=LINE('',#52376,#11311);
#8765=LINE('',#52379,#11312);
#8766=LINE('',#52380,#11313);
#8767=LINE('',#52383,#11314);
#8768=LINE('',#52384,#11315);
#8769=LINE('',#52387,#11316);
#8770=LINE('',#52388,#11317);
#8771=LINE('',#52391,#11318);
#8772=LINE('',#52392,#11319);
#8773=LINE('',#52395,#11320);
#8774=LINE('',#52396,#11321);
#8775=LINE('',#52399,#11322);
#8776=LINE('',#52400,#11323);
#8777=LINE('',#52403,#11324);
#8778=LINE('',#52404,#11325);
#8779=LINE('',#52407,#11326);
#8780=LINE('',#52408,#11327);
#8781=LINE('',#52411,#11328);
#8782=LINE('',#52412,#11329);
#8783=LINE('',#52414,#11330);
#8784=LINE('',#52418,#11331);
#8785=LINE('',#52420,#11332);
#8786=LINE('',#52422,#11333);
#8787=LINE('',#52424,#11334);
#8788=LINE('',#52426,#11335);
#8789=LINE('',#52428,#11336);
#8790=LINE('',#52430,#11337);
#8791=LINE('',#52432,#11338);
#8792=LINE('',#52433,#11339);
#8793=LINE('',#52435,#11340);
#8794=LINE('',#52437,#11341);
#8795=LINE('',#52439,#11342);
#8796=LINE('',#52441,#11343);
#8797=LINE('',#52443,#11344);
#8798=LINE('',#52445,#11345);
#8799=LINE('',#52447,#11346);
#8800=LINE('',#52449,#11347);
#8801=LINE('',#52464,#11348);
#8802=LINE('',#52465,#11349);
#8803=LINE('',#52468,#11350);
#8804=LINE('',#52469,#11351);
#8805=LINE('',#52476,#11352);
#8806=LINE('',#52488,#11353);
#8807=LINE('',#52490,#11354);
#8808=LINE('',#52491,#11355);
#8809=LINE('',#52495,#11356);
#8810=LINE('',#52496,#11357);
#8811=LINE('',#52502,#11358);
#8812=LINE('',#52504,#11359);
#8813=LINE('',#52511,#11360);
#8814=LINE('',#52513,#11361);
#8815=LINE('',#52514,#11362);
#8816=LINE('',#52517,#11363);
#8817=LINE('',#52518,#11364);
#8818=LINE('',#52521,#11365);
#8819=LINE('',#52522,#11366);
#8820=LINE('',#52525,#11367);
#8821=LINE('',#52526,#11368);
#8822=LINE('',#52529,#11369);
#8823=LINE('',#52530,#11370);
#8824=LINE('',#52533,#11371);
#8825=LINE('',#52534,#11372);
#8826=LINE('',#52537,#11373);
#8827=LINE('',#52538,#11374);
#8828=LINE('',#52541,#11375);
#8829=LINE('',#52542,#11376);
#8830=LINE('',#52545,#11377);
#8831=LINE('',#52546,#11378);
#8832=LINE('',#52549,#11379);
#8833=LINE('',#52550,#11380);
#8834=LINE('',#52553,#11381);
#8835=LINE('',#52554,#11382);
#8836=LINE('',#52557,#11383);
#8837=LINE('',#52561,#11384);
#8838=LINE('',#52585,#11385);
#8839=LINE('',#52587,#11386);
#8840=LINE('',#52589,#11387);
#8841=LINE('',#52591,#11388);
#8842=LINE('',#52593,#11389);
#8843=LINE('',#52595,#11390);
#8844=LINE('',#52597,#11391);
#8845=LINE('',#52599,#11392);
#8846=LINE('',#52601,#11393);
#8847=LINE('',#52602,#11394);
#8848=LINE('',#52604,#11395);
#8849=LINE('',#52606,#11396);
#8850=LINE('',#52608,#11397);
#8851=LINE('',#52610,#11398);
#8852=LINE('',#52612,#11399);
#8853=LINE('',#52614,#11400);
#8854=LINE('',#52616,#11401);
#8855=LINE('',#52618,#11402);
#8856=LINE('',#52620,#11403);
#8857=LINE('',#52649,#11404);
#8858=LINE('',#52698,#11405);
#8859=LINE('',#52753,#11406);
#8860=LINE('',#52871,#11407);
#8861=LINE('',#52878,#11408);
#8862=LINE('',#52887,#11409);
#8863=LINE('',#52889,#11410);
#8864=LINE('',#52890,#11411);
#8865=LINE('',#52893,#11412);
#8866=LINE('',#52895,#11413);
#8867=LINE('',#52897,#11414);
#8868=LINE('',#52899,#11415);
#8869=LINE('',#52901,#11416);
#8870=LINE('',#52903,#11417);
#8871=LINE('',#52905,#11418);
#8872=LINE('',#52907,#11419);
#8873=LINE('',#52909,#11420);
#8874=LINE('',#52911,#11421);
#8875=LINE('',#52913,#11422);
#8876=LINE('',#52915,#11423);
#8877=LINE('',#52917,#11424);
#8878=LINE('',#52919,#11425);
#8879=LINE('',#52920,#11426);
#8880=LINE('',#52924,#11427);
#8881=LINE('',#52928,#11428);
#8882=LINE('',#52930,#11429);
#8883=LINE('',#52932,#11430);
#8884=LINE('',#52934,#11431);
#8885=LINE('',#52936,#11432);
#8886=LINE('',#52937,#11433);
#8887=LINE('',#52941,#11434);
#8888=LINE('',#52943,#11435);
#8889=LINE('',#52945,#11436);
#8890=LINE('',#52947,#11437);
#8891=LINE('',#52949,#11438);
#8892=LINE('',#52950,#11439);
#8893=LINE('',#52954,#11440);
#8894=LINE('',#52958,#11441);
#8895=LINE('',#52964,#11442);
#8896=LINE('',#52967,#11443);
#8897=LINE('',#52972,#11444);
#8898=LINE('',#52973,#11445);
#8899=LINE('',#52976,#11446);
#8900=LINE('',#52977,#11447);
#8901=LINE('',#52981,#11448);
#8902=LINE('',#52983,#11449);
#8903=LINE('',#52987,#11450);
#8904=LINE('',#52991,#11451);
#8905=LINE('',#52999,#11452);
#8906=LINE('',#53000,#11453);
#8907=LINE('',#53003,#11454);
#8908=LINE('',#53004,#11455);
#8909=LINE('',#53008,#11456);
#8910=LINE('',#53010,#11457);
#8911=LINE('',#53016,#11458);
#8912=LINE('',#53022,#11459);
#8913=LINE('',#53029,#11460);
#8914=LINE('',#53035,#11461);
#8915=LINE('',#53042,#11462);
#8916=LINE('',#53048,#11463);
#8917=LINE('',#53055,#11464);
#8918=LINE('',#53061,#11465);
#8919=LINE('',#53065,#11466);
#8920=LINE('',#53080,#11467);
#8921=LINE('',#53087,#11468);
#8922=LINE('',#53094,#11469);
#8923=LINE('',#53100,#11470);
#8924=LINE('',#53107,#11471);
#8925=LINE('',#53110,#11472);
#8926=LINE('',#53116,#11473);
#8927=LINE('',#53123,#11474);
#8928=LINE('',#53131,#11475);
#8929=LINE('',#53136,#11476);
#8930=LINE('',#53140,#11477);
#8931=LINE('',#53147,#11478);
#8932=LINE('',#53152,#11479);
#8933=LINE('',#53154,#11480);
#8934=LINE('',#53155,#11481);
#8935=LINE('',#53157,#11482);
#8936=LINE('',#53158,#11483);
#8937=LINE('',#53162,#11484);
#8938=LINE('',#53167,#11485);
#8939=LINE('',#53168,#11486);
#8940=LINE('',#53170,#11487);
#8941=LINE('',#53171,#11488);
#8942=LINE('',#53190,#11489);
#8943=LINE('',#53226,#11490);
#8944=LINE('',#53264,#11491);
#8945=LINE('',#53266,#11492);
#8946=LINE('',#53267,#11493);
#8947=LINE('',#53270,#11494);
#8948=LINE('',#53271,#11495);
#8949=LINE('',#53274,#11496);
#8950=LINE('',#53275,#11497);
#8951=LINE('',#53278,#11498);
#8952=LINE('',#53279,#11499);
#8953=LINE('',#53282,#11500);
#8954=LINE('',#53283,#11501);
#8955=LINE('',#53286,#11502);
#8956=LINE('',#53287,#11503);
#8957=LINE('',#53290,#11504);
#8958=LINE('',#53291,#11505);
#8959=LINE('',#53294,#11506);
#8960=LINE('',#53295,#11507);
#8961=LINE('',#53298,#11508);
#8962=LINE('',#53299,#11509);
#8963=LINE('',#53302,#11510);
#8964=LINE('',#53303,#11511);
#8965=LINE('',#53306,#11512);
#8966=LINE('',#53307,#11513);
#8967=LINE('',#53310,#11514);
#8968=LINE('',#53311,#11515);
#8969=LINE('',#53314,#11516);
#8970=LINE('',#53315,#11517);
#8971=LINE('',#53318,#11518);
#8972=LINE('',#53319,#11519);
#8973=LINE('',#53322,#11520);
#8974=LINE('',#53323,#11521);
#8975=LINE('',#53325,#11522);
#8976=LINE('',#53328,#11523);
#8977=LINE('',#53330,#11524);
#8978=LINE('',#53332,#11525);
#8979=LINE('',#53334,#11526);
#8980=LINE('',#53336,#11527);
#8981=LINE('',#53338,#11528);
#8982=LINE('',#53340,#11529);
#8983=LINE('',#53342,#11530);
#8984=LINE('',#53344,#11531);
#8985=LINE('',#53346,#11532);
#8986=LINE('',#53348,#11533);
#8987=LINE('',#53350,#11534);
#8988=LINE('',#53352,#11535);
#11183=VECTOR('',#39376,10.);
#11184=VECTOR('',#39377,10.);
#11185=VECTOR('',#39378,9.99999999999999);
#11186=VECTOR('',#39381,10.);
#11187=VECTOR('',#39382,10.);
#11188=VECTOR('',#39385,10.);
#11189=VECTOR('',#39386,10.);
#11190=VECTOR('',#39391,10.);
#11191=VECTOR('',#39394,4.08939999999975);
#11192=VECTOR('',#39399,10.);
#11193=VECTOR('',#39404,10.);
#11194=VECTOR('',#39407,10.);
#11195=VECTOR('',#39408,10.);
#11196=VECTOR('',#39411,10.);
#11197=VECTOR('',#39412,10.);
#11198=VECTOR('',#39415,10.);
#11199=VECTOR('',#39416,10.);
#11200=VECTOR('',#39419,10.);
#11201=VECTOR('',#39420,10.);
#11202=VECTOR('',#39423,10.);
#11203=VECTOR('',#39424,10.);
#11204=VECTOR('',#39425,10.);
#11205=VECTOR('',#39428,10.);
#11206=VECTOR('',#39429,10.);
#11207=VECTOR('',#39430,10.);
#11208=VECTOR('',#39435,4.08939999999991);
#11209=VECTOR('',#39446,10.);
#11210=VECTOR('',#39449,10.);
#11211=VECTOR('',#39450,10.);
#11212=VECTOR('',#39451,10.);
#11213=VECTOR('',#39484,10.);
#11214=VECTOR('',#39485,10.);
#11215=VECTOR('',#39486,10.);
#11216=VECTOR('',#39491,10.);
#11217=VECTOR('',#39492,10.);
#11218=VECTOR('',#39501,4.08939999999986);
#11219=VECTOR('',#39506,4.08939999999985);
#11220=VECTOR('',#39513,10.);
#11221=VECTOR('',#39514,10.);
#11222=VECTOR('',#39515,10.);
#11223=VECTOR('',#39520,10.);
#11224=VECTOR('',#39521,10.);
#11225=VECTOR('',#39526,10.);
#11226=VECTOR('',#39527,10.);
#11227=VECTOR('',#39532,10.);
#11228=VECTOR('',#39533,10.);
#11229=VECTOR('',#39538,10.);
#11230=VECTOR('',#39539,10.);
#11231=VECTOR('',#39544,10.);
#11232=VECTOR('',#39545,10.);
#11233=VECTOR('',#39550,10.);
#11234=VECTOR('',#39551,10.);
#11235=VECTOR('',#39556,10.);
#11236=VECTOR('',#39557,10.);
#11237=VECTOR('',#39562,10.);
#11238=VECTOR('',#39563,10.);
#11239=VECTOR('',#39568,10.);
#11240=VECTOR('',#39569,10.);
#11241=VECTOR('',#39574,10.);
#11242=VECTOR('',#39575,10.);
#11243=VECTOR('',#39580,10.);
#11244=VECTOR('',#39589,10.);
#11245=VECTOR('',#39594,10.);
#11246=VECTOR('',#39597,10.);
#11247=VECTOR('',#39600,10.);
#11248=VECTOR('',#39601,10.);
#11249=VECTOR('',#39602,10.);
#11250=VECTOR('',#39609,10.);
#11251=VECTOR('',#39612,10.);
#11252=VECTOR('',#39613,10.);
#11253=VECTOR('',#39614,10.);
#11254=VECTOR('',#39621,10.);
#11255=VECTOR('',#39624,10.);
#11256=VECTOR('',#39625,10.);
#11257=VECTOR('',#39626,10.);
#11258=VECTOR('',#39633,10.);
#11259=VECTOR('',#39636,10.);
#11260=VECTOR('',#39637,10.);
#11261=VECTOR('',#39640,10.);
#11262=VECTOR('',#39641,10.);
#11263=VECTOR('',#39642,10.);
#11264=VECTOR('',#39643,10.);
#11265=VECTOR('',#39650,10.);
#11266=VECTOR('',#39653,10.);
#11267=VECTOR('',#39656,10.);
#11268=VECTOR('',#39659,10.);
#11269=VECTOR('',#39664,10.);
#11270=VECTOR('',#39667,10.);
#11271=VECTOR('',#39670,10.);
#11272=VECTOR('',#39671,10.);
#11273=VECTOR('',#39676,10.);
#11274=VECTOR('',#39679,10.);
#11275=VECTOR('',#39680,10.);
#11276=VECTOR('',#39685,10.);
#11277=VECTOR('',#39688,10.);
#11278=VECTOR('',#39689,10.);
#11279=VECTOR('',#39694,10.);
#11280=VECTOR('',#39697,10.);
#11281=VECTOR('',#39730,4.08940000000001);
#11282=VECTOR('',#39761,4.0894);
#11283=VECTOR('',#39764,10.);
#11284=VECTOR('',#39765,10.);
#11285=VECTOR('',#39766,10.);
#11286=VECTOR('',#39769,10.);
#11287=VECTOR('',#39770,10.);
#11288=VECTOR('',#39773,10.);
#11289=VECTOR('',#39774,10.);
#11290=VECTOR('',#39777,10.);
#11291=VECTOR('',#39778,10.);
#11292=VECTOR('',#39781,10.);
#11293=VECTOR('',#39782,10.);
#11294=VECTOR('',#39785,9.99999999999999);
#11295=VECTOR('',#39786,10.);
#11296=VECTOR('',#39789,10.);
#11297=VECTOR('',#39790,10.);
#11298=VECTOR('',#39793,10.);
#11299=VECTOR('',#39794,10.);
#11300=VECTOR('',#39797,10.);
#11301=VECTOR('',#39798,10.);
#11302=VECTOR('',#39801,10.);
#11303=VECTOR('',#39802,10.);
#11304=VECTOR('',#39805,10.);
#11305=VECTOR('',#39806,10.);
#11306=VECTOR('',#39809,10.);
#11307=VECTOR('',#39814,10.);
#11308=VECTOR('',#39815,10.);
#11309=VECTOR('',#39816,10.);
#11310=VECTOR('',#39819,10.);
#11311=VECTOR('',#39820,10.);
#11312=VECTOR('',#39823,10.);
#11313=VECTOR('',#39824,10.);
#11314=VECTOR('',#39827,10.);
#11315=VECTOR('',#39828,10.);
#11316=VECTOR('',#39831,10.);
#11317=VECTOR('',#39832,10.);
#11318=VECTOR('',#39835,10.);
#11319=VECTOR('',#39836,10.);
#11320=VECTOR('',#39839,10.);
#11321=VECTOR('',#39840,10.);
#11322=VECTOR('',#39843,10.);
#11323=VECTOR('',#39844,10.);
#11324=VECTOR('',#39847,10.);
#11325=VECTOR('',#39848,10.);
#11326=VECTOR('',#39851,10.);
#11327=VECTOR('',#39852,10.);
#11328=VECTOR('',#39855,10.);
#11329=VECTOR('',#39856,10.);
#11330=VECTOR('',#39859,10.);
#11331=VECTOR('',#39864,10.);
#11332=VECTOR('',#39865,10.);
#11333=VECTOR('',#39866,10.);
#11334=VECTOR('',#39867,10.);
#11335=VECTOR('',#39868,10.);
#11336=VECTOR('',#39869,10.);
#11337=VECTOR('',#39870,10.);
#11338=VECTOR('',#39871,10.);
#11339=VECTOR('',#39872,10.);
#11340=VECTOR('',#39875,10.);
#11341=VECTOR('',#39878,10.);
#11342=VECTOR('',#39881,10.);
#11343=VECTOR('',#39884,10.);
#11344=VECTOR('',#39887,10.);
#11345=VECTOR('',#39890,10.);
#11346=VECTOR('',#39893,10.);
#11347=VECTOR('',#39896,10.);
#11348=VECTOR('',#39901,10.);
#11349=VECTOR('',#39902,10.);
#11350=VECTOR('',#39905,10.);
#11351=VECTOR('',#39906,10.);
#11352=VECTOR('',#39917,10.);
#11353=VECTOR('',#39918,10.);
#11354=VECTOR('',#39921,10.);
#11355=VECTOR('',#39922,10.);
#11356=VECTOR('',#39929,10.);
#11357=VECTOR('',#39930,10.);
#11358=VECTOR('',#39939,10.);
#11359=VECTOR('',#39942,10.);
#11360=VECTOR('',#39951,10.);
#11361=VECTOR('',#39952,10.);
#11362=VECTOR('',#39953,10.);
#11363=VECTOR('',#39956,10.);
#11364=VECTOR('',#39957,10.);
#11365=VECTOR('',#39960,10.);
#11366=VECTOR('',#39961,10.);
#11367=VECTOR('',#39964,10.);
#11368=VECTOR('',#39965,10.);
#11369=VECTOR('',#39968,10.);
#11370=VECTOR('',#39969,10.);
#11371=VECTOR('',#39972,10.);
#11372=VECTOR('',#39973,10.);
#11373=VECTOR('',#39976,10.);
#11374=VECTOR('',#39977,10.);
#11375=VECTOR('',#39980,10.);
#11376=VECTOR('',#39981,10.);
#11377=VECTOR('',#39984,10.);
#11378=VECTOR('',#39985,10.);
#11379=VECTOR('',#39988,10.);
#11380=VECTOR('',#39989,10.);
#11381=VECTOR('',#39992,10.);
#11382=VECTOR('',#39993,10.);
#11383=VECTOR('',#39996,11.1759999999998);
#11384=VECTOR('',#40003,10.);
#11385=VECTOR('',#40030,10.);
#11386=VECTOR('',#40031,10.);
#11387=VECTOR('',#40032,10.);
#11388=VECTOR('',#40033,10.);
#11389=VECTOR('',#40034,10.);
#11390=VECTOR('',#40035,10.);
#11391=VECTOR('',#40036,10.);
#11392=VECTOR('',#40037,10.);
#11393=VECTOR('',#40038,10.);
#11394=VECTOR('',#40039,10.);
#11395=VECTOR('',#40042,10.);
#11396=VECTOR('',#40045,10.);
#11397=VECTOR('',#40048,10.);
#11398=VECTOR('',#40051,10.);
#11399=VECTOR('',#40054,10.);
#11400=VECTOR('',#40057,10.);
#11401=VECTOR('',#40060,10.);
#11402=VECTOR('',#40063,10.);
#11403=VECTOR('',#40066,10.);
#11404=VECTOR('',#40077,4.12749999999997);
#11405=VECTOR('',#40090,4.12750000000001);
#11406=VECTOR('',#40103,4.12749999999996);
#11407=VECTOR('',#40130,90.9319999999999);
#11408=VECTOR('',#40139,82.931);
#11409=VECTOR('',#40148,10.);
#11410=VECTOR('',#40149,10.);
#11411=VECTOR('',#40150,10.);
#11412=VECTOR('',#40153,10.);
#11413=VECTOR('',#40154,10.);
#11414=VECTOR('',#40155,10.);
#11415=VECTOR('',#40156,10.);
#11416=VECTOR('',#40157,10.);
#11417=VECTOR('',#40158,10.);
#11418=VECTOR('',#40159,10.);
#11419=VECTOR('',#40160,10.);
#11420=VECTOR('',#40161,10.);
#11421=VECTOR('',#40162,10.);
#11422=VECTOR('',#40163,10.);
#11423=VECTOR('',#40164,10.);
#11424=VECTOR('',#40165,10.);
#11425=VECTOR('',#40166,10.);
#11426=VECTOR('',#40167,10.);
#11427=VECTOR('',#40172,10.);
#11428=VECTOR('',#40175,10.);
#11429=VECTOR('',#40176,10.);
#11430=VECTOR('',#40177,10.);
#11431=VECTOR('',#40178,10.);
#11432=VECTOR('',#40179,10.);
#11433=VECTOR('',#40180,10.);
#11434=VECTOR('',#40183,10.);
#11435=VECTOR('',#40184,10.);
#11436=VECTOR('',#40185,10.);
#11437=VECTOR('',#40186,10.);
#11438=VECTOR('',#40187,10.);
#11439=VECTOR('',#40188,10.);
#11440=VECTOR('',#40191,10.);
#11441=VECTOR('',#40194,10.);
#11442=VECTOR('',#40199,10.);
#11443=VECTOR('',#40202,10.);
#11444=VECTOR('',#40207,10.);
#11445=VECTOR('',#40208,10.);
#11446=VECTOR('',#40211,10.);
#11447=VECTOR('',#40212,10.);
#11448=VECTOR('',#40217,10.);
#11449=VECTOR('',#40220,10.);
#11450=VECTOR('',#40223,10.);
#11451=VECTOR('',#40226,10.);
#11452=VECTOR('',#40237,10.);
#11453=VECTOR('',#40238,10.);
#11454=VECTOR('',#40241,10.);
#11455=VECTOR('',#40242,10.);
#11456=VECTOR('',#40247,10.);
#11457=VECTOR('',#40250,10.);
#11458=VECTOR('',#40257,3.90270999999991);
#11459=VECTOR('',#40264,3.98868900000005);
#11460=VECTOR('',#40273,3.90270999999999);
#11461=VECTOR('',#40280,3.98868900000002);
#11462=VECTOR('',#40289,3.90271000000012);
#11463=VECTOR('',#40296,3.98868900000004);
#11464=VECTOR('',#40305,3.90271);
#11465=VECTOR('',#40312,3.98868900000001);
#11466=VECTOR('',#40317,82.8587325401841);
#11467=VECTOR('',#40334,57.15);
#11468=VECTOR('',#40343,52.451);
#11469=VECTOR('',#40352,13.081);
#11470=VECTOR('',#40361,12.446);
#11471=VECTOR('',#40370,8.76299999999995);
#11472=VECTOR('',#40373,2.794);
#11473=VECTOR('',#40382,8.76299999999997);
#11474=VECTOR('',#40391,2.794);
#11475=VECTOR('',#40402,2.79400000000002);
#11476=VECTOR('',#40409,8.76300000000001);
#11477=VECTOR('',#40414,8.763);
#11478=VECTOR('',#40423,2.79399999999998);
#11479=VECTOR('',#40428,10.);
#11480=VECTOR('',#40429,10.);
#11481=VECTOR('',#40430,10.);
#11482=VECTOR('',#40431,10.);
#11483=VECTOR('',#40432,10.);
#11484=VECTOR('',#40435,10.);
#11485=VECTOR('',#40442,10.);
#11486=VECTOR('',#40443,10.);
#11487=VECTOR('',#40444,10.);
#11488=VECTOR('',#40445,10.);
#11489=VECTOR('',#40476,2.18439999999999);
#11490=VECTOR('',#40519,2.18440000000006);
#11491=VECTOR('',#40560,10.);
#11492=VECTOR('',#40561,10.);
#11493=VECTOR('',#40562,10.);
#11494=VECTOR('',#40565,10.);
#11495=VECTOR('',#40566,10.);
#11496=VECTOR('',#40569,10.);
#11497=VECTOR('',#40570,10.);
#11498=VECTOR('',#40573,10.);
#11499=VECTOR('',#40574,10.);
#11500=VECTOR('',#40577,10.);
#11501=VECTOR('',#40578,10.);
#11502=VECTOR('',#40581,10.);
#11503=VECTOR('',#40582,10.);
#11504=VECTOR('',#40585,10.);
#11505=VECTOR('',#40586,10.);
#11506=VECTOR('',#40589,10.);
#11507=VECTOR('',#40590,10.);
#11508=VECTOR('',#40593,10.);
#11509=VECTOR('',#40594,10.);
#11510=VECTOR('',#40597,10.);
#11511=VECTOR('',#40598,10.);
#11512=VECTOR('',#40601,10.);
#11513=VECTOR('',#40602,10.);
#11514=VECTOR('',#40605,10.);
#11515=VECTOR('',#40606,10.);
#11516=VECTOR('',#40609,10.);
#11517=VECTOR('',#40610,10.);
#11518=VECTOR('',#40613,10.);
#11519=VECTOR('',#40614,10.);
#11520=VECTOR('',#40617,10.);
#11521=VECTOR('',#40618,10.);
#11522=VECTOR('',#40621,10.);
#11523=VECTOR('',#40626,10.);
#11524=VECTOR('',#40629,10.);
#11525=VECTOR('',#40632,10.);
#11526=VECTOR('',#40635,10.);
#11527=VECTOR('',#40638,10.);
#11528=VECTOR('',#40641,10.);
#11529=VECTOR('',#40644,10.);
#11530=VECTOR('',#40647,10.);
#11531=VECTOR('',#40650,10.);
#11532=VECTOR('',#40653,10.);
#11533=VECTOR('',#40656,10.);
#11534=VECTOR('',#40659,10.);
#11535=VECTOR('',#40662,10.);
#13796=VERTEX_POINT('',#51592);
#13797=VERTEX_POINT('',#51593);
#13798=VERTEX_POINT('',#51598);
#13799=VERTEX_POINT('',#51602);
#13800=VERTEX_POINT('',#51605);
#13801=VERTEX_POINT('',#51610);
#13802=VERTEX_POINT('',#51619);
#13803=VERTEX_POINT('',#51628);
#13804=VERTEX_POINT('',#51636);
#13805=VERTEX_POINT('',#51645);
#13806=VERTEX_POINT('',#51654);
#13807=VERTEX_POINT('',#51662);
#13808=VERTEX_POINT('',#51671);
#13809=VERTEX_POINT('',#51680);
#13810=VERTEX_POINT('',#51688);
#13811=VERTEX_POINT('',#51706);
#13812=VERTEX_POINT('',#51708);
#13813=VERTEX_POINT('',#51712);
#13814=VERTEX_POINT('',#51716);
#13815=VERTEX_POINT('',#51720);
#13816=VERTEX_POINT('',#51721);
#13817=VERTEX_POINT('',#51725);
#13818=VERTEX_POINT('',#51748);
#13819=VERTEX_POINT('',#51749);
#13820=VERTEX_POINT('',#51751);
#13821=VERTEX_POINT('',#51762);
#13822=VERTEX_POINT('',#51764);
#13823=VERTEX_POINT('',#51766);
#13824=VERTEX_POINT('',#51785);
#13825=VERTEX_POINT('',#51787);
#13826=VERTEX_POINT('',#51789);
#13827=VERTEX_POINT('',#51800);
#13828=VERTEX_POINT('',#51803);
#13829=VERTEX_POINT('',#51804);
#13830=VERTEX_POINT('',#51815);
#13831=VERTEX_POINT('',#51828);
#13832=VERTEX_POINT('',#51830);
#13833=VERTEX_POINT('',#51852);
#13834=VERTEX_POINT('',#51853);
#13835=VERTEX_POINT('',#51873);
#13836=VERTEX_POINT('',#51875);
#13837=VERTEX_POINT('',#51896);
#13838=VERTEX_POINT('',#51897);
#13839=VERTEX_POINT('',#51899);
#13840=VERTEX_POINT('',#51910);
#13841=VERTEX_POINT('',#51923);
#13842=VERTEX_POINT('',#51925);
#13843=VERTEX_POINT('',#51929);
#13844=VERTEX_POINT('',#51931);
#13845=VERTEX_POINT('',#51935);
#13846=VERTEX_POINT('',#51936);
#13847=VERTEX_POINT('',#51938);
#13848=VERTEX_POINT('',#51949);
#13849=VERTEX_POINT('',#51963);
#13850=VERTEX_POINT('',#51966);
#13851=VERTEX_POINT('',#51968);
#13852=VERTEX_POINT('',#51970);
#13853=VERTEX_POINT('',#51981);
#13854=VERTEX_POINT('',#51985);
#13855=VERTEX_POINT('',#51986);
#13856=VERTEX_POINT('',#51988);
#13857=VERTEX_POINT('',#52011);
#13858=VERTEX_POINT('',#52012);
#13859=VERTEX_POINT('',#52014);
#13860=VERTEX_POINT('',#52016);
#13861=VERTEX_POINT('',#52018);
#13862=VERTEX_POINT('',#52020);
#13863=VERTEX_POINT('',#52022);
#13864=VERTEX_POINT('',#52024);
#13865=VERTEX_POINT('',#52026);
#13866=VERTEX_POINT('',#52028);
#13867=VERTEX_POINT('',#52030);
#13868=VERTEX_POINT('',#52032);
#13869=VERTEX_POINT('',#52036);
#13870=VERTEX_POINT('',#52037);
#13871=VERTEX_POINT('',#52039);
#13872=VERTEX_POINT('',#52041);
#13873=VERTEX_POINT('',#52045);
#13874=VERTEX_POINT('',#52047);
#13875=VERTEX_POINT('',#52053);
#13876=VERTEX_POINT('',#52058);
#13877=VERTEX_POINT('',#52062);
#13878=VERTEX_POINT('',#52063);
#13879=VERTEX_POINT('',#52065);
#13880=VERTEX_POINT('',#52067);
#13881=VERTEX_POINT('',#52071);
#13882=VERTEX_POINT('',#52073);
#13883=VERTEX_POINT('',#52077);
#13884=VERTEX_POINT('',#52079);
#13885=VERTEX_POINT('',#52083);
#13886=VERTEX_POINT('',#52085);
#13887=VERTEX_POINT('',#52089);
#13888=VERTEX_POINT('',#52091);
#13889=VERTEX_POINT('',#52095);
#13890=VERTEX_POINT('',#52097);
#13891=VERTEX_POINT('',#52101);
#13892=VERTEX_POINT('',#52103);
#13893=VERTEX_POINT('',#52107);
#13894=VERTEX_POINT('',#52109);
#13895=VERTEX_POINT('',#52113);
#13896=VERTEX_POINT('',#52115);
#13897=VERTEX_POINT('',#52119);
#13898=VERTEX_POINT('',#52121);
#13899=VERTEX_POINT('',#52125);
#13900=VERTEX_POINT('',#52127);
#13901=VERTEX_POINT('',#52137);
#13902=VERTEX_POINT('',#52150);
#13903=VERTEX_POINT('',#52151);
#13904=VERTEX_POINT('',#52153);
#13905=VERTEX_POINT('',#52155);
#13906=VERTEX_POINT('',#52159);
#13907=VERTEX_POINT('',#52161);
#13908=VERTEX_POINT('',#52165);
#13909=VERTEX_POINT('',#52167);
#13910=VERTEX_POINT('',#52171);
#13911=VERTEX_POINT('',#52173);
#13912=VERTEX_POINT('',#52177);
#13913=VERTEX_POINT('',#52179);
#13914=VERTEX_POINT('',#52183);
#13915=VERTEX_POINT('',#52185);
#13916=VERTEX_POINT('',#52189);
#13917=VERTEX_POINT('',#52191);
#13918=VERTEX_POINT('',#52198);
#13919=VERTEX_POINT('',#52199);
#13920=VERTEX_POINT('',#52201);
#13921=VERTEX_POINT('',#52203);
#13922=VERTEX_POINT('',#52207);
#13923=VERTEX_POINT('',#52209);
#13924=VERTEX_POINT('',#52211);
#13925=VERTEX_POINT('',#52212);
#13926=VERTEX_POINT('',#52214);
#13927=VERTEX_POINT('',#52216);
#13928=VERTEX_POINT('',#52218);
#13929=VERTEX_POINT('',#52220);
#13930=VERTEX_POINT('',#52222);
#13931=VERTEX_POINT('',#52224);
#13932=VERTEX_POINT('',#52228);
#13933=VERTEX_POINT('',#52230);
#13934=VERTEX_POINT('',#52234);
#13935=VERTEX_POINT('',#52238);
#13936=VERTEX_POINT('',#52242);
#13937=VERTEX_POINT('',#52246);
#13938=VERTEX_POINT('',#52250);
#13939=VERTEX_POINT('',#52254);
#13940=VERTEX_POINT('',#52261);
#13941=VERTEX_POINT('',#52263);
#13942=VERTEX_POINT('',#52264);
#13943=VERTEX_POINT('',#52266);
#13944=VERTEX_POINT('',#52268);
#13945=VERTEX_POINT('',#52270);
#13946=VERTEX_POINT('',#52272);
#13947=VERTEX_POINT('',#52274);
#13948=VERTEX_POINT('',#52276);
#13949=VERTEX_POINT('',#52278);
#13950=VERTEX_POINT('',#52280);
#13951=VERTEX_POINT('',#52282);
#13952=VERTEX_POINT('',#52284);
#13953=VERTEX_POINT('',#52290);
#13954=VERTEX_POINT('',#52292);
#13955=VERTEX_POINT('',#52293);
#13956=VERTEX_POINT('',#52295);
#13957=VERTEX_POINT('',#52297);
#13958=VERTEX_POINT('',#52299);
#13959=VERTEX_POINT('',#52301);
#13960=VERTEX_POINT('',#52303);
#13961=VERTEX_POINT('',#52305);
#13962=VERTEX_POINT('',#52307);
#13963=VERTEX_POINT('',#52309);
#13964=VERTEX_POINT('',#52311);
#13965=VERTEX_POINT('',#52313);
#13966=VERTEX_POINT('',#52319);
#13967=VERTEX_POINT('',#52321);
#13968=VERTEX_POINT('',#52325);
#13969=VERTEX_POINT('',#52329);
#13970=VERTEX_POINT('',#52333);
#13971=VERTEX_POINT('',#52337);
#13972=VERTEX_POINT('',#52341);
#13973=VERTEX_POINT('',#52345);
#13974=VERTEX_POINT('',#52349);
#13975=VERTEX_POINT('',#52353);
#13976=VERTEX_POINT('',#52357);
#13977=VERTEX_POINT('',#52361);
#13978=VERTEX_POINT('',#52368);
#13979=VERTEX_POINT('',#52370);
#13980=VERTEX_POINT('',#52374);
#13981=VERTEX_POINT('',#52378);
#13982=VERTEX_POINT('',#52382);
#13983=VERTEX_POINT('',#52386);
#13984=VERTEX_POINT('',#52390);
#13985=VERTEX_POINT('',#52394);
#13986=VERTEX_POINT('',#52398);
#13987=VERTEX_POINT('',#52402);
#13988=VERTEX_POINT('',#52406);
#13989=VERTEX_POINT('',#52410);
#13990=VERTEX_POINT('',#52417);
#13991=VERTEX_POINT('',#52419);
#13992=VERTEX_POINT('',#52421);
#13993=VERTEX_POINT('',#52423);
#13994=VERTEX_POINT('',#52425);
#13995=VERTEX_POINT('',#52427);
#13996=VERTEX_POINT('',#52429);
#13997=VERTEX_POINT('',#52431);
#13998=VERTEX_POINT('',#52452);
#13999=VERTEX_POINT('',#52453);
#14000=VERTEX_POINT('',#52467);
#14001=VERTEX_POINT('',#52475);
#14002=VERTEX_POINT('',#52477);
#14003=VERTEX_POINT('',#52500);
#14004=VERTEX_POINT('',#52506);
#14005=VERTEX_POINT('',#52510);
#14006=VERTEX_POINT('',#52512);
#14007=VERTEX_POINT('',#52516);
#14008=VERTEX_POINT('',#52520);
#14009=VERTEX_POINT('',#52524);
#14010=VERTEX_POINT('',#52528);
#14011=VERTEX_POINT('',#52532);
#14012=VERTEX_POINT('',#52536);
#14013=VERTEX_POINT('',#52540);
#14014=VERTEX_POINT('',#52544);
#14015=VERTEX_POINT('',#52548);
#14016=VERTEX_POINT('',#52552);
#14017=VERTEX_POINT('',#52556);
#14018=VERTEX_POINT('',#52564);
#14019=VERTEX_POINT('',#52566);
#14020=VERTEX_POINT('',#52568);
#14021=VERTEX_POINT('',#52570);
#14022=VERTEX_POINT('',#52572);
#14023=VERTEX_POINT('',#52574);
#14024=VERTEX_POINT('',#52576);
#14025=VERTEX_POINT('',#52578);
#14026=VERTEX_POINT('',#52580);
#14027=VERTEX_POINT('',#52584);
#14028=VERTEX_POINT('',#52586);
#14029=VERTEX_POINT('',#52588);
#14030=VERTEX_POINT('',#52590);
#14031=VERTEX_POINT('',#52592);
#14032=VERTEX_POINT('',#52594);
#14033=VERTEX_POINT('',#52596);
#14034=VERTEX_POINT('',#52598);
#14035=VERTEX_POINT('',#52600);
#14036=VERTEX_POINT('',#52623);
#14037=VERTEX_POINT('',#52625);
#14038=VERTEX_POINT('',#52628);
#14039=VERTEX_POINT('',#52629);
#14040=VERTEX_POINT('',#52648);
#14041=VERTEX_POINT('',#52650);
#14042=VERTEX_POINT('',#52672);
#14043=VERTEX_POINT('',#52673);
#14044=VERTEX_POINT('',#52677);
#14045=VERTEX_POINT('',#52678);
#14046=VERTEX_POINT('',#52697);
#14047=VERTEX_POINT('',#52699);
#14048=VERTEX_POINT('',#52721);
#14049=VERTEX_POINT('',#52722);
#14050=VERTEX_POINT('',#52724);
#14051=VERTEX_POINT('',#52732);
#14052=VERTEX_POINT('',#52733);
#14053=VERTEX_POINT('',#52752);
#14054=VERTEX_POINT('',#52802);
#14055=VERTEX_POINT('',#52803);
#14056=VERTEX_POINT('',#52863);
#14057=VERTEX_POINT('',#52864);
#14058=VERTEX_POINT('',#52867);
#14059=VERTEX_POINT('',#52874);
#14060=VERTEX_POINT('',#52877);
#14061=VERTEX_POINT('',#52879);
#14062=VERTEX_POINT('',#52883);
#14063=VERTEX_POINT('',#52884);
#14064=VERTEX_POINT('',#52886);
#14065=VERTEX_POINT('',#52888);
#14066=VERTEX_POINT('',#52892);
#14067=VERTEX_POINT('',#52894);
#14068=VERTEX_POINT('',#52896);
#14069=VERTEX_POINT('',#52898);
#14070=VERTEX_POINT('',#52900);
#14071=VERTEX_POINT('',#52902);
#14072=VERTEX_POINT('',#52904);
#14073=VERTEX_POINT('',#52906);
#14074=VERTEX_POINT('',#52908);
#14075=VERTEX_POINT('',#52910);
#14076=VERTEX_POINT('',#52912);
#14077=VERTEX_POINT('',#52914);
#14078=VERTEX_POINT('',#52916);
#14079=VERTEX_POINT('',#52918);
#14080=VERTEX_POINT('',#52922);
#14081=VERTEX_POINT('',#52926);
#14082=VERTEX_POINT('',#52927);
#14083=VERTEX_POINT('',#52929);
#14084=VERTEX_POINT('',#52931);
#14085=VERTEX_POINT('',#52933);
#14086=VERTEX_POINT('',#52935);
#14087=VERTEX_POINT('',#52939);
#14088=VERTEX_POINT('',#52940);
#14089=VERTEX_POINT('',#52942);
#14090=VERTEX_POINT('',#52944);
#14091=VERTEX_POINT('',#52946);
#14092=VERTEX_POINT('',#52948);
#14093=VERTEX_POINT('',#52952);
#14094=VERTEX_POINT('',#52953);
#14095=VERTEX_POINT('',#52955);
#14096=VERTEX_POINT('',#52957);
#14097=VERTEX_POINT('',#52960);
#14098=VERTEX_POINT('',#52961);
#14099=VERTEX_POINT('',#52963);
#14100=VERTEX_POINT('',#52965);
#14101=VERTEX_POINT('',#52969);
#14102=VERTEX_POINT('',#52970);
#14103=VERTEX_POINT('',#52975);
#14104=VERTEX_POINT('',#52979);
#14105=VERTEX_POINT('',#52985);
#14106=VERTEX_POINT('',#52986);
#14107=VERTEX_POINT('',#52988);
#14108=VERTEX_POINT('',#52990);
#14109=VERTEX_POINT('',#52996);
#14110=VERTEX_POINT('',#52997);
#14111=VERTEX_POINT('',#53002);
#14112=VERTEX_POINT('',#53006);
#14113=VERTEX_POINT('',#53012);
#14114=VERTEX_POINT('',#53015);
#14115=VERTEX_POINT('',#53017);
#14116=VERTEX_POINT('',#53021);
#14117=VERTEX_POINT('',#53025);
#14118=VERTEX_POINT('',#53028);
#14119=VERTEX_POINT('',#53030);
#14120=VERTEX_POINT('',#53034);
#14121=VERTEX_POINT('',#53038);
#14122=VERTEX_POINT('',#53041);
#14123=VERTEX_POINT('',#53043);
#14124=VERTEX_POINT('',#53047);
#14125=VERTEX_POINT('',#53051);
#14126=VERTEX_POINT('',#53054);
#14127=VERTEX_POINT('',#53056);
#14128=VERTEX_POINT('',#53060);
#14129=VERTEX_POINT('',#53064);
#14130=VERTEX_POINT('',#53068);
#14131=VERTEX_POINT('',#53070);
#14132=VERTEX_POINT('',#53072);
#14133=VERTEX_POINT('',#53074);
#14134=VERTEX_POINT('',#53076);
#14135=VERTEX_POINT('',#53079);
#14136=VERTEX_POINT('',#53083);
#14137=VERTEX_POINT('',#53086);
#14138=VERTEX_POINT('',#53090);
#14139=VERTEX_POINT('',#53093);
#14140=VERTEX_POINT('',#53097);
#14141=VERTEX_POINT('',#53102);
#14142=VERTEX_POINT('',#53104);
#14143=VERTEX_POINT('',#53109);
#14144=VERTEX_POINT('',#53114);
#14145=VERTEX_POINT('',#53118);
#14146=VERTEX_POINT('',#53121);
#14147=VERTEX_POINT('',#53126);
#14148=VERTEX_POINT('',#53129);
#14149=VERTEX_POINT('',#53133);
#14150=VERTEX_POINT('',#53138);
#14151=VERTEX_POINT('',#53142);
#14152=VERTEX_POINT('',#53145);
#14153=VERTEX_POINT('',#53150);
#14154=VERTEX_POINT('',#53151);
#14155=VERTEX_POINT('',#53153);
#14156=VERTEX_POINT('',#53156);
#14157=VERTEX_POINT('',#53160);
#14158=VERTEX_POINT('',#53161);
#14159=VERTEX_POINT('',#53166);
#14160=VERTEX_POINT('',#53169);
#14161=VERTEX_POINT('',#53175);
#14162=VERTEX_POINT('',#53183);
#14163=VERTEX_POINT('',#53189);
#14164=VERTEX_POINT('',#53194);
#14165=VERTEX_POINT('',#53195);
#14166=VERTEX_POINT('',#53197);
#14167=VERTEX_POINT('',#53199);
#14168=VERTEX_POINT('',#53201);
#14169=VERTEX_POINT('',#53203);
#14170=VERTEX_POINT('',#53205);
#14171=VERTEX_POINT('',#53207);
#14172=VERTEX_POINT('',#53209);
#14173=VERTEX_POINT('',#53212);
#14174=VERTEX_POINT('',#53214);
#14175=VERTEX_POINT('',#53216);
#14176=VERTEX_POINT('',#53218);
#14177=VERTEX_POINT('',#53223);
#14178=VERTEX_POINT('',#53230);
#14179=VERTEX_POINT('',#53231);
#14180=VERTEX_POINT('',#53233);
#14181=VERTEX_POINT('',#53235);
#14182=VERTEX_POINT('',#53237);
#14183=VERTEX_POINT('',#53239);
#14184=VERTEX_POINT('',#53241);
#14185=VERTEX_POINT('',#53243);
#14186=VERTEX_POINT('',#53245);
#14187=VERTEX_POINT('',#53247);
#14188=VERTEX_POINT('',#53249);
#14189=VERTEX_POINT('',#53251);
#14190=VERTEX_POINT('',#53253);
#14191=VERTEX_POINT('',#53255);
#14192=VERTEX_POINT('',#53257);
#14193=VERTEX_POINT('',#53259);
#14194=VERTEX_POINT('',#53263);
#14195=VERTEX_POINT('',#53265);
#14196=VERTEX_POINT('',#53269);
#14197=VERTEX_POINT('',#53273);
#14198=VERTEX_POINT('',#53277);
#14199=VERTEX_POINT('',#53281);
#14200=VERTEX_POINT('',#53285);
#14201=VERTEX_POINT('',#53289);
#14202=VERTEX_POINT('',#53293);
#14203=VERTEX_POINT('',#53297);
#14204=VERTEX_POINT('',#53301);
#14205=VERTEX_POINT('',#53305);
#14206=VERTEX_POINT('',#53309);
#14207=VERTEX_POINT('',#53313);
#14208=VERTEX_POINT('',#53317);
#14209=VERTEX_POINT('',#53321);
#17201=EDGE_CURVE('',#13796,#13797,#778,.F.);
#17202=EDGE_CURVE('',#13797,#13798,#509,.T.);
#17203=EDGE_CURVE('',#13799,#13798,#2448,.T.);
#17204=EDGE_CURVE('',#13798,#13799,#2449,.T.);
#17205=EDGE_CURVE('',#13797,#13800,#779,.F.);
#17206=EDGE_CURVE('',#13800,#13801,#780,.T.);
#17207=EDGE_CURVE('',#13801,#13802,#781,.T.);
#17208=EDGE_CURVE('',#13802,#13803,#782,.T.);
#17209=EDGE_CURVE('',#13803,#13804,#783,.T.);
#17210=EDGE_CURVE('',#13804,#13805,#784,.T.);
#17211=EDGE_CURVE('',#13805,#13806,#785,.T.);
#17212=EDGE_CURVE('',#13806,#13807,#786,.T.);
#17213=EDGE_CURVE('',#13807,#13808,#787,.T.);
#17214=EDGE_CURVE('',#13808,#13809,#788,.T.);
#17215=EDGE_CURVE('',#13809,#13810,#789,.T.);
#17216=EDGE_CURVE('',#13810,#13796,#790,.T.);
#17217=EDGE_CURVE('',#13811,#13801,#8636,.T.);
#17218=EDGE_CURVE('',#13812,#13811,#8637,.T.);
#17219=EDGE_CURVE('',#13812,#13802,#8638,.T.);
#17220=EDGE_CURVE('',#13813,#13812,#8639,.T.);
#17221=EDGE_CURVE('',#13813,#13803,#8640,.T.);
#17222=EDGE_CURVE('',#13814,#13813,#8641,.T.);
#17223=EDGE_CURVE('',#13814,#13804,#8642,.T.);
#17224=EDGE_CURVE('',#13815,#13816,#2450,.T.);
#17225=EDGE_CURVE('',#13816,#13815,#8643,.T.);
#17226=EDGE_CURVE('',#13799,#13817,#8644,.T.);
#17227=EDGE_CURVE('',#13817,#13816,#791,.T.);
#17228=EDGE_CURVE('',#13815,#13817,#792,.T.);
#17229=EDGE_CURVE('',#13818,#13819,#2451,.T.);
#17230=EDGE_CURVE('',#13818,#13820,#793,.T.);
#17231=EDGE_CURVE('',#13820,#13821,#8645,.T.);
#17232=EDGE_CURVE('',#13821,#13822,#2452,.T.);
#17233=EDGE_CURVE('',#13823,#13822,#794,.T.);
#17234=EDGE_CURVE('',#13823,#13824,#2453,.T.);
#17235=EDGE_CURVE('',#13824,#13825,#8646,.T.);
#17236=EDGE_CURVE('',#13825,#13826,#795,.T.);
#17237=EDGE_CURVE('',#13826,#13827,#2454,.T.);
#17238=EDGE_CURVE('',#13819,#13827,#8647,.T.);
#17239=EDGE_CURVE('',#13828,#13829,#796,.T.);
#17240=EDGE_CURVE('',#13830,#13828,#8648,.T.);
#17241=EDGE_CURVE('',#13829,#13830,#797,.T.);
#17242=EDGE_CURVE('',#13831,#13823,#8649,.T.);
#17243=EDGE_CURVE('',#13832,#13822,#8650,.T.);
#17244=EDGE_CURVE('',#13831,#13832,#798,.T.);
#17245=EDGE_CURVE('',#13833,#13834,#799,.T.);
#17246=EDGE_CURVE('',#13835,#13834,#8651,.T.);
#17247=EDGE_CURVE('',#13836,#13835,#800,.T.);
#17248=EDGE_CURVE('',#13836,#13833,#8652,.T.);
#17249=EDGE_CURVE('',#13837,#13838,#8653,.T.);
#17250=EDGE_CURVE('',#13839,#13838,#801,.T.);
#17251=EDGE_CURVE('',#13839,#13840,#8654,.T.);
#17252=EDGE_CURVE('',#13837,#13840,#802,.T.);
#17253=EDGE_CURVE('',#13841,#13839,#8655,.T.);
#17254=EDGE_CURVE('',#13841,#13842,#8656,.T.);
#17255=EDGE_CURVE('',#13840,#13842,#8657,.T.);
#17256=EDGE_CURVE('',#13843,#13821,#8658,.T.);
#17257=EDGE_CURVE('',#13844,#13820,#8659,.T.);
#17258=EDGE_CURVE('',#13843,#13844,#8660,.T.);
#17259=EDGE_CURVE('',#13845,#13846,#2455,.T.);
#17260=EDGE_CURVE('',#13846,#13847,#803,.T.);
#17261=EDGE_CURVE('',#13847,#13848,#8661,.T.);
#17262=EDGE_CURVE('',#13848,#13848,#2456,.T.);
#17263=EDGE_CURVE('',#13847,#13845,#804,.T.);
#17264=EDGE_CURVE('',#13849,#13837,#2457,.T.);
#17265=EDGE_CURVE('',#13842,#13834,#2458,.T.);
#17266=EDGE_CURVE('',#13833,#13850,#2459,.T.);
#17267=EDGE_CURVE('',#13850,#13851,#8662,.T.);
#17268=EDGE_CURVE('',#13851,#13852,#805,.T.);
#17269=EDGE_CURVE('',#13853,#13852,#2460,.T.);
#17270=EDGE_CURVE('',#13853,#13849,#8663,.T.);
#17271=EDGE_CURVE('',#13845,#13846,#8664,.T.);
#17272=EDGE_CURVE('',#13854,#13855,#8665,.T.);
#17273=EDGE_CURVE('',#13856,#13854,#806,.T.);
#17274=EDGE_CURVE('',#13855,#13856,#807,.T.);
#17275=EDGE_CURVE('',#13857,#13858,#2461,.T.);
#17276=EDGE_CURVE('',#13858,#13859,#2462,.T.);
#17277=EDGE_CURVE('',#13859,#13860,#2463,.T.);
#17278=EDGE_CURVE('',#13860,#13861,#2464,.T.);
#17279=EDGE_CURVE('',#13861,#13862,#2465,.T.);
#17280=EDGE_CURVE('',#13862,#13863,#2466,.T.);
#17281=EDGE_CURVE('',#13863,#13864,#2467,.T.);
#17282=EDGE_CURVE('',#13864,#13865,#2468,.T.);
#17283=EDGE_CURVE('',#13865,#13866,#2469,.T.);
#17284=EDGE_CURVE('',#13866,#13867,#2470,.T.);
#17285=EDGE_CURVE('',#13867,#13868,#2471,.T.);
#17286=EDGE_CURVE('',#13868,#13857,#2472,.T.);
#17287=EDGE_CURVE('',#13869,#13870,#2473,.T.);
#17288=EDGE_CURVE('',#13871,#13869,#8666,.T.);
#17289=EDGE_CURVE('',#13872,#13871,#8667,.T.);
#17290=EDGE_CURVE('',#13872,#13870,#8668,.T.);
#17291=EDGE_CURVE('',#13873,#13869,#2474,.T.);
#17292=EDGE_CURVE('',#13874,#13873,#8669,.T.);
#17293=EDGE_CURVE('',#13871,#13874,#8670,.T.);
#17294=EDGE_CURVE('',#13828,#13830,#2475,.T.);
#17295=EDGE_CURVE('',#13875,#13875,#2476,.T.);
#17296=EDGE_CURVE('',#13875,#13829,#8671,.T.);
#17297=EDGE_CURVE('',#13854,#13855,#2477,.T.);
#17298=EDGE_CURVE('',#13856,#13876,#8672,.T.);
#17299=EDGE_CURVE('',#13876,#13876,#2478,.T.);
#17300=EDGE_CURVE('',#13877,#13878,#2479,.T.);
#17301=EDGE_CURVE('',#13879,#13877,#8673,.T.);
#17302=EDGE_CURVE('',#13880,#13879,#8674,.T.);
#17303=EDGE_CURVE('',#13880,#13878,#8675,.T.);
#17304=EDGE_CURVE('',#13881,#13877,#2480,.T.);
#17305=EDGE_CURVE('',#13882,#13881,#8676,.T.);
#17306=EDGE_CURVE('',#13879,#13882,#8677,.T.);
#17307=EDGE_CURVE('',#13883,#13881,#2481,.T.);
#17308=EDGE_CURVE('',#13884,#13883,#8678,.T.);
#17309=EDGE_CURVE('',#13882,#13884,#8679,.T.);
#17310=EDGE_CURVE('',#13885,#13883,#2482,.T.);
#17311=EDGE_CURVE('',#13886,#13885,#8680,.T.);
#17312=EDGE_CURVE('',#13884,#13886,#8681,.T.);
#17313=EDGE_CURVE('',#13887,#13885,#2483,.T.);
#17314=EDGE_CURVE('',#13888,#13887,#8682,.T.);
#17315=EDGE_CURVE('',#13886,#13888,#8683,.T.);
#17316=EDGE_CURVE('',#13889,#13887,#2484,.T.);
#17317=EDGE_CURVE('',#13890,#13889,#8684,.T.);
#17318=EDGE_CURVE('',#13888,#13890,#8685,.T.);
#17319=EDGE_CURVE('',#13891,#13889,#2485,.T.);
#17320=EDGE_CURVE('',#13892,#13891,#8686,.T.);
#17321=EDGE_CURVE('',#13890,#13892,#8687,.T.);
#17322=EDGE_CURVE('',#13893,#13891,#2486,.T.);
#17323=EDGE_CURVE('',#13894,#13893,#8688,.T.);
#17324=EDGE_CURVE('',#13892,#13894,#8689,.T.);
#17325=EDGE_CURVE('',#13895,#13893,#2487,.T.);
#17326=EDGE_CURVE('',#13896,#13895,#8690,.T.);
#17327=EDGE_CURVE('',#13894,#13896,#8691,.T.);
#17328=EDGE_CURVE('',#13897,#13895,#2488,.T.);
#17329=EDGE_CURVE('',#13898,#13897,#8692,.T.);
#17330=EDGE_CURVE('',#13896,#13898,#8693,.T.);
#17331=EDGE_CURVE('',#13899,#13897,#2489,.T.);
#17332=EDGE_CURVE('',#13900,#13899,#8694,.T.);
#17333=EDGE_CURVE('',#13898,#13900,#8695,.T.);
#17334=EDGE_CURVE('',#13878,#13899,#2490,.T.);
#17335=EDGE_CURVE('',#13900,#13880,#8696,.T.);
#17336=EDGE_CURVE('',#13844,#13901,#808,.T.);
#17337=EDGE_CURVE('',#13818,#13901,#8697,.T.);
#17338=EDGE_CURVE('',#13902,#13903,#2491,.T.);
#17339=EDGE_CURVE('',#13904,#13902,#8698,.T.);
#17340=EDGE_CURVE('',#13904,#13905,#2492,.T.);
#17341=EDGE_CURVE('',#13905,#13903,#8699,.T.);
#17342=EDGE_CURVE('',#13903,#13906,#8700,.T.);
#17343=EDGE_CURVE('',#13905,#13907,#8701,.T.);
#17344=EDGE_CURVE('',#13907,#13906,#8702,.T.);
#17345=EDGE_CURVE('',#13906,#13908,#2493,.T.);
#17346=EDGE_CURVE('',#13907,#13909,#2494,.T.);
#17347=EDGE_CURVE('',#13909,#13908,#8703,.T.);
#17348=EDGE_CURVE('',#13908,#13910,#8704,.T.);
#17349=EDGE_CURVE('',#13909,#13911,#8705,.T.);
#17350=EDGE_CURVE('',#13911,#13910,#8706,.T.);
#17351=EDGE_CURVE('',#13910,#13912,#2495,.T.);
#17352=EDGE_CURVE('',#13911,#13913,#2496,.T.);
#17353=EDGE_CURVE('',#13913,#13912,#8707,.T.);
#17354=EDGE_CURVE('',#13912,#13914,#8708,.T.);
#17355=EDGE_CURVE('',#13913,#13915,#8709,.T.);
#17356=EDGE_CURVE('',#13915,#13914,#8710,.T.);
#17357=EDGE_CURVE('',#13914,#13916,#2497,.T.);
#17358=EDGE_CURVE('',#13915,#13917,#2498,.T.);
#17359=EDGE_CURVE('',#13917,#13916,#8711,.T.);
#17360=EDGE_CURVE('',#13916,#13902,#8712,.T.);
#17361=EDGE_CURVE('',#13917,#13904,#8713,.T.);
#17362=EDGE_CURVE('',#13918,#13919,#8714,.T.);
#17363=EDGE_CURVE('',#13919,#13920,#8715,.T.);
#17364=EDGE_CURVE('',#13921,#13920,#8716,.T.);
#17365=EDGE_CURVE('',#13918,#13921,#8717,.T.);
#17366=EDGE_CURVE('',#13922,#13922,#2499,.T.);
#17367=EDGE_CURVE('',#13923,#13923,#2500,.T.);
#17368=EDGE_CURVE('',#13924,#13925,#8718,.T.);
#17369=EDGE_CURVE('',#13925,#13926,#2501,.T.);
#17370=EDGE_CURVE('',#13926,#13927,#8719,.T.);
#17371=EDGE_CURVE('',#13927,#13928,#2502,.T.);
#17372=EDGE_CURVE('',#13928,#13929,#8720,.T.);
#17373=EDGE_CURVE('',#13929,#13930,#2503,.T.);
#17374=EDGE_CURVE('',#13930,#13931,#8721,.T.);
#17375=EDGE_CURVE('',#13931,#13924,#2504,.T.);
#17376=EDGE_CURVE('',#13932,#13925,#8722,.T.);
#17377=EDGE_CURVE('',#13932,#13933,#2505,.T.);
#17378=EDGE_CURVE('',#13933,#13926,#8723,.T.);
#17379=EDGE_CURVE('',#13933,#13934,#8724,.T.);
#17380=EDGE_CURVE('',#13934,#13927,#8725,.T.);
#17381=EDGE_CURVE('',#13934,#13935,#2506,.T.);
#17382=EDGE_CURVE('',#13935,#13928,#8726,.T.);
#17383=EDGE_CURVE('',#13935,#13936,#8727,.T.);
#17384=EDGE_CURVE('',#13936,#13929,#8728,.T.);
#17385=EDGE_CURVE('',#13936,#13937,#2507,.T.);
#17386=EDGE_CURVE('',#13937,#13930,#8729,.T.);
#17387=EDGE_CURVE('',#13937,#13938,#8730,.T.);
#17388=EDGE_CURVE('',#13938,#13931,#8731,.T.);
#17389=EDGE_CURVE('',#13938,#13939,#2508,.T.);
#17390=EDGE_CURVE('',#13939,#13924,#8732,.T.);
#17391=EDGE_CURVE('',#13939,#13932,#8733,.T.);
#17392=EDGE_CURVE('',#13940,#13940,#2509,.T.);
#17393=EDGE_CURVE('',#13941,#13942,#2510,.T.);
#17394=EDGE_CURVE('',#13942,#13943,#2511,.T.);
#17395=EDGE_CURVE('',#13943,#13944,#2512,.T.);
#17396=EDGE_CURVE('',#13944,#13945,#2513,.T.);
#17397=EDGE_CURVE('',#13945,#13946,#2514,.T.);
#17398=EDGE_CURVE('',#13946,#13947,#2515,.T.);
#17399=EDGE_CURVE('',#13947,#13948,#2516,.T.);
#17400=EDGE_CURVE('',#13948,#13949,#2517,.T.);
#17401=EDGE_CURVE('',#13949,#13950,#2518,.T.);
#17402=EDGE_CURVE('',#13950,#13951,#2519,.T.);
#17403=EDGE_CURVE('',#13951,#13952,#2520,.T.);
#17404=EDGE_CURVE('',#13952,#13941,#2521,.T.);
#17405=EDGE_CURVE('',#13940,#13923,#8734,.T.);
#17406=EDGE_CURVE('',#13953,#13953,#2522,.T.);
#17407=EDGE_CURVE('',#13954,#13955,#2523,.T.);
#17408=EDGE_CURVE('',#13955,#13956,#2524,.T.);
#17409=EDGE_CURVE('',#13956,#13957,#2525,.T.);
#17410=EDGE_CURVE('',#13957,#13958,#2526,.T.);
#17411=EDGE_CURVE('',#13958,#13959,#2527,.T.);
#17412=EDGE_CURVE('',#13959,#13960,#2528,.T.);
#17413=EDGE_CURVE('',#13960,#13961,#2529,.T.);
#17414=EDGE_CURVE('',#13961,#13962,#2530,.T.);
#17415=EDGE_CURVE('',#13962,#13963,#2531,.T.);
#17416=EDGE_CURVE('',#13963,#13964,#2532,.T.);
#17417=EDGE_CURVE('',#13964,#13965,#2533,.T.);
#17418=EDGE_CURVE('',#13965,#13954,#2534,.T.);
#17419=EDGE_CURVE('',#13953,#13922,#8735,.T.);
#17420=EDGE_CURVE('',#13966,#13964,#8736,.T.);
#17421=EDGE_CURVE('',#13966,#13967,#8737,.T.);
#17422=EDGE_CURVE('',#13967,#13965,#8738,.T.);
#17423=EDGE_CURVE('',#13967,#13968,#8739,.T.);
#17424=EDGE_CURVE('',#13968,#13954,#8740,.T.);
#17425=EDGE_CURVE('',#13968,#13969,#8741,.T.);
#17426=EDGE_CURVE('',#13969,#13955,#8742,.T.);
#17427=EDGE_CURVE('',#13969,#13970,#8743,.T.);
#17428=EDGE_CURVE('',#13970,#13956,#8744,.T.);
#17429=EDGE_CURVE('',#13970,#13971,#8745,.T.);
#17430=EDGE_CURVE('',#13971,#13957,#8746,.T.);
#17431=EDGE_CURVE('',#13971,#13972,#8747,.T.);
#17432=EDGE_CURVE('',#13972,#13958,#8748,.T.);
#17433=EDGE_CURVE('',#13972,#13973,#8749,.T.);
#17434=EDGE_CURVE('',#13973,#13959,#8750,.T.);
#17435=EDGE_CURVE('',#13973,#13974,#8751,.T.);
#17436=EDGE_CURVE('',#13974,#13960,#8752,.T.);
#17437=EDGE_CURVE('',#13974,#13975,#8753,.T.);
#17438=EDGE_CURVE('',#13975,#13961,#8754,.T.);
#17439=EDGE_CURVE('',#13975,#13976,#8755,.T.);
#17440=EDGE_CURVE('',#13976,#13962,#8756,.T.);
#17441=EDGE_CURVE('',#13976,#13977,#8757,.T.);
#17442=EDGE_CURVE('',#13977,#13963,#8758,.T.);
#17443=EDGE_CURVE('',#13977,#13966,#8759,.T.);
#17444=EDGE_CURVE('',#13978,#13951,#8760,.T.);
#17445=EDGE_CURVE('',#13978,#13979,#8761,.T.);
#17446=EDGE_CURVE('',#13979,#13952,#8762,.T.);
#17447=EDGE_CURVE('',#13979,#13980,#8763,.T.);
#17448=EDGE_CURVE('',#13980,#13941,#8764,.T.);
#17449=EDGE_CURVE('',#13980,#13981,#8765,.T.);
#17450=EDGE_CURVE('',#13981,#13942,#8766,.T.);
#17451=EDGE_CURVE('',#13981,#13982,#8767,.T.);
#17452=EDGE_CURVE('',#13982,#13943,#8768,.T.);
#17453=EDGE_CURVE('',#13982,#13983,#8769,.T.);
#17454=EDGE_CURVE('',#13983,#13944,#8770,.T.);
#17455=EDGE_CURVE('',#13983,#13984,#8771,.T.);
#17456=EDGE_CURVE('',#13984,#13945,#8772,.T.);
#17457=EDGE_CURVE('',#13984,#13985,#8773,.T.);
#17458=EDGE_CURVE('',#13985,#13946,#8774,.T.);
#17459=EDGE_CURVE('',#13985,#13986,#8775,.T.);
#17460=EDGE_CURVE('',#13986,#13947,#8776,.T.);
#17461=EDGE_CURVE('',#13986,#13987,#8777,.T.);
#17462=EDGE_CURVE('',#13987,#13948,#8778,.T.);
#17463=EDGE_CURVE('',#13987,#13988,#8779,.T.);
#17464=EDGE_CURVE('',#13988,#13949,#8780,.T.);
#17465=EDGE_CURVE('',#13988,#13989,#8781,.T.);
#17466=EDGE_CURVE('',#13989,#13950,#8782,.T.);
#17467=EDGE_CURVE('',#13989,#13978,#8783,.T.);
#17468=EDGE_CURVE('',#13811,#13990,#8784,.T.);
#17469=EDGE_CURVE('',#13990,#13991,#8785,.T.);
#17470=EDGE_CURVE('',#13991,#13992,#8786,.T.);
#17471=EDGE_CURVE('',#13992,#13993,#8787,.T.);
#17472=EDGE_CURVE('',#13993,#13994,#8788,.T.);
#17473=EDGE_CURVE('',#13994,#13995,#8789,.T.);
#17474=EDGE_CURVE('',#13995,#13996,#8790,.T.);
#17475=EDGE_CURVE('',#13996,#13997,#8791,.T.);
#17476=EDGE_CURVE('',#13997,#13814,#8792,.T.);
#17477=EDGE_CURVE('',#13997,#13805,#8793,.T.);
#17478=EDGE_CURVE('',#13996,#13806,#8794,.T.);
#17479=EDGE_CURVE('',#13995,#13807,#8795,.T.);
#17480=EDGE_CURVE('',#13994,#13808,#8796,.T.);
#17481=EDGE_CURVE('',#13993,#13809,#8797,.T.);
#17482=EDGE_CURVE('',#13992,#13810,#8798,.T.);
#17483=EDGE_CURVE('',#13991,#13796,#8799,.T.);
#17484=EDGE_CURVE('',#13990,#13800,#8800,.T.);
#17485=EDGE_CURVE('',#13998,#13999,#809,.T.);
#17486=EDGE_CURVE('',#13826,#13998,#8801,.T.);
#17487=EDGE_CURVE('',#13999,#13825,#8802,.T.);
#17488=EDGE_CURVE('',#14000,#13824,#8803,.T.);
#17489=EDGE_CURVE('',#13999,#14000,#8804,.T.);
#17490=EDGE_CURVE('',#14000,#13831,#2535,.T.);
#17491=EDGE_CURVE('',#13832,#13843,#2536,.T.);
#17492=EDGE_CURVE('',#14001,#13851,#8805,.T.);
#17493=EDGE_CURVE('',#14002,#14001,#810,.T.);
#17494=EDGE_CURVE('',#13852,#14002,#8806,.T.);
#17495=EDGE_CURVE('',#13819,#13918,#8807,.T.);
#17496=EDGE_CURVE('',#13921,#13853,#8808,.T.);
#17497=EDGE_CURVE('',#13901,#14002,#2537,.T.);
#17498=EDGE_CURVE('',#13838,#13998,#2538,.T.);
#17499=EDGE_CURVE('',#13920,#13849,#8809,.T.);
#17500=EDGE_CURVE('',#13827,#13919,#8810,.T.);
#17501=EDGE_CURVE('',#13835,#13841,#2539,.T.);
#17502=EDGE_CURVE('',#14003,#13836,#2540,.T.);
#17503=EDGE_CURVE('',#14003,#13850,#8811,.T.);
#17504=EDGE_CURVE('',#14001,#14003,#8812,.T.);
#17505=EDGE_CURVE('',#14004,#14004,#2541,.T.);
#17506=EDGE_CURVE('',#14005,#13867,#8813,.T.);
#17507=EDGE_CURVE('',#14006,#14005,#8814,.T.);
#17508=EDGE_CURVE('',#14006,#13868,#8815,.T.);
#17509=EDGE_CURVE('',#14007,#14006,#8816,.T.);
#17510=EDGE_CURVE('',#14007,#13857,#8817,.T.);
#17511=EDGE_CURVE('',#14008,#13866,#8818,.T.);
#17512=EDGE_CURVE('',#14005,#14008,#8819,.T.);
#17513=EDGE_CURVE('',#14009,#14007,#8820,.T.);
#17514=EDGE_CURVE('',#14009,#13858,#8821,.T.);
#17515=EDGE_CURVE('',#14010,#14009,#8822,.T.);
#17516=EDGE_CURVE('',#14010,#13859,#8823,.T.);
#17517=EDGE_CURVE('',#14011,#14010,#8824,.T.);
#17518=EDGE_CURVE('',#14011,#13860,#8825,.T.);
#17519=EDGE_CURVE('',#14012,#14011,#8826,.T.);
#17520=EDGE_CURVE('',#14012,#13861,#8827,.T.);
#17521=EDGE_CURVE('',#14013,#14012,#8828,.T.);
#17522=EDGE_CURVE('',#14013,#13862,#8829,.T.);
#17523=EDGE_CURVE('',#14014,#14013,#8830,.T.);
#17524=EDGE_CURVE('',#14014,#13863,#8831,.T.);
#17525=EDGE_CURVE('',#14015,#14014,#8832,.T.);
#17526=EDGE_CURVE('',#14015,#13864,#8833,.T.);
#17527=EDGE_CURVE('',#14016,#14015,#8834,.T.);
#17528=EDGE_CURVE('',#14016,#13865,#8835,.T.);
#17529=EDGE_CURVE('',#14004,#14017,#8836,.T.);
#17530=EDGE_CURVE('',#14017,#14017,#2542,.T.);
#17531=EDGE_CURVE('',#14008,#14016,#8837,.T.);
#17532=EDGE_CURVE('',#13870,#14018,#2543,.T.);
#17533=EDGE_CURVE('',#14018,#14019,#2544,.T.);
#17534=EDGE_CURVE('',#14019,#14020,#2545,.T.);
#17535=EDGE_CURVE('',#14020,#14021,#2546,.T.);
#17536=EDGE_CURVE('',#14021,#14022,#2547,.T.);
#17537=EDGE_CURVE('',#14022,#14023,#2548,.T.);
#17538=EDGE_CURVE('',#14023,#14024,#2549,.T.);
#17539=EDGE_CURVE('',#14024,#14025,#2550,.T.);
#17540=EDGE_CURVE('',#14025,#14026,#2551,.T.);
#17541=EDGE_CURVE('',#14026,#13873,#2552,.T.);
#17542=EDGE_CURVE('',#13874,#14027,#8838,.T.);
#17543=EDGE_CURVE('',#14027,#14028,#8839,.T.);
#17544=EDGE_CURVE('',#14028,#14029,#8840,.T.);
#17545=EDGE_CURVE('',#14029,#14030,#8841,.T.);
#17546=EDGE_CURVE('',#14030,#14031,#8842,.T.);
#17547=EDGE_CURVE('',#14031,#14032,#8843,.T.);
#17548=EDGE_CURVE('',#14032,#14033,#8844,.T.);
#17549=EDGE_CURVE('',#14033,#14034,#8845,.T.);
#17550=EDGE_CURVE('',#14034,#14035,#8846,.T.);
#17551=EDGE_CURVE('',#14035,#13872,#8847,.T.);
#17552=EDGE_CURVE('',#14035,#14018,#8848,.T.);
#17553=EDGE_CURVE('',#14034,#14019,#8849,.T.);
#17554=EDGE_CURVE('',#14033,#14020,#8850,.T.);
#17555=EDGE_CURVE('',#14032,#14021,#8851,.T.);
#17556=EDGE_CURVE('',#14031,#14022,#8852,.T.);
#17557=EDGE_CURVE('',#14030,#14023,#8853,.T.);
#17558=EDGE_CURVE('',#14029,#14024,#8854,.T.);
#17559=EDGE_CURVE('',#14028,#14025,#8855,.T.);
#17560=EDGE_CURVE('',#14027,#14026,#8856,.T.);
#17561=EDGE_CURVE('',#14036,#14036,#2553,.T.);
#17562=EDGE_CURVE('',#14037,#14037,#2554,.T.);
#17563=EDGE_CURVE('',#14038,#14039,#811,.T.);
#17564=EDGE_CURVE('',#14039,#14040,#8857,.T.);
#17565=EDGE_CURVE('',#14041,#14040,#2555,.T.);
#17566=EDGE_CURVE('',#14040,#14041,#2556,.T.);
#17567=EDGE_CURVE('',#14039,#14038,#812,.T.);
#17568=EDGE_CURVE('',#14042,#14043,#2557,.T.);
#17569=EDGE_CURVE('',#14043,#14042,#2558,.T.);
#17570=EDGE_CURVE('',#14044,#14045,#813,.T.);
#17571=EDGE_CURVE('',#14045,#14046,#8858,.T.);
#17572=EDGE_CURVE('',#14047,#14046,#2559,.T.);
#17573=EDGE_CURVE('',#14046,#14047,#2560,.T.);
#17574=EDGE_CURVE('',#14045,#14044,#814,.T.);
#17575=EDGE_CURVE('',#14048,#14049,#2561,.T.);
#17576=EDGE_CURVE('',#14050,#14048,#510,.T.);
#17577=EDGE_CURVE('',#14049,#14050,#2562,.T.);
#17578=EDGE_CURVE('',#14051,#14052,#815,.T.);
#17579=EDGE_CURVE('',#14052,#14053,#8859,.T.);
#17580=EDGE_CURVE('',#14053,#14053,#2563,.T.);
#17581=EDGE_CURVE('',#14052,#14051,#816,.T.);
#17582=EDGE_CURVE('',#14049,#14053,#2564,.T.);
#17583=EDGE_CURVE('',#14054,#14055,#2565,.T.);
#17584=EDGE_CURVE('',#14055,#14054,#2566,.T.);
#17585=EDGE_CURVE('',#14055,#14041,#2567,.T.);
#17586=EDGE_CURVE('',#14043,#14047,#2568,.T.);
#17587=EDGE_CURVE('',#14056,#14057,#2569,.T.);
#17588=EDGE_CURVE('',#14057,#14056,#2570,.T.);
#17589=EDGE_CURVE('',#14057,#14058,#2571,.T.);
#17590=EDGE_CURVE('',#14058,#14058,#2572,.T.);
#17591=EDGE_CURVE('',#14056,#14036,#8860,.T.);
#17592=EDGE_CURVE('',#14059,#14059,#2573,.T.);
#17593=EDGE_CURVE('',#14037,#14060,#8861,.T.);
#17594=EDGE_CURVE('',#14061,#14060,#2574,.T.);
#17595=EDGE_CURVE('',#14060,#14061,#2575,.T.);
#17596=EDGE_CURVE('',#14062,#14063,#2576,.T.);
#17597=EDGE_CURVE('',#14064,#14063,#8862,.T.);
#17598=EDGE_CURVE('',#14065,#14064,#8863,.T.);
#17599=EDGE_CURVE('',#14065,#14062,#8864,.T.);
#17600=EDGE_CURVE('',#14064,#14066,#8865,.T.);
#17601=EDGE_CURVE('',#14066,#14067,#8866,.T.);
#17602=EDGE_CURVE('',#14067,#14068,#8867,.T.);
#17603=EDGE_CURVE('',#14068,#14069,#8868,.T.);
#17604=EDGE_CURVE('',#14069,#14070,#8869,.T.);
#17605=EDGE_CURVE('',#14070,#14071,#8870,.T.);
#17606=EDGE_CURVE('',#14071,#14072,#8871,.T.);
#17607=EDGE_CURVE('',#14072,#14073,#8872,.T.);
#17608=EDGE_CURVE('',#14073,#14074,#8873,.T.);
#17609=EDGE_CURVE('',#14074,#14075,#8874,.T.);
#17610=EDGE_CURVE('',#14075,#14076,#8875,.T.);
#17611=EDGE_CURVE('',#14076,#14077,#8876,.T.);
#17612=EDGE_CURVE('',#14077,#14078,#8877,.T.);
#17613=EDGE_CURVE('',#14078,#14079,#8878,.T.);
#17614=EDGE_CURVE('',#14079,#14065,#8879,.T.);
#17615=EDGE_CURVE('',#14080,#14062,#2577,.T.);
#17616=EDGE_CURVE('',#14079,#14080,#8880,.T.);
#17617=EDGE_CURVE('',#14081,#14082,#8881,.T.);
#17618=EDGE_CURVE('',#14081,#14083,#8882,.T.);
#17619=EDGE_CURVE('',#14083,#14084,#8883,.T.);
#17620=EDGE_CURVE('',#14085,#14084,#8884,.T.);
#17621=EDGE_CURVE('',#14085,#14086,#8885,.T.);
#17622=EDGE_CURVE('',#14082,#14086,#8886,.T.);
#17623=EDGE_CURVE('',#14087,#14088,#8887,.T.);
#17624=EDGE_CURVE('',#14088,#14089,#8888,.T.);
#17625=EDGE_CURVE('',#14089,#14090,#8889,.T.);
#17626=EDGE_CURVE('',#14091,#14090,#8890,.T.);
#17627=EDGE_CURVE('',#14092,#14091,#8891,.T.);
#17628=EDGE_CURVE('',#14087,#14092,#8892,.T.);
#17629=EDGE_CURVE('',#14093,#14094,#8893,.T.);
#17630=EDGE_CURVE('',#14094,#14095,#2578,.T.);
#17631=EDGE_CURVE('',#14095,#14096,#8894,.T.);
#17632=EDGE_CURVE('',#14096,#14093,#2579,.T.);
#17633=EDGE_CURVE('',#14097,#14098,#2580,.T.);
#17634=EDGE_CURVE('',#14097,#14099,#8895,.T.);
#17635=EDGE_CURVE('',#14099,#14100,#2581,.T.);
#17636=EDGE_CURVE('',#14100,#14098,#8896,.T.);
#17637=EDGE_CURVE('',#14101,#14102,#2582,.T.);
#17638=EDGE_CURVE('',#14093,#14101,#8897,.T.);
#17639=EDGE_CURVE('',#14096,#14102,#8898,.T.);
#17640=EDGE_CURVE('',#14102,#14103,#8899,.T.);
#17641=EDGE_CURVE('',#14095,#14103,#8900,.T.);
#17642=EDGE_CURVE('',#14103,#14104,#2583,.T.);
#17643=EDGE_CURVE('',#14094,#14104,#8901,.T.);
#17644=EDGE_CURVE('',#14104,#14101,#8902,.T.);
#17645=EDGE_CURVE('',#14105,#14106,#8903,.T.);
#17646=EDGE_CURVE('',#14106,#14107,#2584,.T.);
#17647=EDGE_CURVE('',#14107,#14108,#8904,.T.);
#17648=EDGE_CURVE('',#14108,#14105,#2585,.T.);
#17649=EDGE_CURVE('',#14087,#14084,#2586,.T.);
#17650=EDGE_CURVE('',#14092,#14085,#2587,.T.);
#17651=EDGE_CURVE('',#14109,#14110,#2588,.T.);
#17652=EDGE_CURVE('',#14105,#14109,#8905,.T.);
#17653=EDGE_CURVE('',#14108,#14110,#8906,.T.);
#17654=EDGE_CURVE('',#14110,#14111,#8907,.T.);
#17655=EDGE_CURVE('',#14107,#14111,#8908,.T.);
#17656=EDGE_CURVE('',#14111,#14112,#2589,.T.);
#17657=EDGE_CURVE('',#14106,#14112,#8909,.T.);
#17658=EDGE_CURVE('',#14112,#14109,#8910,.T.);
#17659=EDGE_CURVE('',#14113,#14113,#2590,.T.);
#17660=EDGE_CURVE('',#14113,#14114,#8911,.T.);
#17661=EDGE_CURVE('',#14115,#14114,#2591,.T.);
#17662=EDGE_CURVE('',#14114,#14115,#2592,.T.);
#17663=EDGE_CURVE('',#14115,#14116,#8912,.T.);
#17664=EDGE_CURVE('',#14116,#14116,#2593,.T.);
#17665=EDGE_CURVE('',#14117,#14117,#2594,.T.);
#17666=EDGE_CURVE('',#14117,#14118,#8913,.T.);
#17667=EDGE_CURVE('',#14119,#14118,#2595,.T.);
#17668=EDGE_CURVE('',#14118,#14119,#2596,.T.);
#17669=EDGE_CURVE('',#14119,#14120,#8914,.T.);
#17670=EDGE_CURVE('',#14120,#14120,#2597,.T.);
#17671=EDGE_CURVE('',#14121,#14121,#2598,.T.);
#17672=EDGE_CURVE('',#14121,#14122,#8915,.T.);
#17673=EDGE_CURVE('',#14123,#14122,#2599,.T.);
#17674=EDGE_CURVE('',#14122,#14123,#2600,.T.);
#17675=EDGE_CURVE('',#14123,#14124,#8916,.T.);
#17676=EDGE_CURVE('',#14124,#14124,#2601,.T.);
#17677=EDGE_CURVE('',#14125,#14125,#2602,.T.);
#17678=EDGE_CURVE('',#14125,#14126,#8917,.T.);
#17679=EDGE_CURVE('',#14127,#14126,#2603,.T.);
#17680=EDGE_CURVE('',#14126,#14127,#2604,.T.);
#17681=EDGE_CURVE('',#14127,#14128,#8918,.T.);
#17682=EDGE_CURVE('',#14128,#14128,#2605,.T.);
#17683=EDGE_CURVE('',#14061,#14129,#8919,.T.);
#17684=EDGE_CURVE('',#14129,#14129,#2606,.T.);
#17685=EDGE_CURVE('',#14130,#14130,#2607,.T.);
#17686=EDGE_CURVE('',#14131,#14131,#2608,.T.);
#17687=EDGE_CURVE('',#14132,#14132,#2609,.T.);
#17688=EDGE_CURVE('',#14133,#14133,#2610,.T.);
#17689=EDGE_CURVE('',#14134,#14134,#2611,.T.);
#17690=EDGE_CURVE('',#14134,#14135,#8920,.T.);
#17691=EDGE_CURVE('',#14135,#14135,#2612,.T.);
#17692=EDGE_CURVE('',#14136,#14136,#2613,.T.);
#17693=EDGE_CURVE('',#14136,#14137,#8921,.T.);
#17694=EDGE_CURVE('',#14137,#14137,#2614,.T.);
#17695=EDGE_CURVE('',#14138,#14138,#2615,.T.);
#17696=EDGE_CURVE('',#14138,#14139,#8922,.T.);
#17697=EDGE_CURVE('',#14139,#14139,#2616,.T.);
#17698=EDGE_CURVE('',#14140,#14140,#2617,.T.);
#17699=EDGE_CURVE('',#14140,#14059,#8923,.T.);
#17700=EDGE_CURVE('',#14141,#14141,#2618,.T.);
#17701=EDGE_CURVE('',#14142,#14142,#2619,.T.);
#17702=EDGE_CURVE('',#14130,#14141,#8924,.T.);
#17703=EDGE_CURVE('',#14142,#14143,#8925,.T.);
#17704=EDGE_CURVE('',#14143,#14143,#2620,.T.);
#17705=EDGE_CURVE('',#14144,#14144,#2621,.T.);
#17706=EDGE_CURVE('',#14144,#14133,#8926,.T.);
#17707=EDGE_CURVE('',#14145,#14145,#2622,.T.);
#17708=EDGE_CURVE('',#14146,#14146,#2623,.T.);
#17709=EDGE_CURVE('',#14146,#14145,#8927,.T.);
#17710=EDGE_CURVE('',#14147,#14147,#2624,.T.);
#17711=EDGE_CURVE('',#14148,#14148,#2625,.T.);
#17712=EDGE_CURVE('',#14148,#14147,#8928,.T.);
#17713=EDGE_CURVE('',#14149,#14149,#2626,.T.);
#17714=EDGE_CURVE('',#14132,#14149,#8929,.T.);
#17715=EDGE_CURVE('',#14150,#14150,#2627,.T.);
#17716=EDGE_CURVE('',#14150,#14131,#8930,.T.);
#17717=EDGE_CURVE('',#14151,#14151,#2628,.T.);
#17718=EDGE_CURVE('',#14152,#14152,#2629,.T.);
#17719=EDGE_CURVE('',#14152,#14151,#8931,.T.);
#17720=EDGE_CURVE('',#14153,#14154,#8932,.T.);
#17721=EDGE_CURVE('',#14153,#14155,#8933,.T.);
#17722=EDGE_CURVE('',#14155,#14098,#8934,.T.);
#17723=EDGE_CURVE('',#14100,#14156,#8935,.T.);
#17724=EDGE_CURVE('',#14154,#14156,#8936,.T.);
#17725=EDGE_CURVE('',#14157,#14158,#8937,.T.);
#17726=EDGE_CURVE('',#14157,#14153,#2630,.T.);
#17727=EDGE_CURVE('',#14158,#14154,#2631,.T.);
#17728=EDGE_CURVE('',#14097,#14159,#8938,.T.);
#17729=EDGE_CURVE('',#14159,#14157,#8939,.T.);
#17730=EDGE_CURVE('',#14160,#14158,#8940,.T.);
#17731=EDGE_CURVE('',#14099,#14160,#8941,.T.);
#17732=EDGE_CURVE('',#14086,#14091,#2632,.T.);
#17733=EDGE_CURVE('',#14090,#14082,#2633,.T.);
#17734=EDGE_CURVE('',#14161,#14161,#2634,.T.);
#17735=EDGE_CURVE('',#14089,#14081,#2635,.T.);
#17736=EDGE_CURVE('',#14156,#14160,#2636,.T.);
#17737=EDGE_CURVE('',#14162,#14162,#2637,.T.);
#17738=EDGE_CURVE('',#14098,#14097,#2638,.T.);
#17739=EDGE_CURVE('',#14155,#14159,#2639,.T.);
#17740=EDGE_CURVE('',#14162,#14163,#8942,.T.);
#17741=EDGE_CURVE('',#14163,#14163,#2640,.T.);
#17742=EDGE_CURVE('',#14164,#14165,#2641,.T.);
#17743=EDGE_CURVE('',#14166,#14164,#2642,.T.);
#17744=EDGE_CURVE('',#14167,#14166,#2643,.T.);
#17745=EDGE_CURVE('',#14168,#14167,#2644,.T.);
#17746=EDGE_CURVE('',#14169,#14168,#2645,.T.);
#17747=EDGE_CURVE('',#14170,#14169,#2646,.T.);
#17748=EDGE_CURVE('',#14171,#14170,#2647,.T.);
#17749=EDGE_CURVE('',#14172,#14171,#2648,.T.);
#17750=EDGE_CURVE('',#14063,#14172,#2649,.T.);
#17751=EDGE_CURVE('',#14173,#14080,#2650,.T.);
#17752=EDGE_CURVE('',#14174,#14173,#2651,.T.);
#17753=EDGE_CURVE('',#14175,#14174,#2652,.T.);
#17754=EDGE_CURVE('',#14176,#14175,#2653,.T.);
#17755=EDGE_CURVE('',#14165,#14176,#2654,.T.);
#17756=EDGE_CURVE('',#14083,#14088,#2655,.T.);
#17757=EDGE_CURVE('',#14177,#14177,#2656,.T.);
#17758=EDGE_CURVE('',#14161,#14177,#8943,.T.);
#17759=EDGE_CURVE('',#14084,#14087,#2657,.T.);
#17760=EDGE_CURVE('',#14178,#14179,#2658,.T.);
#17761=EDGE_CURVE('',#14180,#14178,#2659,.T.);
#17762=EDGE_CURVE('',#14181,#14180,#2660,.T.);
#17763=EDGE_CURVE('',#14182,#14181,#2661,.T.);
#17764=EDGE_CURVE('',#14183,#14182,#2662,.T.);
#17765=EDGE_CURVE('',#14184,#14183,#2663,.T.);
#17766=EDGE_CURVE('',#14185,#14184,#2664,.T.);
#17767=EDGE_CURVE('',#14186,#14185,#2665,.T.);
#17768=EDGE_CURVE('',#14187,#14186,#2666,.T.);
#17769=EDGE_CURVE('',#14188,#14187,#2667,.T.);
#17770=EDGE_CURVE('',#14189,#14188,#2668,.T.);
#17771=EDGE_CURVE('',#14190,#14189,#2669,.T.);
#17772=EDGE_CURVE('',#14191,#14190,#2670,.T.);
#17773=EDGE_CURVE('',#14192,#14191,#2671,.T.);
#17774=EDGE_CURVE('',#14193,#14192,#2672,.T.);
#17775=EDGE_CURVE('',#14179,#14193,#2673,.T.);
#17776=EDGE_CURVE('',#14194,#14187,#8944,.T.);
#17777=EDGE_CURVE('',#14195,#14194,#8945,.T.);
#17778=EDGE_CURVE('',#14195,#14188,#8946,.T.);
#17779=EDGE_CURVE('',#14196,#14186,#8947,.T.);
#17780=EDGE_CURVE('',#14194,#14196,#8948,.T.);
#17781=EDGE_CURVE('',#14197,#14185,#8949,.T.);
#17782=EDGE_CURVE('',#14196,#14197,#8950,.T.);
#17783=EDGE_CURVE('',#14198,#14184,#8951,.T.);
#17784=EDGE_CURVE('',#14197,#14198,#8952,.T.);
#17785=EDGE_CURVE('',#14199,#14183,#8953,.T.);
#17786=EDGE_CURVE('',#14198,#14199,#8954,.T.);
#17787=EDGE_CURVE('',#14200,#14182,#8955,.T.);
#17788=EDGE_CURVE('',#14199,#14200,#8956,.T.);
#17789=EDGE_CURVE('',#14201,#14181,#8957,.T.);
#17790=EDGE_CURVE('',#14200,#14201,#8958,.T.);
#17791=EDGE_CURVE('',#14202,#14180,#8959,.T.);
#17792=EDGE_CURVE('',#14201,#14202,#8960,.T.);
#17793=EDGE_CURVE('',#14203,#14178,#8961,.T.);
#17794=EDGE_CURVE('',#14202,#14203,#8962,.T.);
#17795=EDGE_CURVE('',#14204,#14179,#8963,.T.);
#17796=EDGE_CURVE('',#14203,#14204,#8964,.T.);
#17797=EDGE_CURVE('',#14205,#14193,#8965,.T.);
#17798=EDGE_CURVE('',#14204,#14205,#8966,.T.);
#17799=EDGE_CURVE('',#14206,#14192,#8967,.T.);
#17800=EDGE_CURVE('',#14205,#14206,#8968,.T.);
#17801=EDGE_CURVE('',#14207,#14191,#8969,.T.);
#17802=EDGE_CURVE('',#14206,#14207,#8970,.T.);
#17803=EDGE_CURVE('',#14208,#14190,#8971,.T.);
#17804=EDGE_CURVE('',#14207,#14208,#8972,.T.);
#17805=EDGE_CURVE('',#14209,#14189,#8973,.T.);
#17806=EDGE_CURVE('',#14208,#14209,#8974,.T.);
#17807=EDGE_CURVE('',#14209,#14195,#8975,.T.);
#17808=EDGE_CURVE('',#14066,#14172,#8976,.T.);
#17809=EDGE_CURVE('',#14067,#14171,#8977,.T.);
#17810=EDGE_CURVE('',#14068,#14170,#8978,.T.);
#17811=EDGE_CURVE('',#14069,#14169,#8979,.T.);
#17812=EDGE_CURVE('',#14070,#14168,#8980,.T.);
#17813=EDGE_CURVE('',#14071,#14167,#8981,.T.);
#17814=EDGE_CURVE('',#14072,#14166,#8982,.T.);
#17815=EDGE_CURVE('',#14073,#14164,#8983,.T.);
#17816=EDGE_CURVE('',#14074,#14165,#8984,.T.);
#17817=EDGE_CURVE('',#14075,#14176,#8985,.T.);
#17818=EDGE_CURVE('',#14076,#14175,#8986,.T.);
#17819=EDGE_CURVE('',#14077,#14174,#8987,.T.);
#17820=EDGE_CURVE('',#14078,#14173,#8988,.T.);
#22598=ORIENTED_EDGE('',*,*,#17201,.T.);
#22599=ORIENTED_EDGE('',*,*,#17202,.T.);
#22600=ORIENTED_EDGE('',*,*,#17203,.F.);
#22601=ORIENTED_EDGE('',*,*,#17204,.F.);
#22602=ORIENTED_EDGE('',*,*,#17202,.F.);
#22603=ORIENTED_EDGE('',*,*,#17205,.T.);
#22604=ORIENTED_EDGE('',*,*,#17206,.T.);
#22605=ORIENTED_EDGE('',*,*,#17207,.T.);
#22606=ORIENTED_EDGE('',*,*,#17208,.T.);
#22607=ORIENTED_EDGE('',*,*,#17209,.T.);
#22608=ORIENTED_EDGE('',*,*,#17210,.T.);
#22609=ORIENTED_EDGE('',*,*,#17211,.T.);
#22610=ORIENTED_EDGE('',*,*,#17212,.T.);
#22611=ORIENTED_EDGE('',*,*,#17213,.T.);
#22612=ORIENTED_EDGE('',*,*,#17214,.T.);
#22613=ORIENTED_EDGE('',*,*,#17215,.T.);
#22614=ORIENTED_EDGE('',*,*,#17216,.T.);
#22615=ORIENTED_EDGE('',*,*,#17207,.F.);
#22616=ORIENTED_EDGE('',*,*,#17217,.F.);
#22617=ORIENTED_EDGE('',*,*,#17218,.F.);
#22618=ORIENTED_EDGE('',*,*,#17219,.T.);
#22619=ORIENTED_EDGE('',*,*,#17208,.F.);
#22620=ORIENTED_EDGE('',*,*,#17219,.F.);
#22621=ORIENTED_EDGE('',*,*,#17220,.F.);
#22622=ORIENTED_EDGE('',*,*,#17221,.T.);
#22623=ORIENTED_EDGE('',*,*,#17209,.F.);
#22624=ORIENTED_EDGE('',*,*,#17221,.F.);
#22625=ORIENTED_EDGE('',*,*,#17222,.F.);
#22626=ORIENTED_EDGE('',*,*,#17223,.T.);
#22627=ORIENTED_EDGE('',*,*,#17224,.T.);
#22628=ORIENTED_EDGE('',*,*,#17225,.T.);
#22629=ORIENTED_EDGE('',*,*,#17203,.T.);
#22630=ORIENTED_EDGE('',*,*,#17204,.T.);
#22631=ORIENTED_EDGE('',*,*,#17226,.T.);
#22632=ORIENTED_EDGE('',*,*,#17227,.T.);
#22633=ORIENTED_EDGE('',*,*,#17224,.F.);
#22634=ORIENTED_EDGE('',*,*,#17228,.T.);
#22635=ORIENTED_EDGE('',*,*,#17226,.F.);
#22636=ORIENTED_EDGE('',*,*,#17229,.F.);
#22637=ORIENTED_EDGE('',*,*,#17230,.T.);
#22638=ORIENTED_EDGE('',*,*,#17231,.T.);
#22639=ORIENTED_EDGE('',*,*,#17232,.T.);
#22640=ORIENTED_EDGE('',*,*,#17233,.F.);
#22641=ORIENTED_EDGE('',*,*,#17234,.T.);
#22642=ORIENTED_EDGE('',*,*,#17235,.T.);
#22643=ORIENTED_EDGE('',*,*,#17236,.T.);
#22644=ORIENTED_EDGE('',*,*,#17237,.T.);
#22645=ORIENTED_EDGE('',*,*,#17238,.F.);
#22646=ORIENTED_EDGE('',*,*,#17239,.F.);
#22647=ORIENTED_EDGE('',*,*,#17240,.F.);
#22648=ORIENTED_EDGE('',*,*,#17241,.F.);
#22649=ORIENTED_EDGE('',*,*,#17228,.F.);
#22650=ORIENTED_EDGE('',*,*,#17225,.F.);
#22651=ORIENTED_EDGE('',*,*,#17227,.F.);
#22652=ORIENTED_EDGE('',*,*,#17242,.T.);
#22653=ORIENTED_EDGE('',*,*,#17233,.T.);
#22654=ORIENTED_EDGE('',*,*,#17243,.F.);
#22655=ORIENTED_EDGE('',*,*,#17244,.F.);
#22656=ORIENTED_EDGE('',*,*,#17245,.T.);
#22657=ORIENTED_EDGE('',*,*,#17246,.F.);
#22658=ORIENTED_EDGE('',*,*,#17247,.F.);
#22659=ORIENTED_EDGE('',*,*,#17248,.T.);
#22660=ORIENTED_EDGE('',*,*,#17249,.T.);
#22661=ORIENTED_EDGE('',*,*,#17250,.F.);
#22662=ORIENTED_EDGE('',*,*,#17251,.T.);
#22663=ORIENTED_EDGE('',*,*,#17252,.F.);
#22664=ORIENTED_EDGE('',*,*,#17251,.F.);
#22665=ORIENTED_EDGE('',*,*,#17253,.F.);
#22666=ORIENTED_EDGE('',*,*,#17254,.T.);
#22667=ORIENTED_EDGE('',*,*,#17255,.F.);
#22668=ORIENTED_EDGE('',*,*,#17256,.T.);
#22669=ORIENTED_EDGE('',*,*,#17231,.F.);
#22670=ORIENTED_EDGE('',*,*,#17257,.F.);
#22671=ORIENTED_EDGE('',*,*,#17258,.F.);
#22672=ORIENTED_EDGE('',*,*,#17259,.T.);
#22673=ORIENTED_EDGE('',*,*,#17260,.T.);
#22674=ORIENTED_EDGE('',*,*,#17261,.T.);
#22675=ORIENTED_EDGE('',*,*,#17262,.F.);
#22676=ORIENTED_EDGE('',*,*,#17261,.F.);
#22677=ORIENTED_EDGE('',*,*,#17263,.T.);
#22678=ORIENTED_EDGE('',*,*,#17264,.T.);
#22679=ORIENTED_EDGE('',*,*,#17252,.T.);
#22680=ORIENTED_EDGE('',*,*,#17255,.T.);
#22681=ORIENTED_EDGE('',*,*,#17265,.T.);
#22682=ORIENTED_EDGE('',*,*,#17245,.F.);
#22683=ORIENTED_EDGE('',*,*,#17266,.T.);
#22684=ORIENTED_EDGE('',*,*,#17267,.T.);
#22685=ORIENTED_EDGE('',*,*,#17268,.T.);
#22686=ORIENTED_EDGE('',*,*,#17269,.F.);
#22687=ORIENTED_EDGE('',*,*,#17270,.T.);
#22688=ORIENTED_EDGE('',*,*,#17271,.F.);
#22689=ORIENTED_EDGE('',*,*,#17263,.F.);
#22690=ORIENTED_EDGE('',*,*,#17260,.F.);
#22691=ORIENTED_EDGE('',*,*,#17272,.F.);
#22692=ORIENTED_EDGE('',*,*,#17273,.F.);
#22693=ORIENTED_EDGE('',*,*,#17274,.F.);
#22694=ORIENTED_EDGE('',*,*,#17259,.F.);
#22695=ORIENTED_EDGE('',*,*,#17271,.T.);
#22696=ORIENTED_EDGE('',*,*,#17262,.T.);
#22697=ORIENTED_EDGE('',*,*,#17275,.T.);
#22698=ORIENTED_EDGE('',*,*,#17276,.T.);
#22699=ORIENTED_EDGE('',*,*,#17277,.T.);
#22700=ORIENTED_EDGE('',*,*,#17278,.T.);
#22701=ORIENTED_EDGE('',*,*,#17279,.T.);
#22702=ORIENTED_EDGE('',*,*,#17280,.T.);
#22703=ORIENTED_EDGE('',*,*,#17281,.T.);
#22704=ORIENTED_EDGE('',*,*,#17282,.T.);
#22705=ORIENTED_EDGE('',*,*,#17283,.T.);
#22706=ORIENTED_EDGE('',*,*,#17284,.T.);
#22707=ORIENTED_EDGE('',*,*,#17285,.T.);
#22708=ORIENTED_EDGE('',*,*,#17286,.T.);
#22709=ORIENTED_EDGE('',*,*,#17287,.F.);
#22710=ORIENTED_EDGE('',*,*,#17288,.F.);
#22711=ORIENTED_EDGE('',*,*,#17289,.F.);
#22712=ORIENTED_EDGE('',*,*,#17290,.T.);
#22713=ORIENTED_EDGE('',*,*,#17291,.F.);
#22714=ORIENTED_EDGE('',*,*,#17292,.F.);
#22715=ORIENTED_EDGE('',*,*,#17293,.F.);
#22716=ORIENTED_EDGE('',*,*,#17288,.T.);
#22717=ORIENTED_EDGE('',*,*,#17294,.T.);
#22718=ORIENTED_EDGE('',*,*,#17240,.T.);
#22719=ORIENTED_EDGE('',*,*,#17295,.T.);
#22720=ORIENTED_EDGE('',*,*,#17296,.T.);
#22721=ORIENTED_EDGE('',*,*,#17241,.T.);
#22722=ORIENTED_EDGE('',*,*,#17294,.F.);
#22723=ORIENTED_EDGE('',*,*,#17239,.T.);
#22724=ORIENTED_EDGE('',*,*,#17296,.F.);
#22725=ORIENTED_EDGE('',*,*,#17297,.T.);
#22726=ORIENTED_EDGE('',*,*,#17274,.T.);
#22727=ORIENTED_EDGE('',*,*,#17298,.T.);
#22728=ORIENTED_EDGE('',*,*,#17299,.F.);
#22729=ORIENTED_EDGE('',*,*,#17298,.F.);
#22730=ORIENTED_EDGE('',*,*,#17273,.T.);
#22731=ORIENTED_EDGE('',*,*,#17300,.F.);
#22732=ORIENTED_EDGE('',*,*,#17301,.F.);
#22733=ORIENTED_EDGE('',*,*,#17302,.F.);
#22734=ORIENTED_EDGE('',*,*,#17303,.T.);
#22735=ORIENTED_EDGE('',*,*,#17304,.F.);
#22736=ORIENTED_EDGE('',*,*,#17305,.F.);
#22737=ORIENTED_EDGE('',*,*,#17306,.F.);
#22738=ORIENTED_EDGE('',*,*,#17301,.T.);
#22739=ORIENTED_EDGE('',*,*,#17307,.F.);
#22740=ORIENTED_EDGE('',*,*,#17308,.F.);
#22741=ORIENTED_EDGE('',*,*,#17309,.F.);
#22742=ORIENTED_EDGE('',*,*,#17305,.T.);
#22743=ORIENTED_EDGE('',*,*,#17310,.F.);
#22744=ORIENTED_EDGE('',*,*,#17311,.F.);
#22745=ORIENTED_EDGE('',*,*,#17312,.F.);
#22746=ORIENTED_EDGE('',*,*,#17308,.T.);
#22747=ORIENTED_EDGE('',*,*,#17313,.F.);
#22748=ORIENTED_EDGE('',*,*,#17314,.F.);
#22749=ORIENTED_EDGE('',*,*,#17315,.F.);
#22750=ORIENTED_EDGE('',*,*,#17311,.T.);
#22751=ORIENTED_EDGE('',*,*,#17316,.F.);
#22752=ORIENTED_EDGE('',*,*,#17317,.F.);
#22753=ORIENTED_EDGE('',*,*,#17318,.F.);
#22754=ORIENTED_EDGE('',*,*,#17314,.T.);
#22755=ORIENTED_EDGE('',*,*,#17319,.F.);
#22756=ORIENTED_EDGE('',*,*,#17320,.F.);
#22757=ORIENTED_EDGE('',*,*,#17321,.F.);
#22758=ORIENTED_EDGE('',*,*,#17317,.T.);
#22759=ORIENTED_EDGE('',*,*,#17322,.F.);
#22760=ORIENTED_EDGE('',*,*,#17323,.F.);
#22761=ORIENTED_EDGE('',*,*,#17324,.F.);
#22762=ORIENTED_EDGE('',*,*,#17320,.T.);
#22763=ORIENTED_EDGE('',*,*,#17325,.F.);
#22764=ORIENTED_EDGE('',*,*,#17326,.F.);
#22765=ORIENTED_EDGE('',*,*,#17327,.F.);
#22766=ORIENTED_EDGE('',*,*,#17323,.T.);
#22767=ORIENTED_EDGE('',*,*,#17328,.F.);
#22768=ORIENTED_EDGE('',*,*,#17329,.F.);
#22769=ORIENTED_EDGE('',*,*,#17330,.F.);
#22770=ORIENTED_EDGE('',*,*,#17326,.T.);
#22771=ORIENTED_EDGE('',*,*,#17331,.F.);
#22772=ORIENTED_EDGE('',*,*,#17332,.F.);
#22773=ORIENTED_EDGE('',*,*,#17333,.F.);
#22774=ORIENTED_EDGE('',*,*,#17329,.T.);
#22775=ORIENTED_EDGE('',*,*,#17334,.F.);
#22776=ORIENTED_EDGE('',*,*,#17303,.F.);
#22777=ORIENTED_EDGE('',*,*,#17335,.F.);
#22778=ORIENTED_EDGE('',*,*,#17332,.T.);
#22779=ORIENTED_EDGE('',*,*,#17302,.T.);
#22780=ORIENTED_EDGE('',*,*,#17306,.T.);
#22781=ORIENTED_EDGE('',*,*,#17309,.T.);
#22782=ORIENTED_EDGE('',*,*,#17312,.T.);
#22783=ORIENTED_EDGE('',*,*,#17315,.T.);
#22784=ORIENTED_EDGE('',*,*,#17318,.T.);
#22785=ORIENTED_EDGE('',*,*,#17321,.T.);
#22786=ORIENTED_EDGE('',*,*,#17324,.T.);
#22787=ORIENTED_EDGE('',*,*,#17327,.T.);
#22788=ORIENTED_EDGE('',*,*,#17330,.T.);
#22789=ORIENTED_EDGE('',*,*,#17333,.T.);
#22790=ORIENTED_EDGE('',*,*,#17335,.T.);
#22791=ORIENTED_EDGE('',*,*,#17299,.T.);
#22792=ORIENTED_EDGE('',*,*,#17322,.T.);
#22793=ORIENTED_EDGE('',*,*,#17319,.T.);
#22794=ORIENTED_EDGE('',*,*,#17316,.T.);
#22795=ORIENTED_EDGE('',*,*,#17313,.T.);
#22796=ORIENTED_EDGE('',*,*,#17310,.T.);
#22797=ORIENTED_EDGE('',*,*,#17307,.T.);
#22798=ORIENTED_EDGE('',*,*,#17304,.T.);
#22799=ORIENTED_EDGE('',*,*,#17300,.T.);
#22800=ORIENTED_EDGE('',*,*,#17334,.T.);
#22801=ORIENTED_EDGE('',*,*,#17331,.T.);
#22802=ORIENTED_EDGE('',*,*,#17328,.T.);
#22803=ORIENTED_EDGE('',*,*,#17325,.T.);
#22804=ORIENTED_EDGE('',*,*,#17297,.F.);
#22805=ORIENTED_EDGE('',*,*,#17272,.T.);
#22806=ORIENTED_EDGE('',*,*,#17336,.F.);
#22807=ORIENTED_EDGE('',*,*,#17257,.T.);
#22808=ORIENTED_EDGE('',*,*,#17230,.F.);
#22809=ORIENTED_EDGE('',*,*,#17337,.T.);
#22810=ORIENTED_EDGE('',*,*,#17338,.F.);
#22811=ORIENTED_EDGE('',*,*,#17339,.F.);
#22812=ORIENTED_EDGE('',*,*,#17340,.T.);
#22813=ORIENTED_EDGE('',*,*,#17341,.T.);
#22814=ORIENTED_EDGE('',*,*,#17342,.F.);
#22815=ORIENTED_EDGE('',*,*,#17341,.F.);
#22816=ORIENTED_EDGE('',*,*,#17343,.T.);
#22817=ORIENTED_EDGE('',*,*,#17344,.T.);
#22818=ORIENTED_EDGE('',*,*,#17345,.F.);
#22819=ORIENTED_EDGE('',*,*,#17344,.F.);
#22820=ORIENTED_EDGE('',*,*,#17346,.T.);
#22821=ORIENTED_EDGE('',*,*,#17347,.T.);
#22822=ORIENTED_EDGE('',*,*,#17348,.F.);
#22823=ORIENTED_EDGE('',*,*,#17347,.F.);
#22824=ORIENTED_EDGE('',*,*,#17349,.T.);
#22825=ORIENTED_EDGE('',*,*,#17350,.T.);
#22826=ORIENTED_EDGE('',*,*,#17351,.F.);
#22827=ORIENTED_EDGE('',*,*,#17350,.F.);
#22828=ORIENTED_EDGE('',*,*,#17352,.T.);
#22829=ORIENTED_EDGE('',*,*,#17353,.T.);
#22830=ORIENTED_EDGE('',*,*,#17354,.F.);
#22831=ORIENTED_EDGE('',*,*,#17353,.F.);
#22832=ORIENTED_EDGE('',*,*,#17355,.T.);
#22833=ORIENTED_EDGE('',*,*,#17356,.T.);
#22834=ORIENTED_EDGE('',*,*,#17357,.F.);
#22835=ORIENTED_EDGE('',*,*,#17356,.F.);
#22836=ORIENTED_EDGE('',*,*,#17358,.T.);
#22837=ORIENTED_EDGE('',*,*,#17359,.T.);
#22838=ORIENTED_EDGE('',*,*,#17360,.F.);
#22839=ORIENTED_EDGE('',*,*,#17359,.F.);
#22840=ORIENTED_EDGE('',*,*,#17361,.T.);
#22841=ORIENTED_EDGE('',*,*,#17339,.T.);
#22842=ORIENTED_EDGE('',*,*,#17338,.T.);
#22843=ORIENTED_EDGE('',*,*,#17342,.T.);
#22844=ORIENTED_EDGE('',*,*,#17345,.T.);
#22845=ORIENTED_EDGE('',*,*,#17348,.T.);
#22846=ORIENTED_EDGE('',*,*,#17351,.T.);
#22847=ORIENTED_EDGE('',*,*,#17354,.T.);
#22848=ORIENTED_EDGE('',*,*,#17357,.T.);
#22849=ORIENTED_EDGE('',*,*,#17360,.T.);
#22850=ORIENTED_EDGE('',*,*,#17362,.T.);
#22851=ORIENTED_EDGE('',*,*,#17363,.T.);
#22852=ORIENTED_EDGE('',*,*,#17364,.F.);
#22853=ORIENTED_EDGE('',*,*,#17365,.F.);
#22854=ORIENTED_EDGE('',*,*,#17340,.F.);
#22855=ORIENTED_EDGE('',*,*,#17361,.F.);
#22856=ORIENTED_EDGE('',*,*,#17358,.F.);
#22857=ORIENTED_EDGE('',*,*,#17355,.F.);
#22858=ORIENTED_EDGE('',*,*,#17352,.F.);
#22859=ORIENTED_EDGE('',*,*,#17349,.F.);
#22860=ORIENTED_EDGE('',*,*,#17346,.F.);
#22861=ORIENTED_EDGE('',*,*,#17343,.F.);
#22862=ORIENTED_EDGE('',*,*,#17366,.F.);
#22863=ORIENTED_EDGE('',*,*,#17367,.F.);
#22864=ORIENTED_EDGE('',*,*,#17368,.T.);
#22865=ORIENTED_EDGE('',*,*,#17369,.T.);
#22866=ORIENTED_EDGE('',*,*,#17370,.T.);
#22867=ORIENTED_EDGE('',*,*,#17371,.T.);
#22868=ORIENTED_EDGE('',*,*,#17372,.T.);
#22869=ORIENTED_EDGE('',*,*,#17373,.T.);
#22870=ORIENTED_EDGE('',*,*,#17374,.T.);
#22871=ORIENTED_EDGE('',*,*,#17375,.T.);
#22872=ORIENTED_EDGE('',*,*,#17369,.F.);
#22873=ORIENTED_EDGE('',*,*,#17376,.F.);
#22874=ORIENTED_EDGE('',*,*,#17377,.T.);
#22875=ORIENTED_EDGE('',*,*,#17378,.T.);
#22876=ORIENTED_EDGE('',*,*,#17370,.F.);
#22877=ORIENTED_EDGE('',*,*,#17378,.F.);
#22878=ORIENTED_EDGE('',*,*,#17379,.T.);
#22879=ORIENTED_EDGE('',*,*,#17380,.T.);
#22880=ORIENTED_EDGE('',*,*,#17371,.F.);
#22881=ORIENTED_EDGE('',*,*,#17380,.F.);
#22882=ORIENTED_EDGE('',*,*,#17381,.T.);
#22883=ORIENTED_EDGE('',*,*,#17382,.T.);
#22884=ORIENTED_EDGE('',*,*,#17372,.F.);
#22885=ORIENTED_EDGE('',*,*,#17382,.F.);
#22886=ORIENTED_EDGE('',*,*,#17383,.T.);
#22887=ORIENTED_EDGE('',*,*,#17384,.T.);
#22888=ORIENTED_EDGE('',*,*,#17373,.F.);
#22889=ORIENTED_EDGE('',*,*,#17384,.F.);
#22890=ORIENTED_EDGE('',*,*,#17385,.T.);
#22891=ORIENTED_EDGE('',*,*,#17386,.T.);
#22892=ORIENTED_EDGE('',*,*,#17374,.F.);
#22893=ORIENTED_EDGE('',*,*,#17386,.F.);
#22894=ORIENTED_EDGE('',*,*,#17387,.T.);
#22895=ORIENTED_EDGE('',*,*,#17388,.T.);
#22896=ORIENTED_EDGE('',*,*,#17375,.F.);
#22897=ORIENTED_EDGE('',*,*,#17388,.F.);
#22898=ORIENTED_EDGE('',*,*,#17389,.T.);
#22899=ORIENTED_EDGE('',*,*,#17390,.T.);
#22900=ORIENTED_EDGE('',*,*,#17368,.F.);
#22901=ORIENTED_EDGE('',*,*,#17390,.F.);
#22902=ORIENTED_EDGE('',*,*,#17391,.T.);
#22903=ORIENTED_EDGE('',*,*,#17376,.T.);
#22904=ORIENTED_EDGE('',*,*,#17377,.F.);
#22905=ORIENTED_EDGE('',*,*,#17391,.F.);
#22906=ORIENTED_EDGE('',*,*,#17389,.F.);
#22907=ORIENTED_EDGE('',*,*,#17387,.F.);
#22908=ORIENTED_EDGE('',*,*,#17385,.F.);
#22909=ORIENTED_EDGE('',*,*,#17383,.F.);
#22910=ORIENTED_EDGE('',*,*,#17381,.F.);
#22911=ORIENTED_EDGE('',*,*,#17379,.F.);
#22912=ORIENTED_EDGE('',*,*,#17392,.F.);
#22913=ORIENTED_EDGE('',*,*,#17393,.T.);
#22914=ORIENTED_EDGE('',*,*,#17394,.T.);
#22915=ORIENTED_EDGE('',*,*,#17395,.T.);
#22916=ORIENTED_EDGE('',*,*,#17396,.T.);
#22917=ORIENTED_EDGE('',*,*,#17397,.T.);
#22918=ORIENTED_EDGE('',*,*,#17398,.T.);
#22919=ORIENTED_EDGE('',*,*,#17399,.T.);
#22920=ORIENTED_EDGE('',*,*,#17400,.T.);
#22921=ORIENTED_EDGE('',*,*,#17401,.T.);
#22922=ORIENTED_EDGE('',*,*,#17402,.T.);
#22923=ORIENTED_EDGE('',*,*,#17403,.T.);
#22924=ORIENTED_EDGE('',*,*,#17404,.T.);
#22925=ORIENTED_EDGE('',*,*,#17392,.T.);
#22926=ORIENTED_EDGE('',*,*,#17405,.T.);
#22927=ORIENTED_EDGE('',*,*,#17367,.T.);
#22928=ORIENTED_EDGE('',*,*,#17405,.F.);
#22929=ORIENTED_EDGE('',*,*,#17406,.F.);
#22930=ORIENTED_EDGE('',*,*,#17407,.T.);
#22931=ORIENTED_EDGE('',*,*,#17408,.T.);
#22932=ORIENTED_EDGE('',*,*,#17409,.T.);
#22933=ORIENTED_EDGE('',*,*,#17410,.T.);
#22934=ORIENTED_EDGE('',*,*,#17411,.T.);
#22935=ORIENTED_EDGE('',*,*,#17412,.T.);
#22936=ORIENTED_EDGE('',*,*,#17413,.T.);
#22937=ORIENTED_EDGE('',*,*,#17414,.T.);
#22938=ORIENTED_EDGE('',*,*,#17415,.T.);
#22939=ORIENTED_EDGE('',*,*,#17416,.T.);
#22940=ORIENTED_EDGE('',*,*,#17417,.T.);
#22941=ORIENTED_EDGE('',*,*,#17418,.T.);
#22942=ORIENTED_EDGE('',*,*,#17406,.T.);
#22943=ORIENTED_EDGE('',*,*,#17419,.T.);
#22944=ORIENTED_EDGE('',*,*,#17366,.T.);
#22945=ORIENTED_EDGE('',*,*,#17419,.F.);
#22946=ORIENTED_EDGE('',*,*,#17420,.F.);
#22947=ORIENTED_EDGE('',*,*,#17421,.T.);
#22948=ORIENTED_EDGE('',*,*,#17422,.T.);
#22949=ORIENTED_EDGE('',*,*,#17417,.F.);
#22950=ORIENTED_EDGE('',*,*,#17422,.F.);
#22951=ORIENTED_EDGE('',*,*,#17423,.T.);
#22952=ORIENTED_EDGE('',*,*,#17424,.T.);
#22953=ORIENTED_EDGE('',*,*,#17418,.F.);
#22954=ORIENTED_EDGE('',*,*,#17424,.F.);
#22955=ORIENTED_EDGE('',*,*,#17425,.T.);
#22956=ORIENTED_EDGE('',*,*,#17426,.T.);
#22957=ORIENTED_EDGE('',*,*,#17407,.F.);
#22958=ORIENTED_EDGE('',*,*,#17426,.F.);
#22959=ORIENTED_EDGE('',*,*,#17427,.T.);
#22960=ORIENTED_EDGE('',*,*,#17428,.T.);
#22961=ORIENTED_EDGE('',*,*,#17408,.F.);
#22962=ORIENTED_EDGE('',*,*,#17428,.F.);
#22963=ORIENTED_EDGE('',*,*,#17429,.T.);
#22964=ORIENTED_EDGE('',*,*,#17430,.T.);
#22965=ORIENTED_EDGE('',*,*,#17409,.F.);
#22966=ORIENTED_EDGE('',*,*,#17430,.F.);
#22967=ORIENTED_EDGE('',*,*,#17431,.T.);
#22968=ORIENTED_EDGE('',*,*,#17432,.T.);
#22969=ORIENTED_EDGE('',*,*,#17410,.F.);
#22970=ORIENTED_EDGE('',*,*,#17432,.F.);
#22971=ORIENTED_EDGE('',*,*,#17433,.T.);
#22972=ORIENTED_EDGE('',*,*,#17434,.T.);
#22973=ORIENTED_EDGE('',*,*,#17411,.F.);
#22974=ORIENTED_EDGE('',*,*,#17434,.F.);
#22975=ORIENTED_EDGE('',*,*,#17435,.T.);
#22976=ORIENTED_EDGE('',*,*,#17436,.T.);
#22977=ORIENTED_EDGE('',*,*,#17412,.F.);
#22978=ORIENTED_EDGE('',*,*,#17436,.F.);
#22979=ORIENTED_EDGE('',*,*,#17437,.T.);
#22980=ORIENTED_EDGE('',*,*,#17438,.T.);
#22981=ORIENTED_EDGE('',*,*,#17413,.F.);
#22982=ORIENTED_EDGE('',*,*,#17438,.F.);
#22983=ORIENTED_EDGE('',*,*,#17439,.T.);
#22984=ORIENTED_EDGE('',*,*,#17440,.T.);
#22985=ORIENTED_EDGE('',*,*,#17414,.F.);
#22986=ORIENTED_EDGE('',*,*,#17440,.F.);
#22987=ORIENTED_EDGE('',*,*,#17441,.T.);
#22988=ORIENTED_EDGE('',*,*,#17442,.T.);
#22989=ORIENTED_EDGE('',*,*,#17415,.F.);
#22990=ORIENTED_EDGE('',*,*,#17442,.F.);
#22991=ORIENTED_EDGE('',*,*,#17443,.T.);
#22992=ORIENTED_EDGE('',*,*,#17420,.T.);
#22993=ORIENTED_EDGE('',*,*,#17416,.F.);
#22994=ORIENTED_EDGE('',*,*,#17421,.F.);
#22995=ORIENTED_EDGE('',*,*,#17443,.F.);
#22996=ORIENTED_EDGE('',*,*,#17441,.F.);
#22997=ORIENTED_EDGE('',*,*,#17439,.F.);
#22998=ORIENTED_EDGE('',*,*,#17437,.F.);
#22999=ORIENTED_EDGE('',*,*,#17435,.F.);
#23000=ORIENTED_EDGE('',*,*,#17433,.F.);
#23001=ORIENTED_EDGE('',*,*,#17431,.F.);
#23002=ORIENTED_EDGE('',*,*,#17429,.F.);
#23003=ORIENTED_EDGE('',*,*,#17427,.F.);
#23004=ORIENTED_EDGE('',*,*,#17425,.F.);
#23005=ORIENTED_EDGE('',*,*,#17423,.F.);
#23006=ORIENTED_EDGE('',*,*,#17444,.F.);
#23007=ORIENTED_EDGE('',*,*,#17445,.T.);
#23008=ORIENTED_EDGE('',*,*,#17446,.T.);
#23009=ORIENTED_EDGE('',*,*,#17403,.F.);
#23010=ORIENTED_EDGE('',*,*,#17446,.F.);
#23011=ORIENTED_EDGE('',*,*,#17447,.T.);
#23012=ORIENTED_EDGE('',*,*,#17448,.T.);
#23013=ORIENTED_EDGE('',*,*,#17404,.F.);
#23014=ORIENTED_EDGE('',*,*,#17448,.F.);
#23015=ORIENTED_EDGE('',*,*,#17449,.T.);
#23016=ORIENTED_EDGE('',*,*,#17450,.T.);
#23017=ORIENTED_EDGE('',*,*,#17393,.F.);
#23018=ORIENTED_EDGE('',*,*,#17450,.F.);
#23019=ORIENTED_EDGE('',*,*,#17451,.T.);
#23020=ORIENTED_EDGE('',*,*,#17452,.T.);
#23021=ORIENTED_EDGE('',*,*,#17394,.F.);
#23022=ORIENTED_EDGE('',*,*,#17452,.F.);
#23023=ORIENTED_EDGE('',*,*,#17453,.T.);
#23024=ORIENTED_EDGE('',*,*,#17454,.T.);
#23025=ORIENTED_EDGE('',*,*,#17395,.F.);
#23026=ORIENTED_EDGE('',*,*,#17454,.F.);
#23027=ORIENTED_EDGE('',*,*,#17455,.T.);
#23028=ORIENTED_EDGE('',*,*,#17456,.T.);
#23029=ORIENTED_EDGE('',*,*,#17396,.F.);
#23030=ORIENTED_EDGE('',*,*,#17456,.F.);
#23031=ORIENTED_EDGE('',*,*,#17457,.T.);
#23032=ORIENTED_EDGE('',*,*,#17458,.T.);
#23033=ORIENTED_EDGE('',*,*,#17397,.F.);
#23034=ORIENTED_EDGE('',*,*,#17458,.F.);
#23035=ORIENTED_EDGE('',*,*,#17459,.T.);
#23036=ORIENTED_EDGE('',*,*,#17460,.T.);
#23037=ORIENTED_EDGE('',*,*,#17398,.F.);
#23038=ORIENTED_EDGE('',*,*,#17460,.F.);
#23039=ORIENTED_EDGE('',*,*,#17461,.T.);
#23040=ORIENTED_EDGE('',*,*,#17462,.T.);
#23041=ORIENTED_EDGE('',*,*,#17399,.F.);
#23042=ORIENTED_EDGE('',*,*,#17462,.F.);
#23043=ORIENTED_EDGE('',*,*,#17463,.T.);
#23044=ORIENTED_EDGE('',*,*,#17464,.T.);
#23045=ORIENTED_EDGE('',*,*,#17400,.F.);
#23046=ORIENTED_EDGE('',*,*,#17464,.F.);
#23047=ORIENTED_EDGE('',*,*,#17465,.T.);
#23048=ORIENTED_EDGE('',*,*,#17466,.T.);
#23049=ORIENTED_EDGE('',*,*,#17401,.F.);
#23050=ORIENTED_EDGE('',*,*,#17466,.F.);
#23051=ORIENTED_EDGE('',*,*,#17467,.T.);
#23052=ORIENTED_EDGE('',*,*,#17444,.T.);
#23053=ORIENTED_EDGE('',*,*,#17402,.F.);
#23054=ORIENTED_EDGE('',*,*,#17445,.F.);
#23055=ORIENTED_EDGE('',*,*,#17467,.F.);
#23056=ORIENTED_EDGE('',*,*,#17465,.F.);
#23057=ORIENTED_EDGE('',*,*,#17463,.F.);
#23058=ORIENTED_EDGE('',*,*,#17461,.F.);
#23059=ORIENTED_EDGE('',*,*,#17459,.F.);
#23060=ORIENTED_EDGE('',*,*,#17457,.F.);
#23061=ORIENTED_EDGE('',*,*,#17455,.F.);
#23062=ORIENTED_EDGE('',*,*,#17453,.F.);
#23063=ORIENTED_EDGE('',*,*,#17451,.F.);
#23064=ORIENTED_EDGE('',*,*,#17449,.F.);
#23065=ORIENTED_EDGE('',*,*,#17447,.F.);
#23066=ORIENTED_EDGE('',*,*,#17222,.T.);
#23067=ORIENTED_EDGE('',*,*,#17220,.T.);
#23068=ORIENTED_EDGE('',*,*,#17218,.T.);
#23069=ORIENTED_EDGE('',*,*,#17468,.T.);
#23070=ORIENTED_EDGE('',*,*,#17469,.T.);
#23071=ORIENTED_EDGE('',*,*,#17470,.T.);
#23072=ORIENTED_EDGE('',*,*,#17471,.T.);
#23073=ORIENTED_EDGE('',*,*,#17472,.T.);
#23074=ORIENTED_EDGE('',*,*,#17473,.T.);
#23075=ORIENTED_EDGE('',*,*,#17474,.T.);
#23076=ORIENTED_EDGE('',*,*,#17475,.T.);
#23077=ORIENTED_EDGE('',*,*,#17476,.T.);
#23078=ORIENTED_EDGE('',*,*,#17210,.F.);
#23079=ORIENTED_EDGE('',*,*,#17223,.F.);
#23080=ORIENTED_EDGE('',*,*,#17476,.F.);
#23081=ORIENTED_EDGE('',*,*,#17477,.T.);
#23082=ORIENTED_EDGE('',*,*,#17211,.F.);
#23083=ORIENTED_EDGE('',*,*,#17477,.F.);
#23084=ORIENTED_EDGE('',*,*,#17475,.F.);
#23085=ORIENTED_EDGE('',*,*,#17478,.T.);
#23086=ORIENTED_EDGE('',*,*,#17212,.F.);
#23087=ORIENTED_EDGE('',*,*,#17478,.F.);
#23088=ORIENTED_EDGE('',*,*,#17474,.F.);
#23089=ORIENTED_EDGE('',*,*,#17479,.T.);
#23090=ORIENTED_EDGE('',*,*,#17213,.F.);
#23091=ORIENTED_EDGE('',*,*,#17479,.F.);
#23092=ORIENTED_EDGE('',*,*,#17473,.F.);
#23093=ORIENTED_EDGE('',*,*,#17480,.T.);
#23094=ORIENTED_EDGE('',*,*,#17214,.F.);
#23095=ORIENTED_EDGE('',*,*,#17480,.F.);
#23096=ORIENTED_EDGE('',*,*,#17472,.F.);
#23097=ORIENTED_EDGE('',*,*,#17481,.T.);
#23098=ORIENTED_EDGE('',*,*,#17215,.F.);
#23099=ORIENTED_EDGE('',*,*,#17481,.F.);
#23100=ORIENTED_EDGE('',*,*,#17471,.F.);
#23101=ORIENTED_EDGE('',*,*,#17482,.T.);
#23102=ORIENTED_EDGE('',*,*,#17216,.F.);
#23103=ORIENTED_EDGE('',*,*,#17482,.F.);
#23104=ORIENTED_EDGE('',*,*,#17470,.F.);
#23105=ORIENTED_EDGE('',*,*,#17483,.T.);
#23106=ORIENTED_EDGE('',*,*,#17201,.F.);
#23107=ORIENTED_EDGE('',*,*,#17483,.F.);
#23108=ORIENTED_EDGE('',*,*,#17469,.F.);
#23109=ORIENTED_EDGE('',*,*,#17484,.T.);
#23110=ORIENTED_EDGE('',*,*,#17205,.F.);
#23111=ORIENTED_EDGE('',*,*,#17206,.F.);
#23112=ORIENTED_EDGE('',*,*,#17484,.F.);
#23113=ORIENTED_EDGE('',*,*,#17468,.F.);
#23114=ORIENTED_EDGE('',*,*,#17217,.T.);
#23115=ORIENTED_EDGE('',*,*,#17485,.F.);
#23116=ORIENTED_EDGE('',*,*,#17486,.F.);
#23117=ORIENTED_EDGE('',*,*,#17236,.F.);
#23118=ORIENTED_EDGE('',*,*,#17487,.F.);
#23119=ORIENTED_EDGE('',*,*,#17487,.T.);
#23120=ORIENTED_EDGE('',*,*,#17235,.F.);
#23121=ORIENTED_EDGE('',*,*,#17488,.F.);
#23122=ORIENTED_EDGE('',*,*,#17489,.F.);
#23123=ORIENTED_EDGE('',*,*,#17490,.F.);
#23124=ORIENTED_EDGE('',*,*,#17488,.T.);
#23125=ORIENTED_EDGE('',*,*,#17234,.F.);
#23126=ORIENTED_EDGE('',*,*,#17242,.F.);
#23127=ORIENTED_EDGE('',*,*,#17491,.F.);
#23128=ORIENTED_EDGE('',*,*,#17243,.T.);
#23129=ORIENTED_EDGE('',*,*,#17232,.F.);
#23130=ORIENTED_EDGE('',*,*,#17256,.F.);
#23131=ORIENTED_EDGE('',*,*,#17492,.F.);
#23132=ORIENTED_EDGE('',*,*,#17493,.F.);
#23133=ORIENTED_EDGE('',*,*,#17494,.F.);
#23134=ORIENTED_EDGE('',*,*,#17268,.F.);
#23135=ORIENTED_EDGE('',*,*,#17337,.F.);
#23136=ORIENTED_EDGE('',*,*,#17229,.T.);
#23137=ORIENTED_EDGE('',*,*,#17495,.T.);
#23138=ORIENTED_EDGE('',*,*,#17365,.T.);
#23139=ORIENTED_EDGE('',*,*,#17496,.T.);
#23140=ORIENTED_EDGE('',*,*,#17269,.T.);
#23141=ORIENTED_EDGE('',*,*,#17494,.T.);
#23142=ORIENTED_EDGE('',*,*,#17497,.F.);
#23143=ORIENTED_EDGE('',*,*,#17237,.F.);
#23144=ORIENTED_EDGE('',*,*,#17486,.T.);
#23145=ORIENTED_EDGE('',*,*,#17498,.F.);
#23146=ORIENTED_EDGE('',*,*,#17249,.F.);
#23147=ORIENTED_EDGE('',*,*,#17264,.F.);
#23148=ORIENTED_EDGE('',*,*,#17499,.F.);
#23149=ORIENTED_EDGE('',*,*,#17363,.F.);
#23150=ORIENTED_EDGE('',*,*,#17500,.F.);
#23151=ORIENTED_EDGE('',*,*,#17254,.F.);
#23152=ORIENTED_EDGE('',*,*,#17501,.F.);
#23153=ORIENTED_EDGE('',*,*,#17246,.T.);
#23154=ORIENTED_EDGE('',*,*,#17265,.F.);
#23155=ORIENTED_EDGE('',*,*,#17248,.F.);
#23156=ORIENTED_EDGE('',*,*,#17502,.F.);
#23157=ORIENTED_EDGE('',*,*,#17503,.T.);
#23158=ORIENTED_EDGE('',*,*,#17266,.F.);
#23159=ORIENTED_EDGE('',*,*,#17503,.F.);
#23160=ORIENTED_EDGE('',*,*,#17504,.F.);
#23161=ORIENTED_EDGE('',*,*,#17492,.T.);
#23162=ORIENTED_EDGE('',*,*,#17267,.F.);
#23163=ORIENTED_EDGE('',*,*,#17499,.T.);
#23164=ORIENTED_EDGE('',*,*,#17270,.F.);
#23165=ORIENTED_EDGE('',*,*,#17496,.F.);
#23166=ORIENTED_EDGE('',*,*,#17364,.T.);
#23167=ORIENTED_EDGE('',*,*,#17505,.T.);
#23168=ORIENTED_EDGE('',*,*,#17500,.T.);
#23169=ORIENTED_EDGE('',*,*,#17362,.F.);
#23170=ORIENTED_EDGE('',*,*,#17495,.F.);
#23171=ORIENTED_EDGE('',*,*,#17238,.T.);
#23172=ORIENTED_EDGE('',*,*,#17285,.F.);
#23173=ORIENTED_EDGE('',*,*,#17506,.F.);
#23174=ORIENTED_EDGE('',*,*,#17507,.F.);
#23175=ORIENTED_EDGE('',*,*,#17508,.T.);
#23176=ORIENTED_EDGE('',*,*,#17286,.F.);
#23177=ORIENTED_EDGE('',*,*,#17508,.F.);
#23178=ORIENTED_EDGE('',*,*,#17509,.F.);
#23179=ORIENTED_EDGE('',*,*,#17510,.T.);
#23180=ORIENTED_EDGE('',*,*,#17284,.F.);
#23181=ORIENTED_EDGE('',*,*,#17511,.F.);
#23182=ORIENTED_EDGE('',*,*,#17512,.F.);
#23183=ORIENTED_EDGE('',*,*,#17506,.T.);
#23184=ORIENTED_EDGE('',*,*,#17275,.F.);
#23185=ORIENTED_EDGE('',*,*,#17510,.F.);
#23186=ORIENTED_EDGE('',*,*,#17513,.F.);
#23187=ORIENTED_EDGE('',*,*,#17514,.T.);
#23188=ORIENTED_EDGE('',*,*,#17276,.F.);
#23189=ORIENTED_EDGE('',*,*,#17514,.F.);
#23190=ORIENTED_EDGE('',*,*,#17515,.F.);
#23191=ORIENTED_EDGE('',*,*,#17516,.T.);
#23192=ORIENTED_EDGE('',*,*,#17277,.F.);
#23193=ORIENTED_EDGE('',*,*,#17516,.F.);
#23194=ORIENTED_EDGE('',*,*,#17517,.F.);
#23195=ORIENTED_EDGE('',*,*,#17518,.T.);
#23196=ORIENTED_EDGE('',*,*,#17278,.F.);
#23197=ORIENTED_EDGE('',*,*,#17518,.F.);
#23198=ORIENTED_EDGE('',*,*,#17519,.F.);
#23199=ORIENTED_EDGE('',*,*,#17520,.T.);
#23200=ORIENTED_EDGE('',*,*,#17279,.F.);
#23201=ORIENTED_EDGE('',*,*,#17520,.F.);
#23202=ORIENTED_EDGE('',*,*,#17521,.F.);
#23203=ORIENTED_EDGE('',*,*,#17522,.T.);
#23204=ORIENTED_EDGE('',*,*,#17280,.F.);
#23205=ORIENTED_EDGE('',*,*,#17522,.F.);
#23206=ORIENTED_EDGE('',*,*,#17523,.F.);
#23207=ORIENTED_EDGE('',*,*,#17524,.T.);
#23208=ORIENTED_EDGE('',*,*,#17281,.F.);
#23209=ORIENTED_EDGE('',*,*,#17524,.F.);
#23210=ORIENTED_EDGE('',*,*,#17525,.F.);
#23211=ORIENTED_EDGE('',*,*,#17526,.T.);
#23212=ORIENTED_EDGE('',*,*,#17282,.F.);
#23213=ORIENTED_EDGE('',*,*,#17526,.F.);
#23214=ORIENTED_EDGE('',*,*,#17527,.F.);
#23215=ORIENTED_EDGE('',*,*,#17528,.T.);
#23216=ORIENTED_EDGE('',*,*,#17505,.F.);
#23217=ORIENTED_EDGE('',*,*,#17529,.T.);
#23218=ORIENTED_EDGE('',*,*,#17530,.T.);
#23219=ORIENTED_EDGE('',*,*,#17529,.F.);
#23220=ORIENTED_EDGE('',*,*,#17530,.F.);
#23221=ORIENTED_EDGE('',*,*,#17527,.T.);
#23222=ORIENTED_EDGE('',*,*,#17525,.T.);
#23223=ORIENTED_EDGE('',*,*,#17523,.T.);
#23224=ORIENTED_EDGE('',*,*,#17521,.T.);
#23225=ORIENTED_EDGE('',*,*,#17519,.T.);
#23226=ORIENTED_EDGE('',*,*,#17517,.T.);
#23227=ORIENTED_EDGE('',*,*,#17515,.T.);
#23228=ORIENTED_EDGE('',*,*,#17513,.T.);
#23229=ORIENTED_EDGE('',*,*,#17509,.T.);
#23230=ORIENTED_EDGE('',*,*,#17507,.T.);
#23231=ORIENTED_EDGE('',*,*,#17512,.T.);
#23232=ORIENTED_EDGE('',*,*,#17531,.T.);
#23233=ORIENTED_EDGE('',*,*,#17283,.F.);
#23234=ORIENTED_EDGE('',*,*,#17528,.F.);
#23235=ORIENTED_EDGE('',*,*,#17531,.F.);
#23236=ORIENTED_EDGE('',*,*,#17511,.T.);
#23237=ORIENTED_EDGE('',*,*,#17295,.F.);
#23238=ORIENTED_EDGE('',*,*,#17291,.T.);
#23239=ORIENTED_EDGE('',*,*,#17287,.T.);
#23240=ORIENTED_EDGE('',*,*,#17532,.T.);
#23241=ORIENTED_EDGE('',*,*,#17533,.T.);
#23242=ORIENTED_EDGE('',*,*,#17534,.T.);
#23243=ORIENTED_EDGE('',*,*,#17535,.T.);
#23244=ORIENTED_EDGE('',*,*,#17536,.T.);
#23245=ORIENTED_EDGE('',*,*,#17537,.T.);
#23246=ORIENTED_EDGE('',*,*,#17538,.T.);
#23247=ORIENTED_EDGE('',*,*,#17539,.T.);
#23248=ORIENTED_EDGE('',*,*,#17540,.T.);
#23249=ORIENTED_EDGE('',*,*,#17541,.T.);
#23250=ORIENTED_EDGE('',*,*,#17289,.T.);
#23251=ORIENTED_EDGE('',*,*,#17293,.T.);
#23252=ORIENTED_EDGE('',*,*,#17542,.T.);
#23253=ORIENTED_EDGE('',*,*,#17543,.T.);
#23254=ORIENTED_EDGE('',*,*,#17544,.T.);
#23255=ORIENTED_EDGE('',*,*,#17545,.T.);
#23256=ORIENTED_EDGE('',*,*,#17546,.T.);
#23257=ORIENTED_EDGE('',*,*,#17547,.T.);
#23258=ORIENTED_EDGE('',*,*,#17548,.T.);
#23259=ORIENTED_EDGE('',*,*,#17549,.T.);
#23260=ORIENTED_EDGE('',*,*,#17550,.T.);
#23261=ORIENTED_EDGE('',*,*,#17551,.T.);
#23262=ORIENTED_EDGE('',*,*,#17532,.F.);
#23263=ORIENTED_EDGE('',*,*,#17290,.F.);
#23264=ORIENTED_EDGE('',*,*,#17551,.F.);
#23265=ORIENTED_EDGE('',*,*,#17552,.T.);
#23266=ORIENTED_EDGE('',*,*,#17533,.F.);
#23267=ORIENTED_EDGE('',*,*,#17552,.F.);
#23268=ORIENTED_EDGE('',*,*,#17550,.F.);
#23269=ORIENTED_EDGE('',*,*,#17553,.T.);
#23270=ORIENTED_EDGE('',*,*,#17534,.F.);
#23271=ORIENTED_EDGE('',*,*,#17553,.F.);
#23272=ORIENTED_EDGE('',*,*,#17549,.F.);
#23273=ORIENTED_EDGE('',*,*,#17554,.T.);
#23274=ORIENTED_EDGE('',*,*,#17535,.F.);
#23275=ORIENTED_EDGE('',*,*,#17554,.F.);
#23276=ORIENTED_EDGE('',*,*,#17548,.F.);
#23277=ORIENTED_EDGE('',*,*,#17555,.T.);
#23278=ORIENTED_EDGE('',*,*,#17556,.T.);
#23279=ORIENTED_EDGE('',*,*,#17536,.F.);
#23280=ORIENTED_EDGE('',*,*,#17555,.F.);
#23281=ORIENTED_EDGE('',*,*,#17547,.F.);
#23282=ORIENTED_EDGE('',*,*,#17537,.F.);
#23283=ORIENTED_EDGE('',*,*,#17556,.F.);
#23284=ORIENTED_EDGE('',*,*,#17546,.F.);
#23285=ORIENTED_EDGE('',*,*,#17557,.T.);
#23286=ORIENTED_EDGE('',*,*,#17538,.F.);
#23287=ORIENTED_EDGE('',*,*,#17557,.F.);
#23288=ORIENTED_EDGE('',*,*,#17545,.F.);
#23289=ORIENTED_EDGE('',*,*,#17558,.T.);
#23290=ORIENTED_EDGE('',*,*,#17539,.F.);
#23291=ORIENTED_EDGE('',*,*,#17558,.F.);
#23292=ORIENTED_EDGE('',*,*,#17544,.F.);
#23293=ORIENTED_EDGE('',*,*,#17559,.T.);
#23294=ORIENTED_EDGE('',*,*,#17540,.F.);
#23295=ORIENTED_EDGE('',*,*,#17559,.F.);
#23296=ORIENTED_EDGE('',*,*,#17543,.F.);
#23297=ORIENTED_EDGE('',*,*,#17560,.T.);
#23298=ORIENTED_EDGE('',*,*,#17541,.F.);
#23299=ORIENTED_EDGE('',*,*,#17560,.F.);
#23300=ORIENTED_EDGE('',*,*,#17542,.F.);
#23301=ORIENTED_EDGE('',*,*,#17292,.T.);
#23302=ORIENTED_EDGE('',*,*,#17561,.T.);
#23303=ORIENTED_EDGE('',*,*,#17562,.F.);
#23304=ORIENTED_EDGE('',*,*,#17563,.T.);
#23305=ORIENTED_EDGE('',*,*,#17564,.T.);
#23306=ORIENTED_EDGE('',*,*,#17565,.F.);
#23307=ORIENTED_EDGE('',*,*,#17566,.F.);
#23308=ORIENTED_EDGE('',*,*,#17564,.F.);
#23309=ORIENTED_EDGE('',*,*,#17567,.T.);
#23310=ORIENTED_EDGE('',*,*,#17568,.F.);
#23311=ORIENTED_EDGE('',*,*,#17569,.F.);
#23312=ORIENTED_EDGE('',*,*,#17570,.T.);
#23313=ORIENTED_EDGE('',*,*,#17571,.T.);
#23314=ORIENTED_EDGE('',*,*,#17572,.F.);
#23315=ORIENTED_EDGE('',*,*,#17573,.F.);
#23316=ORIENTED_EDGE('',*,*,#17571,.F.);
#23317=ORIENTED_EDGE('',*,*,#17574,.T.);
#23318=ORIENTED_EDGE('',*,*,#17575,.F.);
#23319=ORIENTED_EDGE('',*,*,#17576,.F.);
#23320=ORIENTED_EDGE('',*,*,#17577,.F.);
#23321=ORIENTED_EDGE('',*,*,#17578,.T.);
#23322=ORIENTED_EDGE('',*,*,#17579,.T.);
#23323=ORIENTED_EDGE('',*,*,#17580,.F.);
#23324=ORIENTED_EDGE('',*,*,#17579,.F.);
#23325=ORIENTED_EDGE('',*,*,#17581,.T.);
#23326=ORIENTED_EDGE('',*,*,#17575,.T.);
#23327=ORIENTED_EDGE('',*,*,#17582,.T.);
#23328=ORIENTED_EDGE('',*,*,#17580,.T.);
#23329=ORIENTED_EDGE('',*,*,#17582,.F.);
#23330=ORIENTED_EDGE('',*,*,#17577,.T.);
#23331=ORIENTED_EDGE('',*,*,#17576,.T.);
#23332=ORIENTED_EDGE('',*,*,#17583,.F.);
#23333=ORIENTED_EDGE('',*,*,#17584,.F.);
#23334=ORIENTED_EDGE('',*,*,#17583,.T.);
#23335=ORIENTED_EDGE('',*,*,#17585,.T.);
#23336=ORIENTED_EDGE('',*,*,#17565,.T.);
#23337=ORIENTED_EDGE('',*,*,#17566,.T.);
#23338=ORIENTED_EDGE('',*,*,#17585,.F.);
#23339=ORIENTED_EDGE('',*,*,#17584,.T.);
#23340=ORIENTED_EDGE('',*,*,#17568,.T.);
#23341=ORIENTED_EDGE('',*,*,#17586,.T.);
#23342=ORIENTED_EDGE('',*,*,#17572,.T.);
#23343=ORIENTED_EDGE('',*,*,#17573,.T.);
#23344=ORIENTED_EDGE('',*,*,#17586,.F.);
#23345=ORIENTED_EDGE('',*,*,#17569,.T.);
#23346=ORIENTED_EDGE('',*,*,#17587,.F.);
#23347=ORIENTED_EDGE('',*,*,#17588,.F.);
#23348=ORIENTED_EDGE('',*,*,#17589,.T.);
#23349=ORIENTED_EDGE('',*,*,#17590,.T.);
#23350=ORIENTED_EDGE('',*,*,#17589,.F.);
#23351=ORIENTED_EDGE('',*,*,#17587,.T.);
#23352=ORIENTED_EDGE('',*,*,#17588,.T.);
#23353=ORIENTED_EDGE('',*,*,#17591,.T.);
#23354=ORIENTED_EDGE('',*,*,#17561,.F.);
#23355=ORIENTED_EDGE('',*,*,#17591,.F.);
#23356=ORIENTED_EDGE('',*,*,#17570,.F.);
#23357=ORIENTED_EDGE('',*,*,#17574,.F.);
#23358=ORIENTED_EDGE('',*,*,#17578,.F.);
#23359=ORIENTED_EDGE('',*,*,#17581,.F.);
#23360=ORIENTED_EDGE('',*,*,#17563,.F.);
#23361=ORIENTED_EDGE('',*,*,#17567,.F.);
#23362=ORIENTED_EDGE('',*,*,#17590,.F.);
#23363=ORIENTED_EDGE('',*,*,#17592,.T.);
#23364=ORIENTED_EDGE('',*,*,#17562,.T.);
#23365=ORIENTED_EDGE('',*,*,#17593,.T.);
#23366=ORIENTED_EDGE('',*,*,#17594,.F.);
#23367=ORIENTED_EDGE('',*,*,#17595,.F.);
#23368=ORIENTED_EDGE('',*,*,#17593,.F.);
#23369=ORIENTED_EDGE('',*,*,#17497,.T.);
#23370=ORIENTED_EDGE('',*,*,#17493,.T.);
#23371=ORIENTED_EDGE('',*,*,#17504,.T.);
#23372=ORIENTED_EDGE('',*,*,#17502,.T.);
#23373=ORIENTED_EDGE('',*,*,#17247,.T.);
#23374=ORIENTED_EDGE('',*,*,#17501,.T.);
#23375=ORIENTED_EDGE('',*,*,#17253,.T.);
#23376=ORIENTED_EDGE('',*,*,#17250,.T.);
#23377=ORIENTED_EDGE('',*,*,#17498,.T.);
#23378=ORIENTED_EDGE('',*,*,#17485,.T.);
#23379=ORIENTED_EDGE('',*,*,#17489,.T.);
#23380=ORIENTED_EDGE('',*,*,#17490,.T.);
#23381=ORIENTED_EDGE('',*,*,#17244,.T.);
#23382=ORIENTED_EDGE('',*,*,#17491,.T.);
#23383=ORIENTED_EDGE('',*,*,#17258,.T.);
#23384=ORIENTED_EDGE('',*,*,#17336,.T.);
#23385=ORIENTED_EDGE('',*,*,#17596,.T.);
#23386=ORIENTED_EDGE('',*,*,#17597,.F.);
#23387=ORIENTED_EDGE('',*,*,#17598,.F.);
#23388=ORIENTED_EDGE('',*,*,#17599,.T.);
#23389=ORIENTED_EDGE('',*,*,#17600,.T.);
#23390=ORIENTED_EDGE('',*,*,#17601,.T.);
#23391=ORIENTED_EDGE('',*,*,#17602,.T.);
#23392=ORIENTED_EDGE('',*,*,#17603,.T.);
#23393=ORIENTED_EDGE('',*,*,#17604,.T.);
#23394=ORIENTED_EDGE('',*,*,#17605,.T.);
#23395=ORIENTED_EDGE('',*,*,#17606,.T.);
#23396=ORIENTED_EDGE('',*,*,#17607,.T.);
#23397=ORIENTED_EDGE('',*,*,#17608,.T.);
#23398=ORIENTED_EDGE('',*,*,#17609,.T.);
#23399=ORIENTED_EDGE('',*,*,#17610,.T.);
#23400=ORIENTED_EDGE('',*,*,#17611,.T.);
#23401=ORIENTED_EDGE('',*,*,#17612,.T.);
#23402=ORIENTED_EDGE('',*,*,#17613,.T.);
#23403=ORIENTED_EDGE('',*,*,#17614,.T.);
#23404=ORIENTED_EDGE('',*,*,#17598,.T.);
#23405=ORIENTED_EDGE('',*,*,#17615,.T.);
#23406=ORIENTED_EDGE('',*,*,#17599,.F.);
#23407=ORIENTED_EDGE('',*,*,#17614,.F.);
#23408=ORIENTED_EDGE('',*,*,#17616,.T.);
#23409=ORIENTED_EDGE('',*,*,#17617,.F.);
#23410=ORIENTED_EDGE('',*,*,#17618,.T.);
#23411=ORIENTED_EDGE('',*,*,#17619,.T.);
#23412=ORIENTED_EDGE('',*,*,#17620,.F.);
#23413=ORIENTED_EDGE('',*,*,#17621,.T.);
#23414=ORIENTED_EDGE('',*,*,#17622,.F.);
#23415=ORIENTED_EDGE('',*,*,#17623,.T.);
#23416=ORIENTED_EDGE('',*,*,#17624,.T.);
#23417=ORIENTED_EDGE('',*,*,#17625,.T.);
#23418=ORIENTED_EDGE('',*,*,#17626,.F.);
#23419=ORIENTED_EDGE('',*,*,#17627,.F.);
#23420=ORIENTED_EDGE('',*,*,#17628,.F.);
#23421=ORIENTED_EDGE('',*,*,#17629,.T.);
#23422=ORIENTED_EDGE('',*,*,#17630,.T.);
#23423=ORIENTED_EDGE('',*,*,#17631,.T.);
#23424=ORIENTED_EDGE('',*,*,#17632,.T.);
#23425=ORIENTED_EDGE('',*,*,#17633,.F.);
#23426=ORIENTED_EDGE('',*,*,#17634,.T.);
#23427=ORIENTED_EDGE('',*,*,#17635,.T.);
#23428=ORIENTED_EDGE('',*,*,#17636,.T.);
#23429=ORIENTED_EDGE('',*,*,#17637,.F.);
#23430=ORIENTED_EDGE('',*,*,#17638,.F.);
#23431=ORIENTED_EDGE('',*,*,#17632,.F.);
#23432=ORIENTED_EDGE('',*,*,#17639,.T.);
#23433=ORIENTED_EDGE('',*,*,#17640,.F.);
#23434=ORIENTED_EDGE('',*,*,#17639,.F.);
#23435=ORIENTED_EDGE('',*,*,#17631,.F.);
#23436=ORIENTED_EDGE('',*,*,#17641,.T.);
#23437=ORIENTED_EDGE('',*,*,#17642,.F.);
#23438=ORIENTED_EDGE('',*,*,#17641,.F.);
#23439=ORIENTED_EDGE('',*,*,#17630,.F.);
#23440=ORIENTED_EDGE('',*,*,#17643,.T.);
#23441=ORIENTED_EDGE('',*,*,#17644,.F.);
#23442=ORIENTED_EDGE('',*,*,#17643,.F.);
#23443=ORIENTED_EDGE('',*,*,#17629,.F.);
#23444=ORIENTED_EDGE('',*,*,#17638,.T.);
#23445=ORIENTED_EDGE('',*,*,#17645,.T.);
#23446=ORIENTED_EDGE('',*,*,#17646,.T.);
#23447=ORIENTED_EDGE('',*,*,#17647,.T.);
#23448=ORIENTED_EDGE('',*,*,#17648,.T.);
#23449=ORIENTED_EDGE('',*,*,#17649,.F.);
#23450=ORIENTED_EDGE('',*,*,#17628,.T.);
#23451=ORIENTED_EDGE('',*,*,#17650,.T.);
#23452=ORIENTED_EDGE('',*,*,#17620,.T.);
#23453=ORIENTED_EDGE('',*,*,#17651,.F.);
#23454=ORIENTED_EDGE('',*,*,#17652,.F.);
#23455=ORIENTED_EDGE('',*,*,#17648,.F.);
#23456=ORIENTED_EDGE('',*,*,#17653,.T.);
#23457=ORIENTED_EDGE('',*,*,#17654,.F.);
#23458=ORIENTED_EDGE('',*,*,#17653,.F.);
#23459=ORIENTED_EDGE('',*,*,#17647,.F.);
#23460=ORIENTED_EDGE('',*,*,#17655,.T.);
#23461=ORIENTED_EDGE('',*,*,#17656,.F.);
#23462=ORIENTED_EDGE('',*,*,#17655,.F.);
#23463=ORIENTED_EDGE('',*,*,#17646,.F.);
#23464=ORIENTED_EDGE('',*,*,#17657,.T.);
#23465=ORIENTED_EDGE('',*,*,#17658,.F.);
#23466=ORIENTED_EDGE('',*,*,#17657,.F.);
#23467=ORIENTED_EDGE('',*,*,#17645,.F.);
#23468=ORIENTED_EDGE('',*,*,#17652,.T.);
#23469=ORIENTED_EDGE('',*,*,#17659,.F.);
#23470=ORIENTED_EDGE('',*,*,#17659,.T.);
#23471=ORIENTED_EDGE('',*,*,#17660,.T.);
#23472=ORIENTED_EDGE('',*,*,#17661,.F.);
#23473=ORIENTED_EDGE('',*,*,#17662,.F.);
#23474=ORIENTED_EDGE('',*,*,#17660,.F.);
#23475=ORIENTED_EDGE('',*,*,#17662,.T.);
#23476=ORIENTED_EDGE('',*,*,#17663,.T.);
#23477=ORIENTED_EDGE('',*,*,#17664,.F.);
#23478=ORIENTED_EDGE('',*,*,#17663,.F.);
#23479=ORIENTED_EDGE('',*,*,#17661,.T.);
#23480=ORIENTED_EDGE('',*,*,#17665,.F.);
#23481=ORIENTED_EDGE('',*,*,#17665,.T.);
#23482=ORIENTED_EDGE('',*,*,#17666,.T.);
#23483=ORIENTED_EDGE('',*,*,#17667,.F.);
#23484=ORIENTED_EDGE('',*,*,#17668,.F.);
#23485=ORIENTED_EDGE('',*,*,#17666,.F.);
#23486=ORIENTED_EDGE('',*,*,#17668,.T.);
#23487=ORIENTED_EDGE('',*,*,#17669,.T.);
#23488=ORIENTED_EDGE('',*,*,#17670,.F.);
#23489=ORIENTED_EDGE('',*,*,#17669,.F.);
#23490=ORIENTED_EDGE('',*,*,#17667,.T.);
#23491=ORIENTED_EDGE('',*,*,#17671,.F.);
#23492=ORIENTED_EDGE('',*,*,#17671,.T.);
#23493=ORIENTED_EDGE('',*,*,#17672,.T.);
#23494=ORIENTED_EDGE('',*,*,#17673,.F.);
#23495=ORIENTED_EDGE('',*,*,#17674,.F.);
#23496=ORIENTED_EDGE('',*,*,#17672,.F.);
#23497=ORIENTED_EDGE('',*,*,#17674,.T.);
#23498=ORIENTED_EDGE('',*,*,#17675,.T.);
#23499=ORIENTED_EDGE('',*,*,#17676,.F.);
#23500=ORIENTED_EDGE('',*,*,#17675,.F.);
#23501=ORIENTED_EDGE('',*,*,#17673,.T.);
#23502=ORIENTED_EDGE('',*,*,#17677,.F.);
#23503=ORIENTED_EDGE('',*,*,#17677,.T.);
#23504=ORIENTED_EDGE('',*,*,#17678,.T.);
#23505=ORIENTED_EDGE('',*,*,#17679,.F.);
#23506=ORIENTED_EDGE('',*,*,#17680,.F.);
#23507=ORIENTED_EDGE('',*,*,#17678,.F.);
#23508=ORIENTED_EDGE('',*,*,#17680,.T.);
#23509=ORIENTED_EDGE('',*,*,#17681,.T.);
#23510=ORIENTED_EDGE('',*,*,#17682,.F.);
#23511=ORIENTED_EDGE('',*,*,#17681,.F.);
#23512=ORIENTED_EDGE('',*,*,#17679,.T.);
#23513=ORIENTED_EDGE('',*,*,#17595,.T.);
#23514=ORIENTED_EDGE('',*,*,#17683,.T.);
#23515=ORIENTED_EDGE('',*,*,#17684,.F.);
#23516=ORIENTED_EDGE('',*,*,#17683,.F.);
#23517=ORIENTED_EDGE('',*,*,#17594,.T.);
#23518=ORIENTED_EDGE('',*,*,#17684,.T.);
#23519=ORIENTED_EDGE('',*,*,#17685,.T.);
#23520=ORIENTED_EDGE('',*,*,#17686,.T.);
#23521=ORIENTED_EDGE('',*,*,#17687,.F.);
#23522=ORIENTED_EDGE('',*,*,#17688,.T.);
#23523=ORIENTED_EDGE('',*,*,#17664,.T.);
#23524=ORIENTED_EDGE('',*,*,#17670,.T.);
#23525=ORIENTED_EDGE('',*,*,#17676,.T.);
#23526=ORIENTED_EDGE('',*,*,#17682,.T.);
#23527=ORIENTED_EDGE('',*,*,#17689,.F.);
#23528=ORIENTED_EDGE('',*,*,#17689,.T.);
#23529=ORIENTED_EDGE('',*,*,#17690,.T.);
#23530=ORIENTED_EDGE('',*,*,#17691,.F.);
#23531=ORIENTED_EDGE('',*,*,#17690,.F.);
#23532=ORIENTED_EDGE('',*,*,#17691,.T.);
#23533=ORIENTED_EDGE('',*,*,#17692,.F.);
#23534=ORIENTED_EDGE('',*,*,#17692,.T.);
#23535=ORIENTED_EDGE('',*,*,#17693,.T.);
#23536=ORIENTED_EDGE('',*,*,#17694,.F.);
#23537=ORIENTED_EDGE('',*,*,#17693,.F.);
#23538=ORIENTED_EDGE('',*,*,#17694,.T.);
#23539=ORIENTED_EDGE('',*,*,#17642,.T.);
#23540=ORIENTED_EDGE('',*,*,#17644,.T.);
#23541=ORIENTED_EDGE('',*,*,#17637,.T.);
#23542=ORIENTED_EDGE('',*,*,#17640,.T.);
#23543=ORIENTED_EDGE('',*,*,#17656,.T.);
#23544=ORIENTED_EDGE('',*,*,#17658,.T.);
#23545=ORIENTED_EDGE('',*,*,#17651,.T.);
#23546=ORIENTED_EDGE('',*,*,#17654,.T.);
#23547=ORIENTED_EDGE('',*,*,#17695,.F.);
#23548=ORIENTED_EDGE('',*,*,#17695,.T.);
#23549=ORIENTED_EDGE('',*,*,#17696,.T.);
#23550=ORIENTED_EDGE('',*,*,#17697,.F.);
#23551=ORIENTED_EDGE('',*,*,#17696,.F.);
#23552=ORIENTED_EDGE('',*,*,#17697,.T.);
#23553=ORIENTED_EDGE('',*,*,#17698,.F.);
#23554=ORIENTED_EDGE('',*,*,#17698,.T.);
#23555=ORIENTED_EDGE('',*,*,#17699,.T.);
#23556=ORIENTED_EDGE('',*,*,#17592,.F.);
#23557=ORIENTED_EDGE('',*,*,#17699,.F.);
#23558=ORIENTED_EDGE('',*,*,#17700,.T.);
#23559=ORIENTED_EDGE('',*,*,#17701,.F.);
#23560=ORIENTED_EDGE('',*,*,#17685,.F.);
#23561=ORIENTED_EDGE('',*,*,#17702,.T.);
#23562=ORIENTED_EDGE('',*,*,#17700,.F.);
#23563=ORIENTED_EDGE('',*,*,#17702,.F.);
#23564=ORIENTED_EDGE('',*,*,#17701,.T.);
#23565=ORIENTED_EDGE('',*,*,#17703,.T.);
#23566=ORIENTED_EDGE('',*,*,#17704,.F.);
#23567=ORIENTED_EDGE('',*,*,#17703,.F.);
#23568=ORIENTED_EDGE('',*,*,#17704,.T.);
#23569=ORIENTED_EDGE('',*,*,#17705,.T.);
#23570=ORIENTED_EDGE('',*,*,#17706,.T.);
#23571=ORIENTED_EDGE('',*,*,#17688,.F.);
#23572=ORIENTED_EDGE('',*,*,#17706,.F.);
#23573=ORIENTED_EDGE('',*,*,#17705,.F.);
#23574=ORIENTED_EDGE('',*,*,#17707,.T.);
#23575=ORIENTED_EDGE('',*,*,#17708,.T.);
#23576=ORIENTED_EDGE('',*,*,#17709,.T.);
#23577=ORIENTED_EDGE('',*,*,#17707,.F.);
#23578=ORIENTED_EDGE('',*,*,#17709,.F.);
#23579=ORIENTED_EDGE('',*,*,#17708,.F.);
#23580=ORIENTED_EDGE('',*,*,#17710,.T.);
#23581=ORIENTED_EDGE('',*,*,#17711,.T.);
#23582=ORIENTED_EDGE('',*,*,#17712,.T.);
#23583=ORIENTED_EDGE('',*,*,#17710,.F.);
#23584=ORIENTED_EDGE('',*,*,#17712,.F.);
#23585=ORIENTED_EDGE('',*,*,#17713,.T.);
#23586=ORIENTED_EDGE('',*,*,#17711,.F.);
#23587=ORIENTED_EDGE('',*,*,#17687,.T.);
#23588=ORIENTED_EDGE('',*,*,#17714,.T.);
#23589=ORIENTED_EDGE('',*,*,#17713,.F.);
#23590=ORIENTED_EDGE('',*,*,#17714,.F.);
#23591=ORIENTED_EDGE('',*,*,#17715,.T.);
#23592=ORIENTED_EDGE('',*,*,#17716,.T.);
#23593=ORIENTED_EDGE('',*,*,#17686,.F.);
#23594=ORIENTED_EDGE('',*,*,#17716,.F.);
#23595=ORIENTED_EDGE('',*,*,#17715,.F.);
#23596=ORIENTED_EDGE('',*,*,#17717,.T.);
#23597=ORIENTED_EDGE('',*,*,#17718,.T.);
#23598=ORIENTED_EDGE('',*,*,#17719,.T.);
#23599=ORIENTED_EDGE('',*,*,#17717,.F.);
#23600=ORIENTED_EDGE('',*,*,#17719,.F.);
#23601=ORIENTED_EDGE('',*,*,#17718,.F.);
#23602=ORIENTED_EDGE('',*,*,#17720,.F.);
#23603=ORIENTED_EDGE('',*,*,#17721,.T.);
#23604=ORIENTED_EDGE('',*,*,#17722,.T.);
#23605=ORIENTED_EDGE('',*,*,#17636,.F.);
#23606=ORIENTED_EDGE('',*,*,#17723,.T.);
#23607=ORIENTED_EDGE('',*,*,#17724,.F.);
#23608=ORIENTED_EDGE('',*,*,#17725,.F.);
#23609=ORIENTED_EDGE('',*,*,#17726,.T.);
#23610=ORIENTED_EDGE('',*,*,#17720,.T.);
#23611=ORIENTED_EDGE('',*,*,#17727,.F.);
#23612=ORIENTED_EDGE('',*,*,#17728,.T.);
#23613=ORIENTED_EDGE('',*,*,#17729,.T.);
#23614=ORIENTED_EDGE('',*,*,#17725,.T.);
#23615=ORIENTED_EDGE('',*,*,#17730,.F.);
#23616=ORIENTED_EDGE('',*,*,#17731,.F.);
#23617=ORIENTED_EDGE('',*,*,#17634,.F.);
#23618=ORIENTED_EDGE('',*,*,#17622,.T.);
#23619=ORIENTED_EDGE('',*,*,#17732,.T.);
#23620=ORIENTED_EDGE('',*,*,#17626,.T.);
#23621=ORIENTED_EDGE('',*,*,#17733,.T.);
#23622=ORIENTED_EDGE('',*,*,#17734,.T.);
#23623=ORIENTED_EDGE('',*,*,#17735,.T.);
#23624=ORIENTED_EDGE('',*,*,#17617,.T.);
#23625=ORIENTED_EDGE('',*,*,#17733,.F.);
#23626=ORIENTED_EDGE('',*,*,#17625,.F.);
#23627=ORIENTED_EDGE('',*,*,#17627,.T.);
#23628=ORIENTED_EDGE('',*,*,#17732,.F.);
#23629=ORIENTED_EDGE('',*,*,#17621,.F.);
#23630=ORIENTED_EDGE('',*,*,#17650,.F.);
#23631=ORIENTED_EDGE('',*,*,#17731,.T.);
#23632=ORIENTED_EDGE('',*,*,#17736,.F.);
#23633=ORIENTED_EDGE('',*,*,#17723,.F.);
#23634=ORIENTED_EDGE('',*,*,#17635,.F.);
#23635=ORIENTED_EDGE('',*,*,#17730,.T.);
#23636=ORIENTED_EDGE('',*,*,#17727,.T.);
#23637=ORIENTED_EDGE('',*,*,#17724,.T.);
#23638=ORIENTED_EDGE('',*,*,#17736,.T.);
#23639=ORIENTED_EDGE('',*,*,#17737,.T.);
#23640=ORIENTED_EDGE('',*,*,#17728,.F.);
#23641=ORIENTED_EDGE('',*,*,#17738,.F.);
#23642=ORIENTED_EDGE('',*,*,#17722,.F.);
#23643=ORIENTED_EDGE('',*,*,#17739,.T.);
#23644=ORIENTED_EDGE('',*,*,#17737,.F.);
#23645=ORIENTED_EDGE('',*,*,#17740,.T.);
#23646=ORIENTED_EDGE('',*,*,#17741,.F.);
#23647=ORIENTED_EDGE('',*,*,#17740,.F.);
#23648=ORIENTED_EDGE('',*,*,#17739,.F.);
#23649=ORIENTED_EDGE('',*,*,#17721,.F.);
#23650=ORIENTED_EDGE('',*,*,#17726,.F.);
#23651=ORIENTED_EDGE('',*,*,#17729,.F.);
#23652=ORIENTED_EDGE('',*,*,#17741,.T.);
#23653=ORIENTED_EDGE('',*,*,#17738,.T.);
#23654=ORIENTED_EDGE('',*,*,#17633,.T.);
#23655=ORIENTED_EDGE('',*,*,#17742,.F.);
#23656=ORIENTED_EDGE('',*,*,#17743,.F.);
#23657=ORIENTED_EDGE('',*,*,#17744,.F.);
#23658=ORIENTED_EDGE('',*,*,#17745,.F.);
#23659=ORIENTED_EDGE('',*,*,#17746,.F.);
#23660=ORIENTED_EDGE('',*,*,#17747,.F.);
#23661=ORIENTED_EDGE('',*,*,#17748,.F.);
#23662=ORIENTED_EDGE('',*,*,#17749,.F.);
#23663=ORIENTED_EDGE('',*,*,#17750,.F.);
#23664=ORIENTED_EDGE('',*,*,#17596,.F.);
#23665=ORIENTED_EDGE('',*,*,#17615,.F.);
#23666=ORIENTED_EDGE('',*,*,#17751,.F.);
#23667=ORIENTED_EDGE('',*,*,#17752,.F.);
#23668=ORIENTED_EDGE('',*,*,#17753,.F.);
#23669=ORIENTED_EDGE('',*,*,#17754,.F.);
#23670=ORIENTED_EDGE('',*,*,#17755,.F.);
#23671=ORIENTED_EDGE('',*,*,#17618,.F.);
#23672=ORIENTED_EDGE('',*,*,#17735,.F.);
#23673=ORIENTED_EDGE('',*,*,#17624,.F.);
#23674=ORIENTED_EDGE('',*,*,#17756,.F.);
#23675=ORIENTED_EDGE('',*,*,#17757,.T.);
#23676=ORIENTED_EDGE('',*,*,#17734,.F.);
#23677=ORIENTED_EDGE('',*,*,#17758,.T.);
#23678=ORIENTED_EDGE('',*,*,#17757,.F.);
#23679=ORIENTED_EDGE('',*,*,#17758,.F.);
#23680=ORIENTED_EDGE('',*,*,#17619,.F.);
#23681=ORIENTED_EDGE('',*,*,#17756,.T.);
#23682=ORIENTED_EDGE('',*,*,#17623,.F.);
#23683=ORIENTED_EDGE('',*,*,#17759,.F.);
#23684=ORIENTED_EDGE('',*,*,#17649,.T.);
#23685=ORIENTED_EDGE('',*,*,#17759,.T.);
#23686=ORIENTED_EDGE('',*,*,#17760,.F.);
#23687=ORIENTED_EDGE('',*,*,#17761,.F.);
#23688=ORIENTED_EDGE('',*,*,#17762,.F.);
#23689=ORIENTED_EDGE('',*,*,#17763,.F.);
#23690=ORIENTED_EDGE('',*,*,#17764,.F.);
#23691=ORIENTED_EDGE('',*,*,#17765,.F.);
#23692=ORIENTED_EDGE('',*,*,#17766,.F.);
#23693=ORIENTED_EDGE('',*,*,#17767,.F.);
#23694=ORIENTED_EDGE('',*,*,#17768,.F.);
#23695=ORIENTED_EDGE('',*,*,#17769,.F.);
#23696=ORIENTED_EDGE('',*,*,#17770,.F.);
#23697=ORIENTED_EDGE('',*,*,#17771,.F.);
#23698=ORIENTED_EDGE('',*,*,#17772,.F.);
#23699=ORIENTED_EDGE('',*,*,#17773,.F.);
#23700=ORIENTED_EDGE('',*,*,#17774,.F.);
#23701=ORIENTED_EDGE('',*,*,#17775,.F.);
#23702=ORIENTED_EDGE('',*,*,#17769,.T.);
#23703=ORIENTED_EDGE('',*,*,#17776,.F.);
#23704=ORIENTED_EDGE('',*,*,#17777,.F.);
#23705=ORIENTED_EDGE('',*,*,#17778,.T.);
#23706=ORIENTED_EDGE('',*,*,#17768,.T.);
#23707=ORIENTED_EDGE('',*,*,#17779,.F.);
#23708=ORIENTED_EDGE('',*,*,#17780,.F.);
#23709=ORIENTED_EDGE('',*,*,#17776,.T.);
#23710=ORIENTED_EDGE('',*,*,#17767,.T.);
#23711=ORIENTED_EDGE('',*,*,#17781,.F.);
#23712=ORIENTED_EDGE('',*,*,#17782,.F.);
#23713=ORIENTED_EDGE('',*,*,#17779,.T.);
#23714=ORIENTED_EDGE('',*,*,#17766,.T.);
#23715=ORIENTED_EDGE('',*,*,#17783,.F.);
#23716=ORIENTED_EDGE('',*,*,#17784,.F.);
#23717=ORIENTED_EDGE('',*,*,#17781,.T.);
#23718=ORIENTED_EDGE('',*,*,#17765,.T.);
#23719=ORIENTED_EDGE('',*,*,#17785,.F.);
#23720=ORIENTED_EDGE('',*,*,#17786,.F.);
#23721=ORIENTED_EDGE('',*,*,#17783,.T.);
#23722=ORIENTED_EDGE('',*,*,#17764,.T.);
#23723=ORIENTED_EDGE('',*,*,#17787,.F.);
#23724=ORIENTED_EDGE('',*,*,#17788,.F.);
#23725=ORIENTED_EDGE('',*,*,#17785,.T.);
#23726=ORIENTED_EDGE('',*,*,#17763,.T.);
#23727=ORIENTED_EDGE('',*,*,#17789,.F.);
#23728=ORIENTED_EDGE('',*,*,#17790,.F.);
#23729=ORIENTED_EDGE('',*,*,#17787,.T.);
#23730=ORIENTED_EDGE('',*,*,#17762,.T.);
#23731=ORIENTED_EDGE('',*,*,#17791,.F.);
#23732=ORIENTED_EDGE('',*,*,#17792,.F.);
#23733=ORIENTED_EDGE('',*,*,#17789,.T.);
#23734=ORIENTED_EDGE('',*,*,#17761,.T.);
#23735=ORIENTED_EDGE('',*,*,#17793,.F.);
#23736=ORIENTED_EDGE('',*,*,#17794,.F.);
#23737=ORIENTED_EDGE('',*,*,#17791,.T.);
#23738=ORIENTED_EDGE('',*,*,#17793,.T.);
#23739=ORIENTED_EDGE('',*,*,#17760,.T.);
#23740=ORIENTED_EDGE('',*,*,#17795,.F.);
#23741=ORIENTED_EDGE('',*,*,#17796,.F.);
#23742=ORIENTED_EDGE('',*,*,#17775,.T.);
#23743=ORIENTED_EDGE('',*,*,#17797,.F.);
#23744=ORIENTED_EDGE('',*,*,#17798,.F.);
#23745=ORIENTED_EDGE('',*,*,#17795,.T.);
#23746=ORIENTED_EDGE('',*,*,#17774,.T.);
#23747=ORIENTED_EDGE('',*,*,#17799,.F.);
#23748=ORIENTED_EDGE('',*,*,#17800,.F.);
#23749=ORIENTED_EDGE('',*,*,#17797,.T.);
#23750=ORIENTED_EDGE('',*,*,#17773,.T.);
#23751=ORIENTED_EDGE('',*,*,#17801,.F.);
#23752=ORIENTED_EDGE('',*,*,#17802,.F.);
#23753=ORIENTED_EDGE('',*,*,#17799,.T.);
#23754=ORIENTED_EDGE('',*,*,#17772,.T.);
#23755=ORIENTED_EDGE('',*,*,#17803,.F.);
#23756=ORIENTED_EDGE('',*,*,#17804,.F.);
#23757=ORIENTED_EDGE('',*,*,#17801,.T.);
#23758=ORIENTED_EDGE('',*,*,#17771,.T.);
#23759=ORIENTED_EDGE('',*,*,#17805,.F.);
#23760=ORIENTED_EDGE('',*,*,#17806,.F.);
#23761=ORIENTED_EDGE('',*,*,#17803,.T.);
#23762=ORIENTED_EDGE('',*,*,#17770,.T.);
#23763=ORIENTED_EDGE('',*,*,#17778,.F.);
#23764=ORIENTED_EDGE('',*,*,#17807,.F.);
#23765=ORIENTED_EDGE('',*,*,#17805,.T.);
#23766=ORIENTED_EDGE('',*,*,#17777,.T.);
#23767=ORIENTED_EDGE('',*,*,#17780,.T.);
#23768=ORIENTED_EDGE('',*,*,#17782,.T.);
#23769=ORIENTED_EDGE('',*,*,#17784,.T.);
#23770=ORIENTED_EDGE('',*,*,#17786,.T.);
#23771=ORIENTED_EDGE('',*,*,#17788,.T.);
#23772=ORIENTED_EDGE('',*,*,#17790,.T.);
#23773=ORIENTED_EDGE('',*,*,#17792,.T.);
#23774=ORIENTED_EDGE('',*,*,#17794,.T.);
#23775=ORIENTED_EDGE('',*,*,#17796,.T.);
#23776=ORIENTED_EDGE('',*,*,#17798,.T.);
#23777=ORIENTED_EDGE('',*,*,#17800,.T.);
#23778=ORIENTED_EDGE('',*,*,#17802,.T.);
#23779=ORIENTED_EDGE('',*,*,#17804,.T.);
#23780=ORIENTED_EDGE('',*,*,#17806,.T.);
#23781=ORIENTED_EDGE('',*,*,#17807,.T.);
#23782=ORIENTED_EDGE('',*,*,#17750,.T.);
#23783=ORIENTED_EDGE('',*,*,#17808,.F.);
#23784=ORIENTED_EDGE('',*,*,#17600,.F.);
#23785=ORIENTED_EDGE('',*,*,#17597,.T.);
#23786=ORIENTED_EDGE('',*,*,#17749,.T.);
#23787=ORIENTED_EDGE('',*,*,#17809,.F.);
#23788=ORIENTED_EDGE('',*,*,#17601,.F.);
#23789=ORIENTED_EDGE('',*,*,#17808,.T.);
#23790=ORIENTED_EDGE('',*,*,#17748,.T.);
#23791=ORIENTED_EDGE('',*,*,#17810,.F.);
#23792=ORIENTED_EDGE('',*,*,#17602,.F.);
#23793=ORIENTED_EDGE('',*,*,#17809,.T.);
#23794=ORIENTED_EDGE('',*,*,#17747,.T.);
#23795=ORIENTED_EDGE('',*,*,#17811,.F.);
#23796=ORIENTED_EDGE('',*,*,#17603,.F.);
#23797=ORIENTED_EDGE('',*,*,#17810,.T.);
#23798=ORIENTED_EDGE('',*,*,#17746,.T.);
#23799=ORIENTED_EDGE('',*,*,#17812,.F.);
#23800=ORIENTED_EDGE('',*,*,#17604,.F.);
#23801=ORIENTED_EDGE('',*,*,#17811,.T.);
#23802=ORIENTED_EDGE('',*,*,#17745,.T.);
#23803=ORIENTED_EDGE('',*,*,#17813,.F.);
#23804=ORIENTED_EDGE('',*,*,#17605,.F.);
#23805=ORIENTED_EDGE('',*,*,#17812,.T.);
#23806=ORIENTED_EDGE('',*,*,#17744,.T.);
#23807=ORIENTED_EDGE('',*,*,#17814,.F.);
#23808=ORIENTED_EDGE('',*,*,#17606,.F.);
#23809=ORIENTED_EDGE('',*,*,#17813,.T.);
#23810=ORIENTED_EDGE('',*,*,#17743,.T.);
#23811=ORIENTED_EDGE('',*,*,#17815,.F.);
#23812=ORIENTED_EDGE('',*,*,#17607,.F.);
#23813=ORIENTED_EDGE('',*,*,#17814,.T.);
#23814=ORIENTED_EDGE('',*,*,#17815,.T.);
#23815=ORIENTED_EDGE('',*,*,#17742,.T.);
#23816=ORIENTED_EDGE('',*,*,#17816,.F.);
#23817=ORIENTED_EDGE('',*,*,#17608,.F.);
#23818=ORIENTED_EDGE('',*,*,#17755,.T.);
#23819=ORIENTED_EDGE('',*,*,#17817,.F.);
#23820=ORIENTED_EDGE('',*,*,#17609,.F.);
#23821=ORIENTED_EDGE('',*,*,#17816,.T.);
#23822=ORIENTED_EDGE('',*,*,#17754,.T.);
#23823=ORIENTED_EDGE('',*,*,#17818,.F.);
#23824=ORIENTED_EDGE('',*,*,#17610,.F.);
#23825=ORIENTED_EDGE('',*,*,#17817,.T.);
#23826=ORIENTED_EDGE('',*,*,#17753,.T.);
#23827=ORIENTED_EDGE('',*,*,#17819,.F.);
#23828=ORIENTED_EDGE('',*,*,#17611,.F.);
#23829=ORIENTED_EDGE('',*,*,#17818,.T.);
#23830=ORIENTED_EDGE('',*,*,#17752,.T.);
#23831=ORIENTED_EDGE('',*,*,#17820,.F.);
#23832=ORIENTED_EDGE('',*,*,#17612,.F.);
#23833=ORIENTED_EDGE('',*,*,#17819,.T.);
#23834=ORIENTED_EDGE('',*,*,#17751,.T.);
#23835=ORIENTED_EDGE('',*,*,#17616,.F.);
#23836=ORIENTED_EDGE('',*,*,#17613,.F.);
#23837=ORIENTED_EDGE('',*,*,#17820,.T.);
#31224=PLANE('',#34571);
#31225=PLANE('',#34572);
#31226=PLANE('',#34573);
#31227=PLANE('',#34574);
#31228=PLANE('',#34585);
#31229=PLANE('',#34586);
#31230=PLANE('',#34595);
#31231=PLANE('',#34609);
#31232=PLANE('',#34611);
#31233=PLANE('',#34613);
#31234=PLANE('',#34620);
#31235=PLANE('',#34622);
#31236=PLANE('',#34624);
#31237=PLANE('',#34626);
#31238=PLANE('',#34628);
#31239=PLANE('',#34630);
#31240=PLANE('',#34632);
#31241=PLANE('',#34634);
#31242=PLANE('',#34636);
#31243=PLANE('',#34638);
#31244=PLANE('',#34640);
#31245=PLANE('',#34642);
#31246=PLANE('',#34644);
#31247=PLANE('',#34646);
#31248=PLANE('',#34651);
#31249=PLANE('',#34655);
#31250=PLANE('',#34659);
#31251=PLANE('',#34663);
#31252=PLANE('',#34664);
#31253=PLANE('',#34665);
#31254=PLANE('',#34674);
#31255=PLANE('',#34677);
#31256=PLANE('',#34680);
#31257=PLANE('',#34683);
#31258=PLANE('',#34684);
#31259=PLANE('',#34715);
#31260=PLANE('',#34716);
#31261=PLANE('',#34717);
#31262=PLANE('',#34718);
#31263=PLANE('',#34719);
#31264=PLANE('',#34720);
#31265=PLANE('',#34721);
#31266=PLANE('',#34722);
#31267=PLANE('',#34723);
#31268=PLANE('',#34724);
#31269=PLANE('',#34725);
#31270=PLANE('',#34726);
#31271=PLANE('',#34727);
#31272=PLANE('',#34728);
#31273=PLANE('',#34729);
#31274=PLANE('',#34730);
#31275=PLANE('',#34731);
#31276=PLANE('',#34732);
#31277=PLANE('',#34733);
#31278=PLANE('',#34734);
#31279=PLANE('',#34735);
#31280=PLANE('',#34736);
#31281=PLANE('',#34737);
#31282=PLANE('',#34738);
#31283=PLANE('',#34739);
#31284=PLANE('',#34740);
#31285=PLANE('',#34741);
#31286=PLANE('',#34742);
#31287=PLANE('',#34743);
#31288=PLANE('',#34744);
#31289=PLANE('',#34745);
#31290=PLANE('',#34746);
#31291=PLANE('',#34747);
#31292=PLANE('',#34748);
#31293=PLANE('',#34749);
#31294=PLANE('',#34750);
#31295=PLANE('',#34752);
#31296=PLANE('',#34753);
#31297=PLANE('',#34755);
#31298=PLANE('',#34758);
#31299=PLANE('',#34760);
#31300=PLANE('',#34762);
#31301=PLANE('',#34764);
#31302=PLANE('',#34766);
#31303=PLANE('',#34767);
#31304=PLANE('',#34769);
#31305=PLANE('',#34770);
#31306=PLANE('',#34771);
#31307=PLANE('',#34772);
#31308=PLANE('',#34773);
#31309=PLANE('',#34774);
#31310=PLANE('',#34775);
#31311=PLANE('',#34776);
#31312=PLANE('',#34777);
#31313=PLANE('',#34778);
#31314=PLANE('',#34779);
#31315=PLANE('',#34780);
#31316=PLANE('',#34783);
#31317=PLANE('',#34784);
#31318=PLANE('',#34785);
#31319=PLANE('',#34797);
#31320=PLANE('',#34798);
#31321=PLANE('',#34799);
#31322=PLANE('',#34800);
#31323=PLANE('',#34801);
#31324=PLANE('',#34802);
#31325=PLANE('',#34803);
#31326=PLANE('',#34804);
#31327=PLANE('',#34805);
#31328=PLANE('',#34806);
#31329=PLANE('',#34807);
#31330=PLANE('',#34808);
#31331=PLANE('',#34814);
#31332=PLANE('',#34820);
#31333=PLANE('',#34826);
#31334=PLANE('',#34837);
#31335=PLANE('',#34838);
#31336=PLANE('',#34843);
#31337=PLANE('',#34845);
#31338=PLANE('',#34846);
#31339=PLANE('',#34848);
#31340=PLANE('',#34849);
#31341=PLANE('',#34850);
#31342=PLANE('',#34857);
#31343=PLANE('',#34860);
#31344=PLANE('',#34861);
#31345=PLANE('',#34868);
#31346=PLANE('',#34871);
#31347=PLANE('',#34872);
#31348=PLANE('',#34879);
#31349=PLANE('',#34886);
#31350=PLANE('',#34893);
#31351=PLANE('',#34902);
#31352=PLANE('',#34910);
#31353=PLANE('',#34914);
#31354=PLANE('',#34918);
#31355=PLANE('',#34921);
#31356=PLANE('',#34927);
#31357=PLANE('',#34930);
#31358=PLANE('',#34934);
#31359=PLANE('',#34935);
#31360=PLANE('',#34939);
#31361=PLANE('',#34944);
#31362=PLANE('',#34948);
#31363=PLANE('',#34949);
#31364=PLANE('',#34953);
#31365=PLANE('',#34954);
#31366=PLANE('',#34963);
#31367=PLANE('',#34970);
#31368=PLANE('',#34986);
#31369=PLANE('',#35009);
#31370=PLANE('',#35010);
#31371=PLANE('',#35011);
#31372=PLANE('',#35012);
#31373=PLANE('',#35013);
#31374=PLANE('',#35014);
#31375=PLANE('',#35015);
#31376=PLANE('',#35016);
#31377=PLANE('',#35017);
#31378=PLANE('',#35018);
#31379=PLANE('',#35019);
#31380=PLANE('',#35020);
#31381=PLANE('',#35021);
#31382=PLANE('',#35022);
#31383=PLANE('',#35023);
#31384=PLANE('',#35024);
#31385=PLANE('',#35025);
#31386=PLANE('',#35026);
#31387=PLANE('',#35027);
#31388=PLANE('',#35028);
#31389=PLANE('',#35029);
#31390=PLANE('',#35030);
#31391=PLANE('',#35031);
#31392=PLANE('',#35032);
#31393=PLANE('',#35033);
#31394=PLANE('',#35034);
#31395=PLANE('',#35035);
#31396=PLANE('',#35036);
#31397=PLANE('',#35037);
#31398=PLANE('',#35038);
#31399=PLANE('',#35039);
#32160=ADVANCED_FACE('',(#4479),#870,.F.);
#32161=ADVANCED_FACE('',(#4480),#31224,.T.);
#32162=ADVANCED_FACE('',(#4481),#31225,.T.);
#32163=ADVANCED_FACE('',(#4482),#31226,.T.);
#32164=ADVANCED_FACE('',(#4483),#31227,.T.);
#32165=ADVANCED_FACE('',(#4484),#1107,.T.);
#32166=ADVANCED_FACE('',(#4485,#1923,#1924),#1108,.T.);
#32167=ADVANCED_FACE('',(#4486),#1109,.F.);
#32168=ADVANCED_FACE('',(#4487),#1110,.F.);
#32169=ADVANCED_FACE('',(#4488),#1111,.T.);
#32170=ADVANCED_FACE('',(#4489),#31228,.T.);
#32171=ADVANCED_FACE('',(#4490),#31229,.T.);
#32172=ADVANCED_FACE('',(#4491),#1112,.T.);
#32173=ADVANCED_FACE('',(#4492,#1925,#1926),#1113,.T.);
#32174=ADVANCED_FACE('',(#4493),#31230,.T.);
#32175=ADVANCED_FACE('',(#4494,#1927),#726,.T.);
#32176=ADVANCED_FACE('',(#4495),#31231,.T.);
#32177=ADVANCED_FACE('',(#4496),#31232,.T.);
#32178=ADVANCED_FACE('',(#4497),#31233,.T.);
#32179=ADVANCED_FACE('',(#4498),#1114,.T.);
#32180=ADVANCED_FACE('',(#4499),#1115,.T.);
#32181=ADVANCED_FACE('',(#4500),#31234,.T.);
#32182=ADVANCED_FACE('',(#4501),#31235,.T.);
#32183=ADVANCED_FACE('',(#4502),#31236,.T.);
#32184=ADVANCED_FACE('',(#4503),#31237,.T.);
#32185=ADVANCED_FACE('',(#4504),#31238,.T.);
#32186=ADVANCED_FACE('',(#4505),#31239,.T.);
#32187=ADVANCED_FACE('',(#4506),#31240,.T.);
#32188=ADVANCED_FACE('',(#4507),#31241,.T.);
#32189=ADVANCED_FACE('',(#4508),#31242,.T.);
#32190=ADVANCED_FACE('',(#4509),#31243,.T.);
#32191=ADVANCED_FACE('',(#4510),#31244,.T.);
#32192=ADVANCED_FACE('',(#4511),#31245,.T.);
#32193=ADVANCED_FACE('',(#4512),#31246,.T.);
#32194=ADVANCED_FACE('',(#4513,#1928),#727,.T.);
#32195=ADVANCED_FACE('',(#4514),#31247,.T.);
#32196=ADVANCED_FACE('',(#4515),#1116,.T.);
#32197=ADVANCED_FACE('',(#4516),#1117,.T.);
#32198=ADVANCED_FACE('',(#4517),#31248,.T.);
#32199=ADVANCED_FACE('',(#4518),#1118,.T.);
#32200=ADVANCED_FACE('',(#4519),#31249,.T.);
#32201=ADVANCED_FACE('',(#4520),#1119,.T.);
#32202=ADVANCED_FACE('',(#4521),#31250,.T.);
#32203=ADVANCED_FACE('',(#4522),#1120,.T.);
#32204=ADVANCED_FACE('',(#4523),#31251,.T.);
#32205=ADVANCED_FACE('',(#4524,#1929),#31252,.T.);
#32206=ADVANCED_FACE('',(#4525,#1930,#1931,#1932),#31253,.T.);
#32207=ADVANCED_FACE('',(#4526),#1121,.T.);
#32208=ADVANCED_FACE('',(#4527),#31254,.T.);
#32209=ADVANCED_FACE('',(#4528),#1122,.T.);
#32210=ADVANCED_FACE('',(#4529),#31255,.T.);
#32211=ADVANCED_FACE('',(#4530),#1123,.T.);
#32212=ADVANCED_FACE('',(#4531),#31256,.T.);
#32213=ADVANCED_FACE('',(#4532),#1124,.T.);
#32214=ADVANCED_FACE('',(#4533),#31257,.T.);
#32215=ADVANCED_FACE('',(#4534),#31258,.T.);
#32216=ADVANCED_FACE('',(#4535,#1933),#728,.T.);
#32217=ADVANCED_FACE('',(#4536),#1125,.T.);
#32218=ADVANCED_FACE('',(#4537,#1934),#729,.T.);
#32219=ADVANCED_FACE('',(#4538),#1126,.T.);
#32220=ADVANCED_FACE('',(#4539),#31259,.T.);
#32221=ADVANCED_FACE('',(#4540),#31260,.T.);
#32222=ADVANCED_FACE('',(#4541),#31261,.T.);
#32223=ADVANCED_FACE('',(#4542),#31262,.T.);
#32224=ADVANCED_FACE('',(#4543),#31263,.T.);
#32225=ADVANCED_FACE('',(#4544),#31264,.T.);
#32226=ADVANCED_FACE('',(#4545),#31265,.T.);
#32227=ADVANCED_FACE('',(#4546),#31266,.T.);
#32228=ADVANCED_FACE('',(#4547),#31267,.T.);
#32229=ADVANCED_FACE('',(#4548),#31268,.T.);
#32230=ADVANCED_FACE('',(#4549),#31269,.T.);
#32231=ADVANCED_FACE('',(#4550),#31270,.T.);
#32232=ADVANCED_FACE('',(#4551),#31271,.T.);
#32233=ADVANCED_FACE('',(#4552),#31272,.T.);
#32234=ADVANCED_FACE('',(#4553),#31273,.T.);
#32235=ADVANCED_FACE('',(#4554),#31274,.T.);
#32236=ADVANCED_FACE('',(#4555),#31275,.T.);
#32237=ADVANCED_FACE('',(#4556),#31276,.T.);
#32238=ADVANCED_FACE('',(#4557),#31277,.T.);
#32239=ADVANCED_FACE('',(#4558),#31278,.T.);
#32240=ADVANCED_FACE('',(#4559),#31279,.T.);
#32241=ADVANCED_FACE('',(#4560),#31280,.T.);
#32242=ADVANCED_FACE('',(#4561),#31281,.T.);
#32243=ADVANCED_FACE('',(#4562),#31282,.T.);
#32244=ADVANCED_FACE('',(#4563),#31283,.T.);
#32245=ADVANCED_FACE('',(#4564),#31284,.T.);
#32246=ADVANCED_FACE('',(#4565),#31285,.T.);
#32247=ADVANCED_FACE('',(#4566),#31286,.T.);
#32248=ADVANCED_FACE('',(#4567),#31287,.T.);
#32249=ADVANCED_FACE('',(#4568),#31288,.T.);
#32250=ADVANCED_FACE('',(#4569),#31289,.T.);
#32251=ADVANCED_FACE('',(#4570),#31290,.T.);
#32252=ADVANCED_FACE('',(#4571),#31291,.T.);
#32253=ADVANCED_FACE('',(#4572),#31292,.T.);
#32254=ADVANCED_FACE('',(#4573),#31293,.T.);
#32255=ADVANCED_FACE('',(#4574),#31294,.T.);
#32256=ADVANCED_FACE('',(#4575),#1127,.T.);
#32257=ADVANCED_FACE('',(#4576),#31295,.T.);
#32258=ADVANCED_FACE('',(#4577),#31296,.T.);
#32259=ADVANCED_FACE('',(#4578),#31297,.T.);
#32260=ADVANCED_FACE('',(#4579),#1128,.T.);
#32261=ADVANCED_FACE('',(#4580),#31298,.T.);
#32262=ADVANCED_FACE('',(#4581),#31299,.T.);
#32263=ADVANCED_FACE('',(#4582),#31300,.T.);
#32264=ADVANCED_FACE('',(#4583),#31301,.T.);
#32265=ADVANCED_FACE('',(#4584),#31302,.T.);
#32266=ADVANCED_FACE('',(#4585,#1935),#31303,.T.);
#32267=ADVANCED_FACE('',(#4586),#31304,.T.);
#32268=ADVANCED_FACE('',(#4587),#31305,.T.);
#32269=ADVANCED_FACE('',(#4588),#31306,.T.);
#32270=ADVANCED_FACE('',(#4589),#31307,.T.);
#32271=ADVANCED_FACE('',(#4590),#31308,.T.);
#32272=ADVANCED_FACE('',(#4591),#31309,.T.);
#32273=ADVANCED_FACE('',(#4592),#31310,.T.);
#32274=ADVANCED_FACE('',(#4593),#31311,.T.);
#32275=ADVANCED_FACE('',(#4594),#31312,.T.);
#32276=ADVANCED_FACE('',(#4595),#31313,.T.);
#32277=ADVANCED_FACE('',(#4596),#31314,.T.);
#32278=ADVANCED_FACE('',(#4597),#31315,.T.);
#32279=ADVANCED_FACE('',(#4598),#1129,.F.);
#32280=ADVANCED_FACE('',(#4599),#31316,.T.);
#32281=ADVANCED_FACE('',(#4600),#31317,.T.);
#32282=ADVANCED_FACE('',(#4601),#31318,.T.);
#32283=ADVANCED_FACE('',(#4602,#1936),#730,.T.);
#32284=ADVANCED_FACE('',(#4603),#31319,.T.);
#32285=ADVANCED_FACE('',(#4604),#31320,.T.);
#32286=ADVANCED_FACE('',(#4605),#31321,.T.);
#32287=ADVANCED_FACE('',(#4606),#31322,.T.);
#32288=ADVANCED_FACE('',(#4607),#31323,.T.);
#32289=ADVANCED_FACE('',(#4608),#31324,.T.);
#32290=ADVANCED_FACE('',(#4609),#31325,.T.);
#32291=ADVANCED_FACE('',(#4610),#31326,.T.);
#32292=ADVANCED_FACE('',(#4611),#31327,.T.);
#32293=ADVANCED_FACE('',(#4612),#31328,.T.);
#32294=ADVANCED_FACE('',(#4613),#31329,.T.);
#32295=ADVANCED_FACE('',(#4614,#1937),#31330,.T.);
#32296=ADVANCED_FACE('',(#4615),#1130,.T.);
#32297=ADVANCED_FACE('',(#4616),#31331,.T.);
#32298=ADVANCED_FACE('',(#4617),#1131,.T.);
#32299=ADVANCED_FACE('',(#4618),#31332,.T.);
#32300=ADVANCED_FACE('',(#4619),#1132,.T.);
#32301=ADVANCED_FACE('',(#4620),#871,.F.);
#32302=ADVANCED_FACE('',(#4621),#31333,.T.);
#32303=ADVANCED_FACE('',(#4622),#872,.F.);
#32304=ADVANCED_FACE('',(#4623),#873,.F.);
#32305=ADVANCED_FACE('',(#4624),#895,.T.);
#32306=ADVANCED_FACE('',(#4625,#1938,#1939,#1940),#1133,.T.);
#32307=ADVANCED_FACE('',(#4626),#31334,.T.);
#32308=ADVANCED_FACE('',(#4627),#31335,.T.);
#32309=ADVANCED_FACE('',(#4628,#1941),#1134,.T.);
#32310=ADVANCED_FACE('',(#4629),#31336,.T.);
#32311=ADVANCED_FACE('',(#4630),#31337,.T.);
#32312=ADVANCED_FACE('',(#4631),#31338,.T.);
#32313=ADVANCED_FACE('',(#4632),#31339,.T.);
#32314=ADVANCED_FACE('',(#4633),#31340,.T.);
#32315=ADVANCED_FACE('',(#4634,#1942),#31341,.T.);
#32316=ADVANCED_FACE('',(#4635),#1135,.T.);
#32317=ADVANCED_FACE('',(#4636),#31342,.T.);
#32318=ADVANCED_FACE('',(#4637),#1136,.T.);
#32319=ADVANCED_FACE('',(#4638),#31343,.T.);
#32320=ADVANCED_FACE('',(#4639,#1943),#31344,.T.);
#32321=ADVANCED_FACE('',(#4640),#1137,.T.);
#32322=ADVANCED_FACE('',(#4641),#31345,.T.);
#32323=ADVANCED_FACE('',(#4642),#1138,.T.);
#32324=ADVANCED_FACE('',(#4643),#31346,.T.);
#32325=ADVANCED_FACE('',(#4644),#31347,.T.);
#32326=ADVANCED_FACE('',(#4645),#1139,.F.);
#32327=ADVANCED_FACE('',(#4646),#578,.F.);
#32328=ADVANCED_FACE('',(#4647),#31348,.T.);
#32329=ADVANCED_FACE('',(#4648),#1140,.F.);
#32330=ADVANCED_FACE('',(#4649),#579,.F.);
#32331=ADVANCED_FACE('',(#4650),#31349,.T.);
#32332=ADVANCED_FACE('',(#4651),#1141,.F.);
#32333=ADVANCED_FACE('',(#4652),#580,.F.);
#32334=ADVANCED_FACE('',(#4653),#31350,.T.);
#32335=ADVANCED_FACE('',(#4654),#1142,.F.);
#32336=ADVANCED_FACE('',(#4655),#581,.F.);
#32337=ADVANCED_FACE('',(#4656),#582,.T.);
#32338=ADVANCED_FACE('',(#4657,#1944,#1945,#1946,#1947,#1948,#1949,#1950,
#1951,#1952),#31351,.T.);
#32339=ADVANCED_FACE('',(#4658),#1143,.T.);
#32340=ADVANCED_FACE('',(#4659,#1953),#31352,.T.);
#32341=ADVANCED_FACE('',(#4660),#1144,.F.);
#32342=ADVANCED_FACE('',(#4661,#1954,#1955,#1956),#31353,.T.);
#32343=ADVANCED_FACE('',(#4662),#1145,.T.);
#32344=ADVANCED_FACE('',(#4663,#1957),#31354,.T.);
#32345=ADVANCED_FACE('',(#4664),#1146,.F.);
#32346=ADVANCED_FACE('',(#4665,#1958),#31355,.T.);
#32347=ADVANCED_FACE('',(#4666),#1147,.F.);
#32348=ADVANCED_FACE('',(#4667),#1148,.F.);
#32349=ADVANCED_FACE('',(#4668),#31356,.T.);
#32350=ADVANCED_FACE('',(#4669),#1149,.F.);
#32351=ADVANCED_FACE('',(#4670,#1959),#31357,.T.);
#32352=ADVANCED_FACE('',(#4671),#1150,.F.);
#32353=ADVANCED_FACE('',(#4672),#31358,.T.);
#32354=ADVANCED_FACE('',(#4673),#31359,.T.);
#32355=ADVANCED_FACE('',(#4674),#1151,.F.);
#32356=ADVANCED_FACE('',(#4675,#1960),#31360,.T.);
#32357=ADVANCED_FACE('',(#4676),#1152,.F.);
#32358=ADVANCED_FACE('',(#4677),#1153,.F.);
#32359=ADVANCED_FACE('',(#4678,#1961),#31361,.T.);
#32360=ADVANCED_FACE('',(#4679),#1154,.F.);
#32361=ADVANCED_FACE('',(#4680),#31362,.T.);
#32362=ADVANCED_FACE('',(#4681),#31363,.T.);
#32363=ADVANCED_FACE('',(#4682),#1155,.F.);
#32364=ADVANCED_FACE('',(#4683),#31364,.T.);
#32365=ADVANCED_FACE('',(#4684,#1962),#31365,.T.);
#32366=ADVANCED_FACE('',(#4685),#1156,.F.);
#32367=ADVANCED_FACE('',(#4686),#1157,.F.);
#32368=ADVANCED_FACE('',(#4687),#1158,.F.);
#32369=ADVANCED_FACE('',(#4688,#1963),#31366,.T.);
#32370=ADVANCED_FACE('',(#4689),#1159,.T.);
#32371=ADVANCED_FACE('',(#4690),#1160,.T.);
#32372=ADVANCED_FACE('',(#4691,#1964),#31367,.T.);
#32373=ADVANCED_FACE('',(#4692,#1965),#731,.T.);
#32374=ADVANCED_FACE('',(#4693,#1966),#31368,.T.);
#32375=ADVANCED_FACE('',(#4694),#1161,.T.);
#32376=ADVANCED_FACE('',(#4695),#1162,.T.);
#32377=ADVANCED_FACE('',(#4696,#1967),#732,.T.);
#32378=ADVANCED_FACE('',(#4697),#31369,.T.);
#32379=ADVANCED_FACE('',(#4698),#31370,.T.);
#32380=ADVANCED_FACE('',(#4699),#31371,.T.);
#32381=ADVANCED_FACE('',(#4700),#31372,.T.);
#32382=ADVANCED_FACE('',(#4701),#31373,.T.);
#32383=ADVANCED_FACE('',(#4702),#31374,.T.);
#32384=ADVANCED_FACE('',(#4703),#31375,.T.);
#32385=ADVANCED_FACE('',(#4704),#31376,.T.);
#32386=ADVANCED_FACE('',(#4705),#31377,.T.);
#32387=ADVANCED_FACE('',(#4706),#31378,.T.);
#32388=ADVANCED_FACE('',(#4707),#31379,.T.);
#32389=ADVANCED_FACE('',(#4708),#31380,.T.);
#32390=ADVANCED_FACE('',(#4709),#31381,.T.);
#32391=ADVANCED_FACE('',(#4710),#31382,.T.);
#32392=ADVANCED_FACE('',(#4711),#31383,.T.);
#32393=ADVANCED_FACE('',(#4712),#31384,.T.);
#32394=ADVANCED_FACE('',(#4713),#31385,.T.);
#32395=ADVANCED_FACE('',(#4714),#31386,.T.);
#32396=ADVANCED_FACE('',(#4715),#31387,.T.);
#32397=ADVANCED_FACE('',(#4716),#31388,.T.);
#32398=ADVANCED_FACE('',(#4717),#31389,.T.);
#32399=ADVANCED_FACE('',(#4718),#31390,.T.);
#32400=ADVANCED_FACE('',(#4719),#31391,.T.);
#32401=ADVANCED_FACE('',(#4720),#31392,.T.);
#32402=ADVANCED_FACE('',(#4721),#31393,.T.);
#32403=ADVANCED_FACE('',(#4722),#31394,.T.);
#32404=ADVANCED_FACE('',(#4723),#31395,.T.);
#32405=ADVANCED_FACE('',(#4724),#31396,.T.);
#32406=ADVANCED_FACE('',(#4725),#31397,.T.);
#32407=ADVANCED_FACE('',(#4726),#31398,.T.);
#32408=ADVANCED_FACE('',(#4727),#31399,.T.);
#33799=CLOSED_SHELL('',(#32160,#32161,#32162,#32163,#32164,#32165,#32166,
#32167,#32168,#32169,#32170,#32171,#32172,#32173,#32174,#32175,#32176,#32177,
#32178,#32179,#32180,#32181,#32182,#32183,#32184,#32185,#32186,#32187,#32188,
#32189,#32190,#32191,#32192,#32193,#32194,#32195,#32196,#32197,#32198,#32199,
#32200,#32201,#32202,#32203,#32204,#32205,#32206,#32207,#32208,#32209,#32210,
#32211,#32212,#32213,#32214,#32215,#32216,#32217,#32218,#32219,#32220,#32221,
#32222,#32223,#32224,#32225,#32226,#32227,#32228,#32229,#32230,#32231,#32232,
#32233,#32234,#32235,#32236,#32237,#32238,#32239,#32240,#32241,#32242,#32243,
#32244,#32245,#32246,#32247,#32248,#32249,#32250,#32251,#32252,#32253,#32254,
#32255,#32256,#32257,#32258,#32259,#32260,#32261,#32262,#32263,#32264,#32265,
#32266,#32267,#32268,#32269,#32270,#32271,#32272,#32273,#32274,#32275,#32276,
#32277,#32278,#32279,#32280,#32281,#32282,#32283,#32284,#32285,#32286,#32287,
#32288,#32289,#32290,#32291,#32292,#32293,#32294,#32295,#32296,#32297,#32298,
#32299,#32300,#32301,#32302,#32303,#32304,#32305,#32306,#32307,#32308,#32309,
#32310,#32311,#32312,#32313,#32314,#32315,#32316,#32317,#32318,#32319,#32320,
#32321,#32322,#32323,#32324,#32325,#32326,#32327,#32328,#32329,#32330,#32331,
#32332,#32333,#32334,#32335,#32336,#32337,#32338,#32339,#32340,#32341,#32342,
#32343,#32344,#32345,#32346,#32347,#32348,#32349,#32350,#32351,#32352,#32353,
#32354,#32355,#32356,#32357,#32358,#32359,#32360,#32361,#32362,#32363,#32364,
#32365,#32366,#32367,#32368,#32369,#32370,#32371,#32372,#32373,#32374,#32375,
#32376,#32377,#32378,#32379,#32380,#32381,#32382,#32383,#32384,#32385,#32386,
#32387,#32388,#32389,#32390,#32391,#32392,#32393,#32394,#32395,#32396,#32397,
#32398,#32399,#32400,#32401,#32402,#32403,#32404,#32405,#32406,#32407,#32408));
#34568=AXIS2_PLACEMENT_3D('',#51564,#39368,#39369);
#34569=AXIS2_PLACEMENT_3D('',#51603,#39370,#39371);
#34570=AXIS2_PLACEMENT_3D('',#51604,#39372,#39373);
#34571=AXIS2_PLACEMENT_3D('',#51705,#39374,#39375);
#34572=AXIS2_PLACEMENT_3D('',#51711,#39379,#39380);
#34573=AXIS2_PLACEMENT_3D('',#51715,#39383,#39384);
#34574=AXIS2_PLACEMENT_3D('',#51719,#39387,#39388);
#34575=AXIS2_PLACEMENT_3D('',#51722,#39389,#39390);
#34576=AXIS2_PLACEMENT_3D('',#51724,#39392,#39393);
#34577=AXIS2_PLACEMENT_3D('',#51747,#39395,#39396);
#34578=AXIS2_PLACEMENT_3D('',#51750,#39397,#39398);
#34579=AXIS2_PLACEMENT_3D('',#51765,#39400,#39401);
#34580=AXIS2_PLACEMENT_3D('',#51786,#39402,#39403);
#34581=AXIS2_PLACEMENT_3D('',#51801,#39405,#39406);
#34582=AXIS2_PLACEMENT_3D('',#51827,#39409,#39410);
#34583=AXIS2_PLACEMENT_3D('',#51851,#39413,#39414);
#34584=AXIS2_PLACEMENT_3D('',#51895,#39417,#39418);
#34585=AXIS2_PLACEMENT_3D('',#51922,#39421,#39422);
#34586=AXIS2_PLACEMENT_3D('',#51928,#39426,#39427);
#34587=AXIS2_PLACEMENT_3D('',#51934,#39431,#39432);
#34588=AXIS2_PLACEMENT_3D('',#51937,#39433,#39434);
#34589=AXIS2_PLACEMENT_3D('',#51951,#39436,#39437);
#34590=AXIS2_PLACEMENT_3D('',#51962,#39438,#39439);
#34591=AXIS2_PLACEMENT_3D('',#51964,#39440,#39441);
#34592=AXIS2_PLACEMENT_3D('',#51965,#39442,#39443);
#34593=AXIS2_PLACEMENT_3D('',#51967,#39444,#39445);
#34594=AXIS2_PLACEMENT_3D('',#51982,#39447,#39448);
#34595=AXIS2_PLACEMENT_3D('',#52009,#39452,#39453);
#34596=AXIS2_PLACEMENT_3D('',#52010,#39454,#39455);
#34597=AXIS2_PLACEMENT_3D('',#52013,#39456,#39457);
#34598=AXIS2_PLACEMENT_3D('',#52015,#39458,#39459);
#34599=AXIS2_PLACEMENT_3D('',#52017,#39460,#39461);
#34600=AXIS2_PLACEMENT_3D('',#52019,#39462,#39463);
#34601=AXIS2_PLACEMENT_3D('',#52021,#39464,#39465);
#34602=AXIS2_PLACEMENT_3D('',#52023,#39466,#39467);
#34603=AXIS2_PLACEMENT_3D('',#52025,#39468,#39469);
#34604=AXIS2_PLACEMENT_3D('',#52027,#39470,#39471);
#34605=AXIS2_PLACEMENT_3D('',#52029,#39472,#39473);
#34606=AXIS2_PLACEMENT_3D('',#52031,#39474,#39475);
#34607=AXIS2_PLACEMENT_3D('',#52033,#39476,#39477);
#34608=AXIS2_PLACEMENT_3D('',#52034,#39478,#39479);
#34609=AXIS2_PLACEMENT_3D('',#52035,#39480,#39481);
#34610=AXIS2_PLACEMENT_3D('',#52038,#39482,#39483);
#34611=AXIS2_PLACEMENT_3D('',#52044,#39487,#39488);
#34612=AXIS2_PLACEMENT_3D('',#52046,#39489,#39490);
#34613=AXIS2_PLACEMENT_3D('',#52050,#39493,#39494);
#34614=AXIS2_PLACEMENT_3D('',#52051,#39495,#39496);
#34615=AXIS2_PLACEMENT_3D('',#52052,#39497,#39498);
#34616=AXIS2_PLACEMENT_3D('',#52054,#39499,#39500);
#34617=AXIS2_PLACEMENT_3D('',#52056,#39502,#39503);
#34618=AXIS2_PLACEMENT_3D('',#52057,#39504,#39505);
#34619=AXIS2_PLACEMENT_3D('',#52060,#39507,#39508);
#34620=AXIS2_PLACEMENT_3D('',#52061,#39509,#39510);
#34621=AXIS2_PLACEMENT_3D('',#52064,#39511,#39512);
#34622=AXIS2_PLACEMENT_3D('',#52070,#39516,#39517);
#34623=AXIS2_PLACEMENT_3D('',#52072,#39518,#39519);
#34624=AXIS2_PLACEMENT_3D('',#52076,#39522,#39523);
#34625=AXIS2_PLACEMENT_3D('',#52078,#39524,#39525);
#34626=AXIS2_PLACEMENT_3D('',#52082,#39528,#39529);
#34627=AXIS2_PLACEMENT_3D('',#52084,#39530,#39531);
#34628=AXIS2_PLACEMENT_3D('',#52088,#39534,#39535);
#34629=AXIS2_PLACEMENT_3D('',#52090,#39536,#39537);
#34630=AXIS2_PLACEMENT_3D('',#52094,#39540,#39541);
#34631=AXIS2_PLACEMENT_3D('',#52096,#39542,#39543);
#34632=AXIS2_PLACEMENT_3D('',#52100,#39546,#39547);
#34633=AXIS2_PLACEMENT_3D('',#52102,#39548,#39549);
#34634=AXIS2_PLACEMENT_3D('',#52106,#39552,#39553);
#34635=AXIS2_PLACEMENT_3D('',#52108,#39554,#39555);
#34636=AXIS2_PLACEMENT_3D('',#52112,#39558,#39559);
#34637=AXIS2_PLACEMENT_3D('',#52114,#39560,#39561);
#34638=AXIS2_PLACEMENT_3D('',#52118,#39564,#39565);
#34639=AXIS2_PLACEMENT_3D('',#52120,#39566,#39567);
#34640=AXIS2_PLACEMENT_3D('',#52124,#39570,#39571);
#34641=AXIS2_PLACEMENT_3D('',#52126,#39572,#39573);
#34642=AXIS2_PLACEMENT_3D('',#52130,#39576,#39577);
#34643=AXIS2_PLACEMENT_3D('',#52131,#39578,#39579);
#34644=AXIS2_PLACEMENT_3D('',#52133,#39581,#39582);
#34645=AXIS2_PLACEMENT_3D('',#52134,#39583,#39584);
#34646=AXIS2_PLACEMENT_3D('',#52135,#39585,#39586);
#34647=AXIS2_PLACEMENT_3D('',#52136,#39587,#39588);
#34648=AXIS2_PLACEMENT_3D('',#52149,#39590,#39591);
#34649=AXIS2_PLACEMENT_3D('',#52152,#39592,#39593);
#34650=AXIS2_PLACEMENT_3D('',#52156,#39595,#39596);
#34651=AXIS2_PLACEMENT_3D('',#52158,#39598,#39599);
#34652=AXIS2_PLACEMENT_3D('',#52164,#39603,#39604);
#34653=AXIS2_PLACEMENT_3D('',#52166,#39605,#39606);
#34654=AXIS2_PLACEMENT_3D('',#52168,#39607,#39608);
#34655=AXIS2_PLACEMENT_3D('',#52170,#39610,#39611);
#34656=AXIS2_PLACEMENT_3D('',#52176,#39615,#39616);
#34657=AXIS2_PLACEMENT_3D('',#52178,#39617,#39618);
#34658=AXIS2_PLACEMENT_3D('',#52180,#39619,#39620);
#34659=AXIS2_PLACEMENT_3D('',#52182,#39622,#39623);
#34660=AXIS2_PLACEMENT_3D('',#52188,#39627,#39628);
#34661=AXIS2_PLACEMENT_3D('',#52190,#39629,#39630);
#34662=AXIS2_PLACEMENT_3D('',#52192,#39631,#39632);
#34663=AXIS2_PLACEMENT_3D('',#52194,#39634,#39635);
#34664=AXIS2_PLACEMENT_3D('',#52197,#39638,#39639);
#34665=AXIS2_PLACEMENT_3D('',#52206,#39644,#39645);
#34666=AXIS2_PLACEMENT_3D('',#52208,#39646,#39647);
#34667=AXIS2_PLACEMENT_3D('',#52210,#39648,#39649);
#34668=AXIS2_PLACEMENT_3D('',#52215,#39651,#39652);
#34669=AXIS2_PLACEMENT_3D('',#52219,#39654,#39655);
#34670=AXIS2_PLACEMENT_3D('',#52223,#39657,#39658);
#34671=AXIS2_PLACEMENT_3D('',#52226,#39660,#39661);
#34672=AXIS2_PLACEMENT_3D('',#52227,#39662,#39663);
#34673=AXIS2_PLACEMENT_3D('',#52231,#39665,#39666);
#34674=AXIS2_PLACEMENT_3D('',#52233,#39668,#39669);
#34675=AXIS2_PLACEMENT_3D('',#52237,#39672,#39673);
#34676=AXIS2_PLACEMENT_3D('',#52239,#39674,#39675);
#34677=AXIS2_PLACEMENT_3D('',#52241,#39677,#39678);
#34678=AXIS2_PLACEMENT_3D('',#52245,#39681,#39682);
#34679=AXIS2_PLACEMENT_3D('',#52247,#39683,#39684);
#34680=AXIS2_PLACEMENT_3D('',#52249,#39686,#39687);
#34681=AXIS2_PLACEMENT_3D('',#52253,#39690,#39691);
#34682=AXIS2_PLACEMENT_3D('',#52255,#39692,#39693);
#34683=AXIS2_PLACEMENT_3D('',#52257,#39695,#39696);
#34684=AXIS2_PLACEMENT_3D('',#52259,#39698,#39699);
#34685=AXIS2_PLACEMENT_3D('',#52260,#39700,#39701);
#34686=AXIS2_PLACEMENT_3D('',#52262,#39702,#39703);
#34687=AXIS2_PLACEMENT_3D('',#52265,#39704,#39705);
#34688=AXIS2_PLACEMENT_3D('',#52267,#39706,#39707);
#34689=AXIS2_PLACEMENT_3D('',#52269,#39708,#39709);
#34690=AXIS2_PLACEMENT_3D('',#52271,#39710,#39711);
#34691=AXIS2_PLACEMENT_3D('',#52273,#39712,#39713);
#34692=AXIS2_PLACEMENT_3D('',#52275,#39714,#39715);
#34693=AXIS2_PLACEMENT_3D('',#52277,#39716,#39717);
#34694=AXIS2_PLACEMENT_3D('',#52279,#39718,#39719);
#34695=AXIS2_PLACEMENT_3D('',#52281,#39720,#39721);
#34696=AXIS2_PLACEMENT_3D('',#52283,#39722,#39723);
#34697=AXIS2_PLACEMENT_3D('',#52285,#39724,#39725);
#34698=AXIS2_PLACEMENT_3D('',#52286,#39726,#39727);
#34699=AXIS2_PLACEMENT_3D('',#52287,#39728,#39729);
#34700=AXIS2_PLACEMENT_3D('',#52289,#39731,#39732);
#34701=AXIS2_PLACEMENT_3D('',#52291,#39733,#39734);
#34702=AXIS2_PLACEMENT_3D('',#52294,#39735,#39736);
#34703=AXIS2_PLACEMENT_3D('',#52296,#39737,#39738);
#34704=AXIS2_PLACEMENT_3D('',#52298,#39739,#39740);
#34705=AXIS2_PLACEMENT_3D('',#52300,#39741,#39742);
#34706=AXIS2_PLACEMENT_3D('',#52302,#39743,#39744);
#34707=AXIS2_PLACEMENT_3D('',#52304,#39745,#39746);
#34708=AXIS2_PLACEMENT_3D('',#52306,#39747,#39748);
#34709=AXIS2_PLACEMENT_3D('',#52308,#39749,#39750);
#34710=AXIS2_PLACEMENT_3D('',#52310,#39751,#39752);
#34711=AXIS2_PLACEMENT_3D('',#52312,#39753,#39754);
#34712=AXIS2_PLACEMENT_3D('',#52314,#39755,#39756);
#34713=AXIS2_PLACEMENT_3D('',#52315,#39757,#39758);
#34714=AXIS2_PLACEMENT_3D('',#52316,#39759,#39760);
#34715=AXIS2_PLACEMENT_3D('',#52318,#39762,#39763);
#34716=AXIS2_PLACEMENT_3D('',#52324,#39767,#39768);
#34717=AXIS2_PLACEMENT_3D('',#52328,#39771,#39772);
#34718=AXIS2_PLACEMENT_3D('',#52332,#39775,#39776);
#34719=AXIS2_PLACEMENT_3D('',#52336,#39779,#39780);
#34720=AXIS2_PLACEMENT_3D('',#52340,#39783,#39784);
#34721=AXIS2_PLACEMENT_3D('',#52344,#39787,#39788);
#34722=AXIS2_PLACEMENT_3D('',#52348,#39791,#39792);
#34723=AXIS2_PLACEMENT_3D('',#52352,#39795,#39796);
#34724=AXIS2_PLACEMENT_3D('',#52356,#39799,#39800);
#34725=AXIS2_PLACEMENT_3D('',#52360,#39803,#39804);
#34726=AXIS2_PLACEMENT_3D('',#52364,#39807,#39808);
#34727=AXIS2_PLACEMENT_3D('',#52366,#39810,#39811);
#34728=AXIS2_PLACEMENT_3D('',#52367,#39812,#39813);
#34729=AXIS2_PLACEMENT_3D('',#52373,#39817,#39818);
#34730=AXIS2_PLACEMENT_3D('',#52377,#39821,#39822);
#34731=AXIS2_PLACEMENT_3D('',#52381,#39825,#39826);
#34732=AXIS2_PLACEMENT_3D('',#52385,#39829,#39830);
#34733=AXIS2_PLACEMENT_3D('',#52389,#39833,#39834);
#34734=AXIS2_PLACEMENT_3D('',#52393,#39837,#39838);
#34735=AXIS2_PLACEMENT_3D('',#52397,#39841,#39842);
#34736=AXIS2_PLACEMENT_3D('',#52401,#39845,#39846);
#34737=AXIS2_PLACEMENT_3D('',#52405,#39849,#39850);
#34738=AXIS2_PLACEMENT_3D('',#52409,#39853,#39854);
#34739=AXIS2_PLACEMENT_3D('',#52413,#39857,#39858);
#34740=AXIS2_PLACEMENT_3D('',#52415,#39860,#39861);
#34741=AXIS2_PLACEMENT_3D('',#52416,#39862,#39863);
#34742=AXIS2_PLACEMENT_3D('',#52434,#39873,#39874);
#34743=AXIS2_PLACEMENT_3D('',#52436,#39876,#39877);
#34744=AXIS2_PLACEMENT_3D('',#52438,#39879,#39880);
#34745=AXIS2_PLACEMENT_3D('',#52440,#39882,#39883);
#34746=AXIS2_PLACEMENT_3D('',#52442,#39885,#39886);
#34747=AXIS2_PLACEMENT_3D('',#52444,#39888,#39889);
#34748=AXIS2_PLACEMENT_3D('',#52446,#39891,#39892);
#34749=AXIS2_PLACEMENT_3D('',#52448,#39894,#39895);
#34750=AXIS2_PLACEMENT_3D('',#52450,#39897,#39898);
#34751=AXIS2_PLACEMENT_3D('',#52451,#39899,#39900);
#34752=AXIS2_PLACEMENT_3D('',#52466,#39903,#39904);
#34753=AXIS2_PLACEMENT_3D('',#52470,#39907,#39908);
#34754=AXIS2_PLACEMENT_3D('',#52471,#39909,#39910);
#34755=AXIS2_PLACEMENT_3D('',#52472,#39911,#39912);
#34756=AXIS2_PLACEMENT_3D('',#52473,#39913,#39914);
#34757=AXIS2_PLACEMENT_3D('',#52474,#39915,#39916);
#34758=AXIS2_PLACEMENT_3D('',#52489,#39919,#39920);
#34759=AXIS2_PLACEMENT_3D('',#52492,#39923,#39924);
#34760=AXIS2_PLACEMENT_3D('',#52493,#39925,#39926);
#34761=AXIS2_PLACEMENT_3D('',#52494,#39927,#39928);
#34762=AXIS2_PLACEMENT_3D('',#52497,#39931,#39932);
#34763=AXIS2_PLACEMENT_3D('',#52498,#39933,#39934);
#34764=AXIS2_PLACEMENT_3D('',#52499,#39935,#39936);
#34765=AXIS2_PLACEMENT_3D('',#52501,#39937,#39938);
#34766=AXIS2_PLACEMENT_3D('',#52503,#39940,#39941);
#34767=AXIS2_PLACEMENT_3D('',#52505,#39943,#39944);
#34768=AXIS2_PLACEMENT_3D('',#52507,#39945,#39946);
#34769=AXIS2_PLACEMENT_3D('',#52508,#39947,#39948);
#34770=AXIS2_PLACEMENT_3D('',#52509,#39949,#39950);
#34771=AXIS2_PLACEMENT_3D('',#52515,#39954,#39955);
#34772=AXIS2_PLACEMENT_3D('',#52519,#39958,#39959);
#34773=AXIS2_PLACEMENT_3D('',#52523,#39962,#39963);
#34774=AXIS2_PLACEMENT_3D('',#52527,#39966,#39967);
#34775=AXIS2_PLACEMENT_3D('',#52531,#39970,#39971);
#34776=AXIS2_PLACEMENT_3D('',#52535,#39974,#39975);
#34777=AXIS2_PLACEMENT_3D('',#52539,#39978,#39979);
#34778=AXIS2_PLACEMENT_3D('',#52543,#39982,#39983);
#34779=AXIS2_PLACEMENT_3D('',#52547,#39986,#39987);
#34780=AXIS2_PLACEMENT_3D('',#52551,#39990,#39991);
#34781=AXIS2_PLACEMENT_3D('',#52555,#39994,#39995);
#34782=AXIS2_PLACEMENT_3D('',#52558,#39997,#39998);
#34783=AXIS2_PLACEMENT_3D('',#52559,#39999,#40000);
#34784=AXIS2_PLACEMENT_3D('',#52560,#40001,#40002);
#34785=AXIS2_PLACEMENT_3D('',#52562,#40004,#40005);
#34786=AXIS2_PLACEMENT_3D('',#52563,#40006,#40007);
#34787=AXIS2_PLACEMENT_3D('',#52565,#40008,#40009);
#34788=AXIS2_PLACEMENT_3D('',#52567,#40010,#40011);
#34789=AXIS2_PLACEMENT_3D('',#52569,#40012,#40013);
#34790=AXIS2_PLACEMENT_3D('',#52571,#40014,#40015);
#34791=AXIS2_PLACEMENT_3D('',#52573,#40016,#40017);
#34792=AXIS2_PLACEMENT_3D('',#52575,#40018,#40019);
#34793=AXIS2_PLACEMENT_3D('',#52577,#40020,#40021);
#34794=AXIS2_PLACEMENT_3D('',#52579,#40022,#40023);
#34795=AXIS2_PLACEMENT_3D('',#52581,#40024,#40025);
#34796=AXIS2_PLACEMENT_3D('',#52582,#40026,#40027);
#34797=AXIS2_PLACEMENT_3D('',#52583,#40028,#40029);
#34798=AXIS2_PLACEMENT_3D('',#52603,#40040,#40041);
#34799=AXIS2_PLACEMENT_3D('',#52605,#40043,#40044);
#34800=AXIS2_PLACEMENT_3D('',#52607,#40046,#40047);
#34801=AXIS2_PLACEMENT_3D('',#52609,#40049,#40050);
#34802=AXIS2_PLACEMENT_3D('',#52611,#40052,#40053);
#34803=AXIS2_PLACEMENT_3D('',#52613,#40055,#40056);
#34804=AXIS2_PLACEMENT_3D('',#52615,#40058,#40059);
#34805=AXIS2_PLACEMENT_3D('',#52617,#40061,#40062);
#34806=AXIS2_PLACEMENT_3D('',#52619,#40064,#40065);
#34807=AXIS2_PLACEMENT_3D('',#52621,#40067,#40068);
#34808=AXIS2_PLACEMENT_3D('',#52622,#40069,#40070);
#34809=AXIS2_PLACEMENT_3D('',#52624,#40071,#40072);
#34810=AXIS2_PLACEMENT_3D('',#52626,#40073,#40074);
#34811=AXIS2_PLACEMENT_3D('',#52627,#40075,#40076);
#34812=AXIS2_PLACEMENT_3D('',#52651,#40078,#40079);
#34813=AXIS2_PLACEMENT_3D('',#52652,#40080,#40081);
#34814=AXIS2_PLACEMENT_3D('',#52671,#40082,#40083);
#34815=AXIS2_PLACEMENT_3D('',#52674,#40084,#40085);
#34816=AXIS2_PLACEMENT_3D('',#52675,#40086,#40087);
#34817=AXIS2_PLACEMENT_3D('',#52676,#40088,#40089);
#34818=AXIS2_PLACEMENT_3D('',#52700,#40091,#40092);
#34819=AXIS2_PLACEMENT_3D('',#52701,#40093,#40094);
#34820=AXIS2_PLACEMENT_3D('',#52720,#40095,#40096);
#34821=AXIS2_PLACEMENT_3D('',#52723,#40097,#40098);
#34822=AXIS2_PLACEMENT_3D('',#52730,#40099,#40100);
#34823=AXIS2_PLACEMENT_3D('',#52731,#40101,#40102);
#34824=AXIS2_PLACEMENT_3D('',#52754,#40104,#40105);
#34825=AXIS2_PLACEMENT_3D('',#52800,#40106,#40107);
#34826=AXIS2_PLACEMENT_3D('',#52801,#40108,#40109);
#34827=AXIS2_PLACEMENT_3D('',#52804,#40110,#40111);
#34828=AXIS2_PLACEMENT_3D('',#52805,#40112,#40113);
#34829=AXIS2_PLACEMENT_3D('',#52833,#40114,#40115);
#34830=AXIS2_PLACEMENT_3D('',#52861,#40116,#40117);
#34831=AXIS2_PLACEMENT_3D('',#52862,#40118,#40119);
#34832=AXIS2_PLACEMENT_3D('',#52865,#40120,#40121);
#34833=AXIS2_PLACEMENT_3D('',#52866,#40122,#40123);
#34834=AXIS2_PLACEMENT_3D('',#52868,#40124,#40125);
#34835=AXIS2_PLACEMENT_3D('',#52869,#40126,#40127);
#34836=AXIS2_PLACEMENT_3D('',#52870,#40128,#40129);
#34837=AXIS2_PLACEMENT_3D('',#52872,#40131,#40132);
#34838=AXIS2_PLACEMENT_3D('',#52873,#40133,#40134);
#34839=AXIS2_PLACEMENT_3D('',#52875,#40135,#40136);
#34840=AXIS2_PLACEMENT_3D('',#52876,#40137,#40138);
#34841=AXIS2_PLACEMENT_3D('',#52880,#40140,#40141);
#34842=AXIS2_PLACEMENT_3D('',#52881,#40142,#40143);
#34843=AXIS2_PLACEMENT_3D('',#52882,#40144,#40145);
#34844=AXIS2_PLACEMENT_3D('',#52885,#40146,#40147);
#34845=AXIS2_PLACEMENT_3D('',#52891,#40151,#40152);
#34846=AXIS2_PLACEMENT_3D('',#52921,#40168,#40169);
#34847=AXIS2_PLACEMENT_3D('',#52923,#40170,#40171);
#34848=AXIS2_PLACEMENT_3D('',#52925,#40173,#40174);
#34849=AXIS2_PLACEMENT_3D('',#52938,#40181,#40182);
#34850=AXIS2_PLACEMENT_3D('',#52951,#40189,#40190);
#34851=AXIS2_PLACEMENT_3D('',#52956,#40192,#40193);
#34852=AXIS2_PLACEMENT_3D('',#52959,#40195,#40196);
#34853=AXIS2_PLACEMENT_3D('',#52962,#40197,#40198);
#34854=AXIS2_PLACEMENT_3D('',#52966,#40200,#40201);
#34855=AXIS2_PLACEMENT_3D('',#52968,#40203,#40204);
#34856=AXIS2_PLACEMENT_3D('',#52971,#40205,#40206);
#34857=AXIS2_PLACEMENT_3D('',#52974,#40209,#40210);
#34858=AXIS2_PLACEMENT_3D('',#52978,#40213,#40214);
#34859=AXIS2_PLACEMENT_3D('',#52980,#40215,#40216);
#34860=AXIS2_PLACEMENT_3D('',#52982,#40218,#40219);
#34861=AXIS2_PLACEMENT_3D('',#52984,#40221,#40222);
#34862=AXIS2_PLACEMENT_3D('',#52989,#40224,#40225);
#34863=AXIS2_PLACEMENT_3D('',#52992,#40227,#40228);
#34864=AXIS2_PLACEMENT_3D('',#52993,#40229,#40230);
#34865=AXIS2_PLACEMENT_3D('',#52994,#40231,#40232);
#34866=AXIS2_PLACEMENT_3D('',#52995,#40233,#40234);
#34867=AXIS2_PLACEMENT_3D('',#52998,#40235,#40236);
#34868=AXIS2_PLACEMENT_3D('',#53001,#40239,#40240);
#34869=AXIS2_PLACEMENT_3D('',#53005,#40243,#40244);
#34870=AXIS2_PLACEMENT_3D('',#53007,#40245,#40246);
#34871=AXIS2_PLACEMENT_3D('',#53009,#40248,#40249);
#34872=AXIS2_PLACEMENT_3D('',#53011,#40251,#40252);
#34873=AXIS2_PLACEMENT_3D('',#53013,#40253,#40254);
#34874=AXIS2_PLACEMENT_3D('',#53014,#40255,#40256);
#34875=AXIS2_PLACEMENT_3D('',#53018,#40258,#40259);
#34876=AXIS2_PLACEMENT_3D('',#53019,#40260,#40261);
#34877=AXIS2_PLACEMENT_3D('',#53020,#40262,#40263);
#34878=AXIS2_PLACEMENT_3D('',#53023,#40265,#40266);
#34879=AXIS2_PLACEMENT_3D('',#53024,#40267,#40268);
#34880=AXIS2_PLACEMENT_3D('',#53026,#40269,#40270);
#34881=AXIS2_PLACEMENT_3D('',#53027,#40271,#40272);
#34882=AXIS2_PLACEMENT_3D('',#53031,#40274,#40275);
#34883=AXIS2_PLACEMENT_3D('',#53032,#40276,#40277);
#34884=AXIS2_PLACEMENT_3D('',#53033,#40278,#40279);
#34885=AXIS2_PLACEMENT_3D('',#53036,#40281,#40282);
#34886=AXIS2_PLACEMENT_3D('',#53037,#40283,#40284);
#34887=AXIS2_PLACEMENT_3D('',#53039,#40285,#40286);
#34888=AXIS2_PLACEMENT_3D('',#53040,#40287,#40288);
#34889=AXIS2_PLACEMENT_3D('',#53044,#40290,#40291);
#34890=AXIS2_PLACEMENT_3D('',#53045,#40292,#40293);
#34891=AXIS2_PLACEMENT_3D('',#53046,#40294,#40295);
#34892=AXIS2_PLACEMENT_3D('',#53049,#40297,#40298);
#34893=AXIS2_PLACEMENT_3D('',#53050,#40299,#40300);
#34894=AXIS2_PLACEMENT_3D('',#53052,#40301,#40302);
#34895=AXIS2_PLACEMENT_3D('',#53053,#40303,#40304);
#34896=AXIS2_PLACEMENT_3D('',#53057,#40306,#40307);
#34897=AXIS2_PLACEMENT_3D('',#53058,#40308,#40309);
#34898=AXIS2_PLACEMENT_3D('',#53059,#40310,#40311);
#34899=AXIS2_PLACEMENT_3D('',#53062,#40313,#40314);
#34900=AXIS2_PLACEMENT_3D('',#53063,#40315,#40316);
#34901=AXIS2_PLACEMENT_3D('',#53066,#40318,#40319);
#34902=AXIS2_PLACEMENT_3D('',#53067,#40320,#40321);
#34903=AXIS2_PLACEMENT_3D('',#53069,#40322,#40323);
#34904=AXIS2_PLACEMENT_3D('',#53071,#40324,#40325);
#34905=AXIS2_PLACEMENT_3D('',#53073,#40326,#40327);
#34906=AXIS2_PLACEMENT_3D('',#53075,#40328,#40329);
#34907=AXIS2_PLACEMENT_3D('',#53077,#40330,#40331);
#34908=AXIS2_PLACEMENT_3D('',#53078,#40332,#40333);
#34909=AXIS2_PLACEMENT_3D('',#53081,#40335,#40336);
#34910=AXIS2_PLACEMENT_3D('',#53082,#40337,#40338);
#34911=AXIS2_PLACEMENT_3D('',#53084,#40339,#40340);
#34912=AXIS2_PLACEMENT_3D('',#53085,#40341,#40342);
#34913=AXIS2_PLACEMENT_3D('',#53088,#40344,#40345);
#34914=AXIS2_PLACEMENT_3D('',#53089,#40346,#40347);
#34915=AXIS2_PLACEMENT_3D('',#53091,#40348,#40349);
#34916=AXIS2_PLACEMENT_3D('',#53092,#40350,#40351);
#34917=AXIS2_PLACEMENT_3D('',#53095,#40353,#40354);
#34918=AXIS2_PLACEMENT_3D('',#53096,#40355,#40356);
#34919=AXIS2_PLACEMENT_3D('',#53098,#40357,#40358);
#34920=AXIS2_PLACEMENT_3D('',#53099,#40359,#40360);
#34921=AXIS2_PLACEMENT_3D('',#53101,#40362,#40363);
#34922=AXIS2_PLACEMENT_3D('',#53103,#40364,#40365);
#34923=AXIS2_PLACEMENT_3D('',#53105,#40366,#40367);
#34924=AXIS2_PLACEMENT_3D('',#53106,#40368,#40369);
#34925=AXIS2_PLACEMENT_3D('',#53108,#40371,#40372);
#34926=AXIS2_PLACEMENT_3D('',#53111,#40374,#40375);
#34927=AXIS2_PLACEMENT_3D('',#53112,#40376,#40377);
#34928=AXIS2_PLACEMENT_3D('',#53113,#40378,#40379);
#34929=AXIS2_PLACEMENT_3D('',#53115,#40380,#40381);
#34930=AXIS2_PLACEMENT_3D('',#53117,#40383,#40384);
#34931=AXIS2_PLACEMENT_3D('',#53119,#40385,#40386);
#34932=AXIS2_PLACEMENT_3D('',#53120,#40387,#40388);
#34933=AXIS2_PLACEMENT_3D('',#53122,#40389,#40390);
#34934=AXIS2_PLACEMENT_3D('',#53124,#40392,#40393);
#34935=AXIS2_PLACEMENT_3D('',#53125,#40394,#40395);
#34936=AXIS2_PLACEMENT_3D('',#53127,#40396,#40397);
#34937=AXIS2_PLACEMENT_3D('',#53128,#40398,#40399);
#34938=AXIS2_PLACEMENT_3D('',#53130,#40400,#40401);
#34939=AXIS2_PLACEMENT_3D('',#53132,#40403,#40404);
#34940=AXIS2_PLACEMENT_3D('',#53134,#40405,#40406);
#34941=AXIS2_PLACEMENT_3D('',#53135,#40407,#40408);
#34942=AXIS2_PLACEMENT_3D('',#53137,#40410,#40411);
#34943=AXIS2_PLACEMENT_3D('',#53139,#40412,#40413);
#34944=AXIS2_PLACEMENT_3D('',#53141,#40415,#40416);
#34945=AXIS2_PLACEMENT_3D('',#53143,#40417,#40418);
#34946=AXIS2_PLACEMENT_3D('',#53144,#40419,#40420);
#34947=AXIS2_PLACEMENT_3D('',#53146,#40421,#40422);
#34948=AXIS2_PLACEMENT_3D('',#53148,#40424,#40425);
#34949=AXIS2_PLACEMENT_3D('',#53149,#40426,#40427);
#34950=AXIS2_PLACEMENT_3D('',#53159,#40433,#40434);
#34951=AXIS2_PLACEMENT_3D('',#53163,#40436,#40437);
#34952=AXIS2_PLACEMENT_3D('',#53164,#40438,#40439);
#34953=AXIS2_PLACEMENT_3D('',#53165,#40440,#40441);
#34954=AXIS2_PLACEMENT_3D('',#53172,#40446,#40447);
#34955=AXIS2_PLACEMENT_3D('',#53173,#40448,#40449);
#34956=AXIS2_PLACEMENT_3D('',#53174,#40450,#40451);
#34957=AXIS2_PLACEMENT_3D('',#53176,#40452,#40453);
#34958=AXIS2_PLACEMENT_3D('',#53177,#40454,#40455);
#34959=AXIS2_PLACEMENT_3D('',#53178,#40456,#40457);
#34960=AXIS2_PLACEMENT_3D('',#53179,#40458,#40459);
#34961=AXIS2_PLACEMENT_3D('',#53180,#40460,#40461);
#34962=AXIS2_PLACEMENT_3D('',#53181,#40462,#40463);
#34963=AXIS2_PLACEMENT_3D('',#53182,#40464,#40465);
#34964=AXIS2_PLACEMENT_3D('',#53184,#40466,#40467);
#34965=AXIS2_PLACEMENT_3D('',#53185,#40468,#40469);
#34966=AXIS2_PLACEMENT_3D('',#53186,#40470,#40471);
#34967=AXIS2_PLACEMENT_3D('',#53187,#40472,#40473);
#34968=AXIS2_PLACEMENT_3D('',#53188,#40474,#40475);
#34969=AXIS2_PLACEMENT_3D('',#53191,#40477,#40478);
#34970=AXIS2_PLACEMENT_3D('',#53192,#40479,#40480);
#34971=AXIS2_PLACEMENT_3D('',#53193,#40481,#40482);
#34972=AXIS2_PLACEMENT_3D('',#53196,#40483,#40484);
#34973=AXIS2_PLACEMENT_3D('',#53198,#40485,#40486);
#34974=AXIS2_PLACEMENT_3D('',#53200,#40487,#40488);
#34975=AXIS2_PLACEMENT_3D('',#53202,#40489,#40490);
#34976=AXIS2_PLACEMENT_3D('',#53204,#40491,#40492);
#34977=AXIS2_PLACEMENT_3D('',#53206,#40493,#40494);
#34978=AXIS2_PLACEMENT_3D('',#53208,#40495,#40496);
#34979=AXIS2_PLACEMENT_3D('',#53210,#40497,#40498);
#34980=AXIS2_PLACEMENT_3D('',#53211,#40499,#40500);
#34981=AXIS2_PLACEMENT_3D('',#53213,#40501,#40502);
#34982=AXIS2_PLACEMENT_3D('',#53215,#40503,#40504);
#34983=AXIS2_PLACEMENT_3D('',#53217,#40505,#40506);
#34984=AXIS2_PLACEMENT_3D('',#53219,#40507,#40508);
#34985=AXIS2_PLACEMENT_3D('',#53220,#40509,#40510);
#34986=AXIS2_PLACEMENT_3D('',#53221,#40511,#40512);
#34987=AXIS2_PLACEMENT_3D('',#53222,#40513,#40514);
#34988=AXIS2_PLACEMENT_3D('',#53224,#40515,#40516);
#34989=AXIS2_PLACEMENT_3D('',#53225,#40517,#40518);
#34990=AXIS2_PLACEMENT_3D('',#53227,#40520,#40521);
#34991=AXIS2_PLACEMENT_3D('',#53228,#40522,#40523);
#34992=AXIS2_PLACEMENT_3D('',#53229,#40524,#40525);
#34993=AXIS2_PLACEMENT_3D('',#53232,#40526,#40527);
#34994=AXIS2_PLACEMENT_3D('',#53234,#40528,#40529);
#34995=AXIS2_PLACEMENT_3D('',#53236,#40530,#40531);
#34996=AXIS2_PLACEMENT_3D('',#53238,#40532,#40533);
#34997=AXIS2_PLACEMENT_3D('',#53240,#40534,#40535);
#34998=AXIS2_PLACEMENT_3D('',#53242,#40536,#40537);
#34999=AXIS2_PLACEMENT_3D('',#53244,#40538,#40539);
#35000=AXIS2_PLACEMENT_3D('',#53246,#40540,#40541);
#35001=AXIS2_PLACEMENT_3D('',#53248,#40542,#40543);
#35002=AXIS2_PLACEMENT_3D('',#53250,#40544,#40545);
#35003=AXIS2_PLACEMENT_3D('',#53252,#40546,#40547);
#35004=AXIS2_PLACEMENT_3D('',#53254,#40548,#40549);
#35005=AXIS2_PLACEMENT_3D('',#53256,#40550,#40551);
#35006=AXIS2_PLACEMENT_3D('',#53258,#40552,#40553);
#35007=AXIS2_PLACEMENT_3D('',#53260,#40554,#40555);
#35008=AXIS2_PLACEMENT_3D('',#53261,#40556,#40557);
#35009=AXIS2_PLACEMENT_3D('',#53262,#40558,#40559);
#35010=AXIS2_PLACEMENT_3D('',#53268,#40563,#40564);
#35011=AXIS2_PLACEMENT_3D('',#53272,#40567,#40568);
#35012=AXIS2_PLACEMENT_3D('',#53276,#40571,#40572);
#35013=AXIS2_PLACEMENT_3D('',#53280,#40575,#40576);
#35014=AXIS2_PLACEMENT_3D('',#53284,#40579,#40580);
#35015=AXIS2_PLACEMENT_3D('',#53288,#40583,#40584);
#35016=AXIS2_PLACEMENT_3D('',#53292,#40587,#40588);
#35017=AXIS2_PLACEMENT_3D('',#53296,#40591,#40592);
#35018=AXIS2_PLACEMENT_3D('',#53300,#40595,#40596);
#35019=AXIS2_PLACEMENT_3D('',#53304,#40599,#40600);
#35020=AXIS2_PLACEMENT_3D('',#53308,#40603,#40604);
#35021=AXIS2_PLACEMENT_3D('',#53312,#40607,#40608);
#35022=AXIS2_PLACEMENT_3D('',#53316,#40611,#40612);
#35023=AXIS2_PLACEMENT_3D('',#53320,#40615,#40616);
#35024=AXIS2_PLACEMENT_3D('',#53324,#40619,#40620);
#35025=AXIS2_PLACEMENT_3D('',#53326,#40622,#40623);
#35026=AXIS2_PLACEMENT_3D('',#53327,#40624,#40625);
#35027=AXIS2_PLACEMENT_3D('',#53329,#40627,#40628);
#35028=AXIS2_PLACEMENT_3D('',#53331,#40630,#40631);
#35029=AXIS2_PLACEMENT_3D('',#53333,#40633,#40634);
#35030=AXIS2_PLACEMENT_3D('',#53335,#40636,#40637);
#35031=AXIS2_PLACEMENT_3D('',#53337,#40639,#40640);
#35032=AXIS2_PLACEMENT_3D('',#53339,#40642,#40643);
#35033=AXIS2_PLACEMENT_3D('',#53341,#40645,#40646);
#35034=AXIS2_PLACEMENT_3D('',#53343,#40648,#40649);
#35035=AXIS2_PLACEMENT_3D('',#53345,#40651,#40652);
#35036=AXIS2_PLACEMENT_3D('',#53347,#40654,#40655);
#35037=AXIS2_PLACEMENT_3D('',#53349,#40657,#40658);
#35038=AXIS2_PLACEMENT_3D('',#53351,#40660,#40661);
#35039=AXIS2_PLACEMENT_3D('',#53353,#40663,#40664);
#39368=DIRECTION('axis',(0.,0.,1.));
#39369=DIRECTION('refdir',(1.,0.,0.));
#39370=DIRECTION('center_axis',(-0.857167300702049,-0.515038074910159,2.44576428750191E-14));
#39371=DIRECTION('ref_axis',(-0.515038074910159,0.857167300702049,-3.63131968870903E-14));
#39372=DIRECTION('center_axis',(-0.857167300702049,-0.515038074910159,2.44576428750191E-14));
#39373=DIRECTION('ref_axis',(-0.515038074910159,0.857167300702049,-3.63131968870903E-14));
#39374=DIRECTION('center_axis',(2.77102527463854E-15,8.5557679050281E-15,
1.));
#39375=DIRECTION('ref_axis',(-6.7618653731838E-14,1.,-8.55576790502791E-15));
#39376=DIRECTION('',(0.857167300702075,0.515038074910116,-6.78177848602257E-15));
#39377=DIRECTION('',(-0.515038074910087,0.857167300702093,-5.90654095760951E-15));
#39378=DIRECTION('',(0.8571673007021,0.515038074910075,-6.78177848602229E-15));
#39379=DIRECTION('center_axis',(-0.515038074910103,0.857167300702083,-5.90654095760938E-15));
#39380=DIRECTION('ref_axis',(-2.77102527463854E-15,-8.5557679050281E-15,
-1.));
#39381=DIRECTION('',(-2.77102527463854E-15,-8.5557679050281E-15,-1.));
#39382=DIRECTION('',(0.85716730070209,0.515038074910091,-6.7817784860224E-15));
#39383=DIRECTION('center_axis',(-2.77102527463854E-15,-8.5557679050281E-15,
-1.));
#39384=DIRECTION('ref_axis',(6.7618653731838E-14,-1.,8.55576790502791E-15));
#39385=DIRECTION('',(0.51503807491012,-0.857167300702073,5.90654095760924E-15));
#39386=DIRECTION('',(0.857167300702092,0.515038074910088,-6.78177848602238E-15));
#39387=DIRECTION('center_axis',(-0.857167300702051,-0.515038074910156,6.78177848602285E-15));
#39388=DIRECTION('ref_axis',(2.77102527463854E-15,8.5557679050281E-15,1.));
#39389=DIRECTION('center_axis',(-0.857167300702059,-0.515038074910142,1.20908994046383E-14));
#39390=DIRECTION('ref_axis',(0.515038074910142,-0.857167300702059,1.31876972665472E-13));
#39391=DIRECTION('',(-2.77102527463854E-15,-8.5557679050281E-15,-1.));
#39392=DIRECTION('center_axis',(0.857167300702053,0.515038074910153,-7.55127991844926E-15));
#39393=DIRECTION('ref_axis',(0.515038074910153,-0.857167300702053,5.90654095760898E-15));
#39394=DIRECTION('',(-0.857167300702053,-0.515038074910153,7.55127991844926E-15));
#39395=DIRECTION('center_axis',(-5.19067754597624E-15,-4.44287817572889E-15,
-1.));
#39396=DIRECTION('ref_axis',(0.861906247151903,0.507067669172983,-6.72671728481439E-15));
#39397=DIRECTION('center_axis',(-2.77102527463854E-15,-8.5557679050281E-15,
-1.));
#39398=DIRECTION('ref_axis',(0.91847083292034,0.395488721804576,-5.92881560485675E-15));
#39399=DIRECTION('',(2.77102527463854E-15,8.5557679050281E-15,1.));
#39400=DIRECTION('center_axis',(3.22934968323309E-13,1.72787305786163E-13,
-1.));
#39401=DIRECTION('ref_axis',(0.885014263114158,0.465563909774484,3.66245586665653E-13));
#39402=DIRECTION('center_axis',(2.77102527463854E-15,8.5557679050281E-15,
1.));
#39403=DIRECTION('ref_axis',(0.861906247151891,0.507067669173004,-6.72671728481454E-15));
#39404=DIRECTION('',(2.77102527463854E-15,8.5557679050281E-15,1.));
#39405=DIRECTION('center_axis',(-4.25208859581478E-13,-2.05700297011475E-13,
-1.));
#39406=DIRECTION('ref_axis',(0.918470832920341,0.395488721804574,-4.71894082964798E-13));
#39407=DIRECTION('',(2.77102527463854E-15,8.5557679050281E-15,1.));
#39408=DIRECTION('',(-2.77102527463854E-15,-8.5557679050281E-15,-1.));
#39409=DIRECTION('center_axis',(-1.,-6.7618653731838E-14,2.77102527463912E-15));
#39410=DIRECTION('ref_axis',(-2.77102527463854E-15,-8.5557679050281E-15,
-1.));
#39411=DIRECTION('',(1.,6.7618653731838E-14,-2.77102527463912E-15));
#39412=DIRECTION('',(1.,6.7618653731838E-14,-2.77102527463912E-15));
#39413=DIRECTION('center_axis',(-1.,-6.7618653731838E-14,2.77102527463912E-15));
#39414=DIRECTION('ref_axis',(2.77102527463841E-15,1.04984153671894E-14,
1.));
#39415=DIRECTION('',(1.,6.7618653731838E-14,-2.77102527463912E-15));
#39416=DIRECTION('',(1.,6.7618653731838E-14,-2.77102527463912E-15));
#39417=DIRECTION('center_axis',(-1.,-6.7618653731838E-14,2.77102527463912E-15));
#39418=DIRECTION('ref_axis',(6.7618653731838E-14,-1.,8.55576790502791E-15));
#39419=DIRECTION('',(-1.,-6.7618653731838E-14,2.77102527463912E-15));
#39420=DIRECTION('',(1.,6.7618653731838E-14,-2.77102527463912E-15));
#39421=DIRECTION('center_axis',(6.7618653731838E-14,-1.,8.55576790502791E-15));
#39422=DIRECTION('ref_axis',(2.77102527463854E-15,8.5557679050281E-15,1.));
#39423=DIRECTION('',(2.77102527463854E-15,8.5557679050281E-15,1.));
#39424=DIRECTION('',(1.,6.7618653731838E-14,-2.77102527463912E-15));
#39425=DIRECTION('',(-2.77102527463854E-15,-8.5557679050281E-15,-1.));
#39426=DIRECTION('center_axis',(-6.7618653731838E-14,1.,-8.55576790502791E-15));
#39427=DIRECTION('ref_axis',(-2.77102527463854E-15,-8.5557679050281E-15,
-1.));
#39428=DIRECTION('',(1.,6.7618653731838E-14,-2.77102527463912E-15));
#39429=DIRECTION('',(1.,6.7618653731838E-14,-2.77102527463912E-15));
#39430=DIRECTION('',(-2.77102527463854E-15,-8.5557679050281E-15,-1.));
#39431=DIRECTION('center_axis',(-0.85716730070211,0.515038074910058,-2.11149495005192E-14));
#39432=DIRECTION('ref_axis',(0.515038074910058,0.85716730070211,-8.76090800356362E-15));
#39433=DIRECTION('center_axis',(0.857167300702118,-0.515038074910045,-9.73848807776743E-16));
#39434=DIRECTION('ref_axis',(0.515038074910045,0.857167300702118,-1.31047159934894E-14));
#39435=DIRECTION('',(0.85716730070211,-0.515038074910058,2.11149495005192E-14));
#39436=DIRECTION('center_axis',(0.85716730070212,-0.515038074910041,-1.95197940709233E-15));
#39437=DIRECTION('ref_axis',(0.515038074910041,0.85716730070212,2.09861197125113E-15));
#39438=DIRECTION('center_axis',(1.64678176605324E-15,8.08403097159972E-16,
-1.));
#39439=DIRECTION('ref_axis',(0.918470832920391,-0.395488721804457,1.19280671270647E-15));
#39440=DIRECTION('center_axis',(4.19666809032036E-13,-2.05700297011328E-13,
-1.));
#39441=DIRECTION('ref_axis',(0.893066438469014,-0.449924812030044,4.67340009953242E-13));
#39442=DIRECTION('center_axis',(2.77102527463854E-15,8.5557679050281E-15,
1.));
#39443=DIRECTION('ref_axis',(0.885014263114177,-0.465563909774447,1.53085986548262E-15));
#39444=DIRECTION('center_axis',(3.22934968323738E-13,-1.898988415964E-13,
-1.));
#39445=DIRECTION('ref_axis',(0.861906247151989,-0.507067669172838,3.74631229608968E-13));
#39446=DIRECTION('',(-2.77102527463854E-15,-8.5557679050281E-15,-1.));
#39447=DIRECTION('center_axis',(5.00337040136837E-14,-3.31988340433105E-14,
-1.));
#39448=DIRECTION('ref_axis',(0.893066438469019,-0.449924812030035,5.96204010134664E-14));
#39449=DIRECTION('',(2.77102527463854E-15,8.5557679050281E-15,1.));
#39450=DIRECTION('',(2.77102527463854E-15,8.5557679050281E-15,1.));
#39451=DIRECTION('',(2.77102527463854E-15,8.5557679050281E-15,1.));
#39452=DIRECTION('center_axis',(-0.85716730070212,0.515038074910041,-2.03131397634351E-15));
#39453=DIRECTION('ref_axis',(-2.77102527463854E-15,-8.5557679050281E-15,
-1.));
#39454=DIRECTION('center_axis',(-7.09168149328433E-14,1.,0.));
#39455=DIRECTION('ref_axis',(0.,-8.86460186660541E-15,-1.));
#39456=DIRECTION('center_axis',(-0.515038074912743,-0.857167300700497,6.99406836105656E-14));
#39457=DIRECTION('ref_axis',(0.857167300700497,-0.515038074912743,-7.69635029986347E-14));
#39458=DIRECTION('center_axis',(5.4143828599301E-14,-4.58060313724235E-14,
1.));
#39459=DIRECTION('ref_axis',(0.813525514741032,-0.581529222709692,-7.06849318507178E-14));
#39460=DIRECTION('center_axis',(-0.515038074910113,-0.857167300702077,-4.75968469660724E-14));
#39461=DIRECTION('ref_axis',(0.765900867954103,-0.460199669632744,0.449012387955015));
#39462=DIRECTION('center_axis',(2.77102527463854E-15,8.5557679050281E-15,
1.));
#39463=DIRECTION('ref_axis',(0.89942493888384,-0.43707525589285,1.24718520816265E-15));
#39464=DIRECTION('center_axis',(0.515038074910163,0.857167300702047,7.80464133895757E-14));
#39465=DIRECTION('ref_axis',(0.854456218440598,-0.513409092344321,0.0794712191071334));
#39466=DIRECTION('center_axis',(2.77102527463854E-15,8.5557679050281E-15,
1.));
#39467=DIRECTION('ref_axis',(0.997159343857271,-0.0753209330673478,-2.1187253229561E-15));
#39468=DIRECTION('center_axis',(0.515038074910056,0.857167300702111,-8.76090800356364E-15));
#39469=DIRECTION('ref_axis',(0.853796957819509,-0.513012968599281,-0.0885914717515463));
#39470=DIRECTION('center_axis',(-2.77102527463854E-15,-8.5557679050281E-15,
-1.));
#39471=DIRECTION('ref_axis',(0.895386922140334,-0.44528896197869,1.32864921752887E-15));
#39472=DIRECTION('center_axis',(0.515038074910152,0.857167300702054,-9.20691349666037E-14));
#39473=DIRECTION('ref_axis',(0.765900867954062,-0.460199669632791,-0.449012387955036));
#39474=DIRECTION('center_axis',(3.34893569077092E-13,-2.11445125090906E-13,
-1.));
#39475=DIRECTION('ref_axis',(0.808168976755185,-0.588950681305725,3.95181343523989E-13));
#39476=DIRECTION('center_axis',(-0.515038074910049,-0.857167300702115,4.43474428456801E-14));
#39477=DIRECTION('ref_axis',(0.854456218440674,-0.513409092344209,-0.0794712191070315));
#39478=DIRECTION('center_axis',(-5.41438285993037E-14,4.58060313724264E-14,
-1.));
#39479=DIRECTION('ref_axis',(0.534642392051038,-0.845078406197877,-6.76572740235932E-14));
#39480=DIRECTION('center_axis',(-2.77102527463854E-15,-8.5557679050281E-15,
-1.));
#39481=DIRECTION('ref_axis',(6.7618653731838E-14,-1.,8.55576790502791E-15));
#39482=DIRECTION('center_axis',(2.77102527463854E-15,8.5557679050281E-15,
1.));
#39483=DIRECTION('ref_axis',(0.895386922140312,0.445288961978735,-6.29092880119255E-15));
#39484=DIRECTION('',(0.857167300702098,0.515038074910078,-6.78177848602231E-15));
#39485=DIRECTION('',(0.51503807491012,-0.857167300702073,5.90654095760924E-15));
#39486=DIRECTION('',(0.857167300702087,0.515038074910096,-6.78177848602243E-15));
#39487=DIRECTION('center_axis',(-0.515038074910065,0.857167300702106,-5.90654095760967E-15));
#39488=DIRECTION('ref_axis',(-2.77102527463854E-15,-8.5557679050281E-15,
-1.));
#39489=DIRECTION('center_axis',(0.515038074910833,-0.857167300701645,3.31402177757022E-14));
#39490=DIRECTION('ref_axis',(0.857167300701645,0.515038074910833,1.33541552527618E-14));
#39491=DIRECTION('',(0.857167300702098,0.515038074910078,-6.78177848602231E-15));
#39492=DIRECTION('',(-2.77102527463854E-15,-8.5557679050281E-15,-1.));
#39493=DIRECTION('center_axis',(-0.857167300702058,-0.515038074910145,3.72458084698414E-15));
#39494=DIRECTION('ref_axis',(2.65998341932259E-15,2.80470534102394E-15,
1.));
#39495=DIRECTION('center_axis',(-0.857167300702053,-0.515038074910153,-1.03164475269556E-15));
#39496=DIRECTION('ref_axis',(0.515038074910153,-0.857167300702053,2.11098689223494E-14));
#39497=DIRECTION('center_axis',(0.85716730070204,0.515038074910174,1.1501575548429E-14));
#39498=DIRECTION('ref_axis',(0.515038074910174,-0.85716730070204,5.90654095760881E-15));
#39499=DIRECTION('center_axis',(-0.85716730070205,-0.515038074910157,9.93521908124291E-15));
#39500=DIRECTION('ref_axis',(0.515038074910157,-0.85716730070205,1.67660609324238E-14));
#39501=DIRECTION('',(-0.85716730070204,-0.515038074910174,-1.1501575548429E-14));
#39502=DIRECTION('center_axis',(-0.857167300702099,0.515038074910076,-2.54241575221074E-14));
#39503=DIRECTION('ref_axis',(0.515038074910076,0.857167300702099,-8.7609080035636E-15));
#39504=DIRECTION('center_axis',(0.85716730070211,-0.515038074910058,1.38516209272139E-14));
#39505=DIRECTION('ref_axis',(0.515038074910058,0.85716730070211,1.64991411593497E-13));
#39506=DIRECTION('',(0.857167300702099,-0.515038074910076,2.54241575221073E-14));
#39507=DIRECTION('center_axis',(0.85716730070212,-0.515038074910041,-1.95197940709221E-15));
#39508=DIRECTION('ref_axis',(0.515038074910041,0.85716730070212,3.03333639057696E-14));
#39509=DIRECTION('center_axis',(2.77102527463854E-15,8.5557679050281E-15,
1.));
#39510=DIRECTION('ref_axis',(-6.7618653731838E-14,1.,-8.55576790502791E-15));
#39511=DIRECTION('center_axis',(1.41462354879372E-13,-4.82321162475789E-14,
-1.));
#39512=DIRECTION('ref_axis',(0.895386922140315,-0.445288961978728,1.48140771512084E-13));
#39513=DIRECTION('',(0.857167300702158,-0.515038074909978,2.03131397634287E-15));
#39514=DIRECTION('',(0.515038074909971,0.857167300702162,-8.76090800356383E-15));
#39515=DIRECTION('',(0.857167300702148,-0.515038074909994,2.03131397634304E-15));
#39516=DIRECTION('center_axis',(-0.515038074909966,-0.857167300702166,8.76090800356385E-15));
#39517=DIRECTION('ref_axis',(2.77102527463854E-15,8.5557679050281E-15,1.));
#39518=DIRECTION('center_axis',(0.515038074910056,0.857167300702111,-8.76090800356364E-15));
#39519=DIRECTION('ref_axis',(0.853796957819509,-0.513012968599281,-0.0885914717515493));
#39520=DIRECTION('',(0.857167300702158,-0.515038074909978,2.03131397634287E-15));
#39521=DIRECTION('',(2.77102527463854E-15,8.5557679050281E-15,1.));
#39522=DIRECTION('center_axis',(-2.77102527463854E-15,-8.5557679050281E-15,
-1.));
#39523=DIRECTION('ref_axis',(6.7618653731838E-14,-1.,8.55576790502791E-15));
#39524=DIRECTION('center_axis',(2.77102527463854E-15,8.5557679050281E-15,
1.));
#39525=DIRECTION('ref_axis',(0.997159343857267,-0.0753209330674082,-2.11872532295557E-15));
#39526=DIRECTION('',(0.857167300702159,-0.515038074909977,2.03131397634286E-15));
#39527=DIRECTION('',(-0.515038074909971,-0.857167300702162,8.76090800356383E-15));
#39528=DIRECTION('center_axis',(-0.515038074910013,-0.857167300702137,8.76090800356374E-15));
#39529=DIRECTION('ref_axis',(2.77102527463854E-15,8.5557679050281E-15,1.));
#39530=DIRECTION('center_axis',(0.515038074910268,0.857167300701984,9.11494052980619E-14));
#39531=DIRECTION('ref_axis',(0.854456218440525,-0.513409092344421,0.079471219107265));
#39532=DIRECTION('',(0.857167300702156,-0.515038074909982,2.03131397634291E-15));
#39533=DIRECTION('',(2.77102527463854E-15,8.5557679050281E-15,1.));
#39534=DIRECTION('center_axis',(-2.77102527463854E-15,-8.5557679050281E-15,
-1.));
#39535=DIRECTION('ref_axis',(6.7618653731838E-14,-1.,8.55576790502791E-15));
#39536=DIRECTION('center_axis',(6.78100213977318E-13,-3.9722294646622E-13,
1.));
#39537=DIRECTION('ref_axis',(0.899424938883905,-0.437075255892716,-7.83516564486894E-13));
#39538=DIRECTION('',(0.857167300702151,-0.515038074909989,2.03131397634299E-15));
#39539=DIRECTION('',(-0.515038074909941,-0.85716730070218,8.76090800356391E-15));
#39540=DIRECTION('center_axis',(0.515038074909992,0.85716730070215,-8.76090800356379E-15));
#39541=DIRECTION('ref_axis',(-2.77102527463854E-15,-8.5557679050281E-15,
-1.));
#39542=DIRECTION('center_axis',(-0.515038074910134,-0.857167300702064,-5.44461381909585E-14));
#39543=DIRECTION('ref_axis',(0.765900867954141,-0.460199669632797,0.449012387954897));
#39544=DIRECTION('',(0.857167300702159,-0.515038074909977,2.03131397634286E-15));
#39545=DIRECTION('',(-2.77102527463854E-15,-8.5557679050281E-15,-1.));
#39546=DIRECTION('center_axis',(-2.77102527463854E-15,-8.5557679050281E-15,
-1.));
#39547=DIRECTION('ref_axis',(6.7618653731838E-14,-1.,8.55576790502791E-15));
#39548=DIRECTION('center_axis',(2.77102527463854E-15,8.5557679050281E-15,
1.));
#39549=DIRECTION('ref_axis',(0.813525514741016,-0.581529222709715,2.72112929658504E-15));
#39550=DIRECTION('',(0.857167300702151,-0.51503807490999,2.031313976343E-15));
#39551=DIRECTION('',(-0.515038074910003,-0.857167300702143,8.76090800356376E-15));
#39552=DIRECTION('center_axis',(0.51503807490998,0.857167300702157,-8.76090800356381E-15));
#39553=DIRECTION('ref_axis',(-2.77102527463854E-15,-8.5557679050281E-15,
-1.));
#39554=DIRECTION('center_axis',(-0.515038074909266,-0.857167300702586,-2.04247301180779E-15));
#39555=DIRECTION('ref_axis',(0.857167300702586,-0.515038074909266,7.947721297203E-14));
#39556=DIRECTION('',(0.857167300702151,-0.51503807490999,2.031313976343E-15));
#39557=DIRECTION('',(-2.77102527463854E-15,-8.5557679050281E-15,-1.));
#39558=DIRECTION('center_axis',(2.77102527463854E-15,8.5557679050281E-15,
1.));
#39559=DIRECTION('ref_axis',(-6.7618653731838E-14,1.,-8.55576790502791E-15));
#39560=DIRECTION('center_axis',(-2.77102527463854E-15,-8.5557679050281E-15,
-1.));
#39561=DIRECTION('ref_axis',(0.534642392051038,-0.845078406197877,5.74878712371346E-15));
#39562=DIRECTION('',(0.857167300702159,-0.515038074909977,2.03131397634286E-15));
#39563=DIRECTION('',(0.515038074909973,0.857167300702161,-8.76090800356383E-15));
#39564=DIRECTION('center_axis',(0.515038074909992,0.85716730070215,-1.83469634573233E-15));
#39565=DIRECTION('ref_axis',(-2.65430854586528E-15,-5.45548554721672E-16,
-1.));
#39566=DIRECTION('center_axis',(-0.515038074910081,-0.857167300702096,5.46958285005906E-14));
#39567=DIRECTION('ref_axis',(0.854456218440659,-0.513409092344244,-0.0794712191069747));
#39568=DIRECTION('',(0.857167300702151,-0.515038074909989,2.03131397634299E-15));
#39569=DIRECTION('',(-2.77102527463854E-15,-8.5557679050281E-15,-1.));
#39570=DIRECTION('center_axis',(2.77102527463854E-15,8.5557679050281E-15,
1.));
#39571=DIRECTION('ref_axis',(-6.7618653731838E-14,1.,-8.55576790502791E-15));
#39572=DIRECTION('center_axis',(-2.77102527463854E-15,-8.5557679050281E-15,
-1.));
#39573=DIRECTION('ref_axis',(0.808168976755134,-0.588950681305795,2.79946867599331E-15));
#39574=DIRECTION('',(0.857167300702156,-0.515038074909982,2.03131397634291E-15));
#39575=DIRECTION('',(0.515038074909941,0.85716730070218,-8.76090800356391E-15));
#39576=DIRECTION('center_axis',(-0.515038074909963,-0.857167300702167,8.76090800356385E-15));
#39577=DIRECTION('ref_axis',(2.77102527463854E-15,8.5557679050281E-15,1.));
#39578=DIRECTION('center_axis',(0.515038074910184,0.857167300702034,-1.02454745030335E-13));
#39579=DIRECTION('ref_axis',(0.765900867954022,-0.460199669632811,-0.449012387955084));
#39580=DIRECTION('',(2.77102527463854E-15,8.5557679050281E-15,1.));
#39581=DIRECTION('center_axis',(0.857167300702158,-0.515038074909979,2.03131397634288E-15));
#39582=DIRECTION('ref_axis',(2.77102527463854E-15,8.5557679050281E-15,1.));
#39583=DIRECTION('center_axis',(-7.09168149328348E-14,1.,0.));
#39584=DIRECTION('ref_axis',(0.,-8.86460186660431E-15,-1.));
#39585=DIRECTION('center_axis',(-0.85716730070212,0.515038074910041,-2.03131397634351E-15));
#39586=DIRECTION('ref_axis',(-2.77102527463854E-15,-8.5557679050281E-15,
-1.));
#39587=DIRECTION('center_axis',(-1.,-6.7618653731838E-14,2.77102527463912E-15));
#39588=DIRECTION('ref_axis',(-6.7618653731838E-14,1.,-9.47596933447271E-15));
#39589=DIRECTION('',(-1.,-6.7618653731838E-14,2.77102527463912E-15));
#39590=DIRECTION('center_axis',(1.,6.7618653731838E-14,-2.77102527463912E-15));
#39591=DIRECTION('ref_axis',(-2.77102527463854E-15,-8.5557679050281E-15,
-1.));
#39592=DIRECTION('center_axis',(-1.,-6.7618653731838E-14,2.77102527463912E-15));
#39593=DIRECTION('ref_axis',(-2.77102527463873E-15,-5.7951636166937E-15,
-1.));
#39594=DIRECTION('',(-1.,-6.7618653731838E-14,2.77102527463912E-15));
#39595=DIRECTION('center_axis',(-1.,-6.7618653731838E-14,2.77102527463912E-15));
#39596=DIRECTION('ref_axis',(-2.77102527463873E-15,-5.7951636166937E-15,
-1.));
#39597=DIRECTION('',(-1.,-6.7618653731838E-14,2.77102527463912E-15));
#39598=DIRECTION('center_axis',(-2.77102527463854E-15,-8.5557679050281E-15,
-1.));
#39599=DIRECTION('ref_axis',(6.7618653731838E-14,-1.,8.55576790502791E-15));
#39600=DIRECTION('',(6.7618653731838E-14,-1.,8.55576790502791E-15));
#39601=DIRECTION('',(6.7618653731838E-14,-1.,8.55576790502791E-15));
#39602=DIRECTION('',(-1.,-6.7618653731838E-14,2.77102527463912E-15));
#39603=DIRECTION('center_axis',(1.,6.7618653731838E-14,-2.77102527463912E-15));
#39604=DIRECTION('ref_axis',(6.7618653731838E-14,-1.,9.01586861975031E-15));
#39605=DIRECTION('center_axis',(-1.,-7.65049048161611E-14,-6.11522580968364E-15));
#39606=DIRECTION('ref_axis',(7.6504904816161E-14,-1.,1.91380843436431E-14));
#39607=DIRECTION('center_axis',(-1.,-7.6504904816161E-14,-6.11522580968382E-15));
#39608=DIRECTION('ref_axis',(7.6504904816161E-14,-1.,9.47596933447271E-15));
#39609=DIRECTION('',(-1.,-6.7618653731838E-14,2.77102527463912E-15));
#39610=DIRECTION('center_axis',(6.7618653731838E-14,-1.,8.55576790502791E-15));
#39611=DIRECTION('ref_axis',(2.77102527463854E-15,8.5557679050281E-15,1.));
#39612=DIRECTION('',(2.77102527463854E-15,8.5557679050281E-15,1.));
#39613=DIRECTION('',(2.77102527463854E-15,8.5557679050281E-15,1.));
#39614=DIRECTION('',(-1.,-6.7618653731838E-14,2.77102527463912E-15));
#39615=DIRECTION('center_axis',(1.,6.7618653731838E-14,-2.77102527463912E-15));
#39616=DIRECTION('ref_axis',(2.77102426704276E-15,1.49011597348792E-8,1.));
#39617=DIRECTION('center_axis',(-1.,-6.7618653731838E-14,2.77102527463912E-15));
#39618=DIRECTION('ref_axis',(2.7710242670427E-15,1.49011606550806E-8,1.));
#39619=DIRECTION('center_axis',(-1.,-5.87324028735622E-14,-6.11522571605215E-15));
#39620=DIRECTION('ref_axis',(-6.11522659123301E-15,1.49011588146778E-8,
1.));
#39621=DIRECTION('',(-1.,-6.7618653731838E-14,2.77102527463912E-15));
#39622=DIRECTION('center_axis',(2.77102527463854E-15,8.5557679050281E-15,
1.));
#39623=DIRECTION('ref_axis',(-6.7618653731838E-14,1.,-8.55576790502791E-15));
#39624=DIRECTION('',(-6.7618653731838E-14,1.,-8.55576790502791E-15));
#39625=DIRECTION('',(-6.7618653731838E-14,1.,-8.55576790502791E-15));
#39626=DIRECTION('',(-1.,-6.7618653731838E-14,2.77102527463912E-15));
#39627=DIRECTION('center_axis',(1.,6.7618653731838E-14,-2.77102527463912E-15));
#39628=DIRECTION('ref_axis',(-6.7618653731838E-14,1.,-8.55576790502791E-15));
#39629=DIRECTION('center_axis',(-1.,-6.7618653731838E-14,2.77102527463912E-15));
#39630=DIRECTION('ref_axis',(-6.7618653731838E-14,1.,-8.55576790502791E-15));
#39631=DIRECTION('center_axis',(-1.,-6.7618653731838E-14,2.77102527463912E-15));
#39632=DIRECTION('ref_axis',(-6.7618653731838E-14,1.,-1.95981850583656E-14));
#39633=DIRECTION('',(-1.,-6.7618653731838E-14,2.77102527463912E-15));
#39634=DIRECTION('center_axis',(-6.7618653731838E-14,1.,-8.55576790502791E-15));
#39635=DIRECTION('ref_axis',(-2.77102527463854E-15,-8.5557679050281E-15,
-1.));
#39636=DIRECTION('',(-2.77102527463854E-15,-8.5557679050281E-15,-1.));
#39637=DIRECTION('',(-2.77102527463854E-15,-8.5557679050281E-15,-1.));
#39638=DIRECTION('center_axis',(-1.,-6.7618653731838E-14,2.77102527463912E-15));
#39639=DIRECTION('ref_axis',(-6.7618653731838E-14,1.,-8.55576790502791E-15));
#39640=DIRECTION('',(2.77102527463854E-15,8.5557679050281E-15,1.));
#39641=DIRECTION('',(6.7618653731838E-14,-1.,8.55576790502791E-15));
#39642=DIRECTION('',(2.77102527463854E-15,8.5557679050281E-15,1.));
#39643=DIRECTION('',(6.7618653731838E-14,-1.,8.55576790502791E-15));
#39644=DIRECTION('center_axis',(1.,6.7618653731838E-14,-2.77102527463912E-15));
#39645=DIRECTION('ref_axis',(6.7618653731838E-14,-1.,8.55576790502791E-15));
#39646=DIRECTION('center_axis',(1.,6.7618653731838E-14,-2.77102527463912E-15));
#39647=DIRECTION('ref_axis',(-2.77102527463861E-15,-7.46981590754665E-15,
-1.));
#39648=DIRECTION('center_axis',(1.,6.7618653731838E-14,-2.77102527463912E-15));
#39649=DIRECTION('ref_axis',(-2.77102527463832E-15,-1.18136238974724E-14,
-1.));
#39650=DIRECTION('',(-2.77102527463854E-15,-8.5557679050281E-15,-1.));
#39651=DIRECTION('center_axis',(-1.,-6.7618653731838E-14,2.77102527463912E-15));
#39652=DIRECTION('ref_axis',(-2.77102527463854E-15,-8.5557679050281E-15,
-1.));
#39653=DIRECTION('',(6.7618653731838E-14,-1.,8.55576790502791E-15));
#39654=DIRECTION('center_axis',(-1.,-6.7618653731838E-14,2.77102527463912E-15));
#39655=DIRECTION('ref_axis',(6.7618653731838E-14,-1.,5.64179671178602E-15));
#39656=DIRECTION('',(2.77102527463854E-15,8.5557679050281E-15,1.));
#39657=DIRECTION('center_axis',(-1.,-5.35487561816597E-14,-1.12988722755394E-14));
#39658=DIRECTION('ref_axis',(-1.12988722755392E-14,-4.55710246456112E-15,
1.));
#39659=DIRECTION('',(-6.7618653731838E-14,1.,-8.55576790502791E-15));
#39660=DIRECTION('center_axis',(-1.,-8.16885512820165E-14,-1.12988722755392E-14));
#39661=DIRECTION('ref_axis',(-8.16885512820165E-14,1.,3.1001168679395E-15));
#39662=DIRECTION('center_axis',(1.,6.7618653731838E-14,-2.77102527463912E-15));
#39663=DIRECTION('ref_axis',(-2.77102527463627E-15,-4.20664366273117E-14,
-1.));
#39664=DIRECTION('',(-1.,-6.7618653731838E-14,2.77102527463912E-15));
#39665=DIRECTION('center_axis',(-1.,-5.354875618166E-14,-1.12988722755392E-14));
#39666=DIRECTION('ref_axis',(1.12988722755397E-14,-8.55576790502718E-15,
-1.));
#39667=DIRECTION('',(-1.,-6.7618653731838E-14,2.77102527463912E-15));
#39668=DIRECTION('center_axis',(-2.77102527463854E-15,-8.5557679050281E-15,
-1.));
#39669=DIRECTION('ref_axis',(6.7618653731838E-14,-1.,8.55576790502791E-15));
#39670=DIRECTION('',(6.7618653731838E-14,-1.,8.55576790502791E-15));
#39671=DIRECTION('',(-1.,-6.7618653731838E-14,2.77102527463912E-15));
#39672=DIRECTION('center_axis',(1.,6.7618653731838E-14,-2.77102527463912E-15));
#39673=DIRECTION('ref_axis',(6.76186537318381E-14,-1.,4.06094510306894E-14));
#39674=DIRECTION('center_axis',(-1.,-8.16885512820162E-14,-1.12988722755389E-14));
#39675=DIRECTION('ref_axis',(8.16885512820161E-14,-1.,5.64179671178601E-15));
#39676=DIRECTION('',(-1.,-6.7618653731838E-14,2.77102527463912E-15));
#39677=DIRECTION('center_axis',(6.7618653731838E-14,-1.,8.55576790502791E-15));
#39678=DIRECTION('ref_axis',(2.77102527463854E-15,8.5557679050281E-15,1.));
#39679=DIRECTION('',(2.77102527463854E-15,8.5557679050281E-15,1.));
#39680=DIRECTION('',(-1.,-6.7618653731838E-14,2.77102527463912E-15));
#39681=DIRECTION('center_axis',(1.,6.7618653731838E-14,-2.77102527463912E-15));
#39682=DIRECTION('ref_axis',(2.77102527463864E-15,7.09878230840716E-15,
1.));
#39683=DIRECTION('center_axis',(-1.,-6.7618653731838E-14,2.77102527463912E-15));
#39684=DIRECTION('ref_axis',(2.77102527463943E-15,-4.5571024645602E-15,
1.));
#39685=DIRECTION('',(-1.,-6.7618653731838E-14,2.77102527463912E-15));
#39686=DIRECTION('center_axis',(2.77102527463854E-15,8.5557679050281E-15,
1.));
#39687=DIRECTION('ref_axis',(-6.7618653731838E-14,1.,-8.55576790502791E-15));
#39688=DIRECTION('',(-6.7618653731838E-14,1.,-8.55576790502791E-15));
#39689=DIRECTION('',(-1.,-6.7618653731838E-14,2.77102527463912E-15));
#39690=DIRECTION('center_axis',(1.,6.7618653731838E-14,-2.77102527463912E-15));
#39691=DIRECTION('ref_axis',(-6.7618653731838E-14,1.,-8.55576790502791E-15));
#39692=DIRECTION('center_axis',(-1.,-6.7618653731838E-14,2.77102527463912E-15));
#39693=DIRECTION('ref_axis',(-6.7618653731838E-14,1.,3.10011686793949E-15));
#39694=DIRECTION('',(-1.,-6.7618653731838E-14,2.77102527463912E-15));
#39695=DIRECTION('center_axis',(-6.7618653731838E-14,1.,-8.55576790502791E-15));
#39696=DIRECTION('ref_axis',(-2.77102527463854E-15,-8.5557679050281E-15,
-1.));
#39697=DIRECTION('',(-2.77102527463854E-15,-8.5557679050281E-15,-1.));
#39698=DIRECTION('center_axis',(1.,6.7618653731838E-14,-2.77102527463912E-15));
#39699=DIRECTION('ref_axis',(6.7618653731838E-14,-1.,8.55576790502791E-15));
#39700=DIRECTION('center_axis',(-6.99688737499255E-14,1.,0.));
#39701=DIRECTION('ref_axis',(0.,-8.7461092187406E-15,-1.));
#39702=DIRECTION('center_axis',(-1.,-6.7618653731838E-14,2.77102527463912E-15));
#39703=DIRECTION('ref_axis',(-2.77102527463869E-15,-6.38386391006521E-15,
-1.));
#39704=DIRECTION('center_axis',(6.51793608929021E-13,0.707106781186447,
-0.707106781186648));
#39705=DIRECTION('ref_axis',(0.896534794971466,-0.313229437797635,-0.313229437796719));
#39706=DIRECTION('center_axis',(4.00117890718912E-13,-0.707106781186849,
-0.707106781186247));
#39707=DIRECTION('ref_axis',(0.996198003956249,-0.0616016919958765,0.0616016919964927));
#39708=DIRECTION('center_axis',(-3.6704722266697E-13,-0.707106781186503,
0.707106781186592));
#39709=DIRECTION('ref_axis',(0.996921797515119,-0.0554388385488158,-0.0554388385482913));
#39710=DIRECTION('center_axis',(-5.26061948198612E-13,-0.707106781186484,
-0.707106781186611));
#39711=DIRECTION('ref_axis',(0.896534794971479,-0.31322943779752,0.313229437796797));
#39712=DIRECTION('center_axis',(9.18554053444912E-12,-0.707106781186299,
0.707106781186796));
#39713=DIRECTION('ref_axis',(0.996198003956234,0.0616016920027945,0.0616016919898103));
#39714=DIRECTION('center_axis',(4.75776948071443E-13,0.707106781186498,
0.707106781186597));
#39715=DIRECTION('ref_axis',(0.996921797515123,-0.0554388385488504,0.0554388385481719));
#39716=DIRECTION('center_axis',(7.70726635632004E-13,-0.707106781186425,
0.70710678118667));
#39717=DIRECTION('ref_axis',(0.896534794971449,0.313229437797744,0.313229437796658));
#39718=DIRECTION('center_axis',(9.23046358674266E-12,0.707106781186311,
0.707106781186784));
#39719=DIRECTION('ref_axis',(0.996198003956241,0.061601691989768,-0.061601692002731));
#39720=DIRECTION('center_axis',(-6.34411876251122E-13,0.707106781186469,
-0.707106781186626));
#39721=DIRECTION('ref_axis',(0.996921797515115,0.0554388385490345,0.0554388385481277));
#39722=DIRECTION('center_axis',(-6.56544319852163E-13,0.707106781186476,
0.707106781186619));
#39723=DIRECTION('ref_axis',(0.896534794971433,0.313229437797672,-0.313229437796776));
#39724=DIRECTION('center_axis',(2.14647884590057E-14,0.707106781186789,
-0.707106781186307));
#39725=DIRECTION('ref_axis',(0.996198003956254,-0.0616016919961379,-0.0616016919961496));
#39726=DIRECTION('center_axis',(5.78996367848738E-13,-0.707106781186491,
-0.707106781186604));
#39727=DIRECTION('ref_axis',(0.996921797515118,0.0554388385489725,-0.0554388385481474));
#39728=DIRECTION('center_axis',(1.,6.7618653731838E-14,-2.77102527463912E-15));
#39729=DIRECTION('ref_axis',(-2.77102527463847E-15,-9.64171990250954E-15,
-1.));
#39730=DIRECTION('',(-1.,-6.7618653731838E-14,2.77102527463912E-15));
#39731=DIRECTION('center_axis',(-6.99688737499273E-14,1.,0.));
#39732=DIRECTION('ref_axis',(0.,-8.74610921874091E-15,-1.));
#39733=DIRECTION('center_axis',(-1.,-6.32748457419122E-14,2.77102527463908E-15));
#39734=DIRECTION('ref_axis',(-2.77102527463847E-15,-9.64171990250955E-15,
-1.));
#39735=DIRECTION('center_axis',(2.22250656035605E-13,0.707106781186488,
-0.707106781186608));
#39736=DIRECTION('ref_axis',(0.896534794971443,-0.313229437797377,-0.313229437797042));
#39737=DIRECTION('center_axis',(1.17092005636022E-13,-0.707106781186556,
-0.707106781186539));
#39738=DIRECTION('ref_axis',(0.996198003956251,-0.0616016919960817,0.0616016919962482));
#39739=DIRECTION('center_axis',(3.08468140487006E-13,-0.707106781186592,
0.707106781186503));
#39740=DIRECTION('ref_axis',(0.99692179751513,-0.0554388385482297,-0.0554388385486716));
#39741=DIRECTION('center_axis',(2.19731246458362E-13,-0.707106781186608,
-0.707106781186487));
#39742=DIRECTION('ref_axis',(0.896534794971441,-0.313229437797046,0.313229437797379));
#39743=DIRECTION('center_axis',(6.15824789516204E-13,-0.707106781186494,
0.707106781186602));
#39744=DIRECTION('ref_axis',(0.996198003956225,0.0616016919968157,0.0616016919959387));
#39745=DIRECTION('center_axis',(-1.98029326998358E-14,0.707106781186549,
0.707106781186547));
#39746=DIRECTION('ref_axis',(0.996921797515125,-0.0554388385484832,0.0554388385485112));
#39747=DIRECTION('center_axis',(6.31015736015947E-14,-0.70710678118654,
0.707106781186555));
#39748=DIRECTION('ref_axis',(0.896534794971412,0.313229437797297,0.313229437797211));
#39749=DIRECTION('center_axis',(1.51175084320796E-12,0.707106781186554,
0.707106781186542));
#39750=DIRECTION('ref_axis',(0.996198003956232,0.061601691995254,-0.0616016919973848));
#39751=DIRECTION('center_axis',(8.47242099047219E-14,0.70710678118659,-0.707106781186506));
#39752=DIRECTION('ref_axis',(0.996921797515118,0.0554388385484938,0.0554388385486198));
#39753=DIRECTION('center_axis',(8.8643031429794E-14,0.707106781186602,0.707106781186494));
#39754=DIRECTION('ref_axis',(0.896534794971411,0.313229437797176,-0.313229437797336));
#39755=DIRECTION('center_axis',(1.95394423019618E-14,0.707106781186544,
-0.707106781186551));
#39756=DIRECTION('ref_axis',(0.996198003956246,-0.0616016919962189,-0.0616016919961908));
#39757=DIRECTION('center_axis',(2.04087760748626E-14,-0.707106781186559,
-0.707106781186536));
#39758=DIRECTION('ref_axis',(0.996921797515118,0.0554388385485753,-0.0554388385485483));
#39759=DIRECTION('center_axis',(1.,6.7618653731838E-14,-2.77102527463912E-15));
#39760=DIRECTION('ref_axis',(-2.77102527463854E-15,-8.5557679050281E-15,
-1.));
#39761=DIRECTION('',(-1.,-6.7618653731838E-14,2.77102527463912E-15));
#39762=DIRECTION('center_axis',(4.9773019351027E-14,-0.707106781186589,
0.707106781186506));
#39763=DIRECTION('ref_axis',(-4.58541978259481E-14,0.707106781186506,0.707106781186589));
#39764=DIRECTION('',(1.,6.7618653731838E-14,-2.77102527463912E-15));
#39765=DIRECTION('',(4.58541978259513E-14,-0.707106781186551,-0.707106781186544));
#39766=DIRECTION('',(1.,6.7618653731838E-14,-2.77102527463912E-15));
#39767=DIRECTION('center_axis',(-4.58541978259514E-14,0.707106781186553,
0.707106781186542));
#39768=DIRECTION('ref_axis',(-4.9773019351024E-14,0.707106781186542,-0.707106781186553));
#39769=DIRECTION('',(4.97730193510239E-14,-0.707106781186541,0.707106781186554));
#39770=DIRECTION('',(1.,6.7618653731838E-14,-2.77102527463912E-15));
#39771=DIRECTION('center_axis',(4.97730193510239E-14,-0.707106781186541,
0.707106781186554));
#39772=DIRECTION('ref_axis',(-4.58541978259515E-14,0.707106781186554,0.707106781186541));
#39773=DIRECTION('',(4.58541978259515E-14,-0.707106781186554,-0.707106781186541));
#39774=DIRECTION('',(1.,6.7618653731838E-14,-2.77102527463912E-15));
#39775=DIRECTION('center_axis',(-4.58541978259512E-14,0.707106781186549,
0.707106781186546));
#39776=DIRECTION('ref_axis',(-4.97730193510242E-14,0.707106781186546,-0.707106781186549));
#39777=DIRECTION('',(4.97730193510238E-14,-0.707106781186539,0.707106781186556));
#39778=DIRECTION('',(1.,6.7618653731838E-14,-2.77102527463912E-15));
#39779=DIRECTION('center_axis',(-4.97730193510225E-14,0.707106781186519,
-0.707106781186576));
#39780=DIRECTION('ref_axis',(4.58541978259531E-14,-0.707106781186576,-0.707106781186519));
#39781=DIRECTION('',(-4.585419782595E-14,0.707106781186533,0.707106781186562));
#39782=DIRECTION('',(1.,6.7618653731838E-14,-2.77102527463912E-15));
#39783=DIRECTION('center_axis',(-4.58541978259529E-14,0.707106781186574,
0.707106781186521));
#39784=DIRECTION('ref_axis',(-4.97730193510226E-14,0.707106781186521,-0.707106781186574));
#39785=DIRECTION('',(4.97730193510239E-14,-0.707106781186541,0.707106781186554));
#39786=DIRECTION('',(1.,6.7618653731838E-14,-2.77102527463912E-15));
#39787=DIRECTION('center_axis',(-4.97730193510239E-14,0.707106781186542,
-0.707106781186554));
#39788=DIRECTION('ref_axis',(4.58541978259515E-14,-0.707106781186554,-0.707106781186541));
#39789=DIRECTION('',(-4.58541978259481E-14,0.707106781186505,0.70710678118659));
#39790=DIRECTION('',(1.,6.7618653731838E-14,-2.77102527463912E-15));
#39791=DIRECTION('center_axis',(4.58541978259531E-14,-0.707106781186576,
-0.707106781186519));
#39792=DIRECTION('ref_axis',(4.97730193510225E-14,-0.707106781186519,0.707106781186576));
#39793=DIRECTION('',(-4.9773019351024E-14,0.707106781186542,-0.707106781186553));
#39794=DIRECTION('',(1.,6.7618653731838E-14,-2.77102527463912E-15));
#39795=DIRECTION('center_axis',(-4.97730193510253E-14,0.707106781186563,
-0.707106781186532));
#39796=DIRECTION('ref_axis',(4.585419782595E-14,-0.707106781186532,-0.707106781186563));
#39797=DIRECTION('',(-4.58541978259528E-14,0.707106781186573,0.707106781186522));
#39798=DIRECTION('',(1.,6.7618653731838E-14,-2.77102527463912E-15));
#39799=DIRECTION('center_axis',(4.58541978259515E-14,-0.707106781186554,
-0.707106781186542));
#39800=DIRECTION('ref_axis',(4.97730193510239E-14,-0.707106781186541,0.707106781186554));
#39801=DIRECTION('',(-4.97730193510206E-14,0.707106781186491,-0.707106781186604));
#39802=DIRECTION('',(1.,6.7618653731838E-14,-2.77102527463912E-15));
#39803=DIRECTION('center_axis',(4.97730193510253E-14,-0.707106781186562,
0.707106781186533));
#39804=DIRECTION('ref_axis',(-4.585419782595E-14,0.707106781186533,0.707106781186562));
#39805=DIRECTION('',(4.58541978259514E-14,-0.707106781186553,-0.707106781186542));
#39806=DIRECTION('',(1.,6.7618653731838E-14,-2.77102527463912E-15));
#39807=DIRECTION('center_axis',(4.58541978259515E-14,-0.707106781186554,
-0.707106781186542));
#39808=DIRECTION('ref_axis',(4.97730193510239E-14,-0.707106781186541,0.707106781186554));
#39809=DIRECTION('',(-4.97730193510239E-14,0.707106781186541,-0.707106781186554));
#39810=DIRECTION('center_axis',(1.,6.7618653731838E-14,-2.77102527463912E-15));
#39811=DIRECTION('ref_axis',(6.7618653731838E-14,-1.,8.55576790502791E-15));
#39812=DIRECTION('center_axis',(4.97730193510297E-14,-0.707106781186631,
0.707106781186464));
#39813=DIRECTION('ref_axis',(-4.58541978259452E-14,0.707106781186464,0.707106781186631));
#39814=DIRECTION('',(1.,6.7618653731838E-14,-2.77102527463912E-15));
#39815=DIRECTION('',(4.58541978259341E-14,-0.707106781186307,-0.707106781186788));
#39816=DIRECTION('',(1.,6.7618653731838E-14,-2.77102527463912E-15));
#39817=DIRECTION('center_axis',(-4.58541978259499E-14,0.707106781186531,
0.707106781186564));
#39818=DIRECTION('ref_axis',(-4.97730193510254E-14,0.707106781186564,-0.707106781186531));
#39819=DIRECTION('',(4.97730193510227E-14,-0.707106781186522,0.707106781186573));
#39820=DIRECTION('',(1.,6.7618653731838E-14,-2.77102527463912E-15));
#39821=DIRECTION('center_axis',(4.97730193510225E-14,-0.707106781186519,
0.707106781186576));
#39822=DIRECTION('ref_axis',(-4.58541978259531E-14,0.707106781186576,0.707106781186519));
#39823=DIRECTION('',(4.585419782595E-14,-0.707106781186532,-0.707106781186563));
#39824=DIRECTION('',(1.,6.7618653731838E-14,-2.77102527463912E-15));
#39825=DIRECTION('center_axis',(-4.58541978259578E-14,0.707106781186643,
0.707106781186452));
#39826=DIRECTION('ref_axis',(-4.97730193510181E-14,0.707106781186452,-0.707106781186643));
#39827=DIRECTION('',(4.97730193510079E-14,-0.707106781186295,0.7071067811868));
#39828=DIRECTION('',(1.,6.7618653731838E-14,-2.77102527463912E-15));
#39829=DIRECTION('center_axis',(-4.97730193510214E-14,0.707106781186502,
-0.707106781186593));
#39830=DIRECTION('ref_axis',(4.58541978259543E-14,-0.707106781186593,-0.707106781186502));
#39831=DIRECTION('',(-4.585419782595E-14,0.707106781186532,0.707106781186563));
#39832=DIRECTION('',(1.,6.7618653731838E-14,-2.77102527463912E-15));
#39833=DIRECTION('center_axis',(-4.58541978259487E-14,0.707106781186514,
0.707106781186581));
#39834=DIRECTION('ref_axis',(-4.97730193510265E-14,0.707106781186581,-0.707106781186514));
#39835=DIRECTION('',(4.97730193510225E-14,-0.70710678118652,0.707106781186575));
#39836=DIRECTION('',(1.,6.7618653731838E-14,-2.77102527463912E-15));
#39837=DIRECTION('center_axis',(-4.97730193510303E-14,0.707106781186639,
-0.707106781186456));
#39838=DIRECTION('ref_axis',(4.58541978259446E-14,-0.707106781186456,-0.707106781186639));
#39839=DIRECTION('',(-4.58541978259685E-14,0.707106781186796,0.707106781186299));
#39840=DIRECTION('',(1.,6.7618653731838E-14,-2.77102527463912E-15));
#39841=DIRECTION('center_axis',(4.58541978259488E-14,-0.707106781186515,
-0.70710678118658));
#39842=DIRECTION('ref_axis',(4.97730193510264E-14,-0.70710678118658,0.707106781186515));
#39843=DIRECTION('',(-4.97730193510223E-14,0.707106781186516,-0.707106781186579));
#39844=DIRECTION('',(1.,6.7618653731838E-14,-2.77102527463912E-15));
#39845=DIRECTION('center_axis',(-4.97730193510214E-14,0.707106781186502,
-0.707106781186593));
#39846=DIRECTION('ref_axis',(4.58541978259543E-14,-0.707106781186593,-0.707106781186502));
#39847=DIRECTION('',(-4.58541978259498E-14,0.70710678118653,0.707106781186565));
#39848=DIRECTION('',(1.,6.7618653731838E-14,-2.77102527463912E-15));
#39849=DIRECTION('center_axis',(4.58541978259616E-14,-0.707106781186697,
-0.707106781186398));
#39850=DIRECTION('ref_axis',(4.97730193510146E-14,-0.707106781186398,0.707106781186697));
#39851=DIRECTION('',(-4.97730193510397E-14,0.707106781186784,-0.707106781186311));
#39852=DIRECTION('',(1.,6.7618653731838E-14,-2.77102527463912E-15));
#39853=DIRECTION('center_axis',(4.97730193510213E-14,-0.707106781186501,
0.707106781186594));
#39854=DIRECTION('ref_axis',(-4.58541978259543E-14,0.707106781186594,0.707106781186501));
#39855=DIRECTION('',(4.585419782595E-14,-0.707106781186533,-0.707106781186562));
#39856=DIRECTION('',(1.,6.7618653731838E-14,-2.77102527463912E-15));
#39857=DIRECTION('center_axis',(3.16979723399869E-14,-0.707106781186513,
-0.707106781186582));
#39858=DIRECTION('ref_axis',(4.97730193510266E-14,-0.707106781186582,0.707106781186513));
#39859=DIRECTION('',(-4.97730193510212E-14,0.7071067811865,-0.707106781186595));
#39860=DIRECTION('center_axis',(1.,6.7618653731838E-14,-2.77102527463912E-15));
#39861=DIRECTION('ref_axis',(6.7618653731838E-14,-1.,8.55576790502791E-15));
#39862=DIRECTION('center_axis',(0.857167300702084,0.515038074910101,-6.78177848602247E-15));
#39863=DIRECTION('ref_axis',(-2.77102527463854E-15,-8.5557679050281E-15,
-1.));
#39864=DIRECTION('',(-2.77102527463854E-15,-8.5557679050281E-15,-1.));
#39865=DIRECTION('',(-0.515038074910099,0.857167300702085,-5.90654095760941E-15));
#39866=DIRECTION('',(2.77102527463854E-15,8.5557679050281E-15,1.));
#39867=DIRECTION('',(-0.515038074910089,0.857167300702092,-5.90654095760949E-15));
#39868=DIRECTION('',(2.77102527463854E-15,8.5557679050281E-15,1.));
#39869=DIRECTION('',(0.515038074910119,-0.857167300702073,5.90654095760925E-15));
#39870=DIRECTION('',(2.77102527463854E-15,8.5557679050281E-15,1.));
#39871=DIRECTION('',(0.515038074910127,-0.857167300702068,5.90654095760919E-15));
#39872=DIRECTION('',(-2.77102527463854E-15,-8.5557679050281E-15,-1.));
#39873=DIRECTION('center_axis',(-0.515038074910076,0.857167300702099,-5.90654095760959E-15));
#39874=DIRECTION('ref_axis',(-2.77102527463854E-15,-8.5557679050281E-15,
-1.));
#39875=DIRECTION('',(0.857167300702085,0.515038074910099,-6.78177848602246E-15));
#39876=DIRECTION('center_axis',(-2.77102527463854E-15,-8.5557679050281E-15,
-1.));
#39877=DIRECTION('ref_axis',(6.7618653731838E-14,-1.,8.55576790502791E-15));
#39878=DIRECTION('',(0.8571673007021,0.515038074910075,-6.78177848602229E-15));
#39879=DIRECTION('center_axis',(0.515038074910084,-0.857167300702094,5.90654095760953E-15));
#39880=DIRECTION('ref_axis',(2.77102527463854E-15,8.5557679050281E-15,1.));
#39881=DIRECTION('',(0.857167300702077,0.515038074910113,-6.78177848602255E-15));
#39882=DIRECTION('center_axis',(-2.77102527463854E-15,-8.5557679050281E-15,
-1.));
#39883=DIRECTION('ref_axis',(6.7618653731838E-14,-1.,8.55576790502791E-15));
#39884=DIRECTION('',(0.85716730070208,0.515038074910108,-6.78177848602252E-15));
#39885=DIRECTION('center_axis',(0.51503807491009,-0.857167300702091,5.90654095760948E-15));
#39886=DIRECTION('ref_axis',(2.77102527463854E-15,8.5557679050281E-15,1.));
#39887=DIRECTION('',(0.857167300702075,0.515038074910117,-6.78177848602258E-15));
#39888=DIRECTION('center_axis',(2.77102527463854E-15,8.5557679050281E-15,
1.));
#39889=DIRECTION('ref_axis',(-6.7618653731838E-14,1.,-8.55576790502791E-15));
#39890=DIRECTION('',(0.857167300702077,0.515038074910113,-6.78177848602255E-15));
#39891=DIRECTION('center_axis',(0.515038074910101,-0.857167300702084,5.90654095760939E-15));
#39892=DIRECTION('ref_axis',(2.77102527463854E-15,8.5557679050281E-15,1.));
#39893=DIRECTION('',(0.857167300702087,0.515038074910097,-6.78177848602244E-15));
#39894=DIRECTION('center_axis',(2.77102527463854E-15,8.5557679050281E-15,
1.));
#39895=DIRECTION('ref_axis',(-6.7618653731838E-14,1.,-8.55576790502791E-15));
#39896=DIRECTION('',(0.857167300702085,0.515038074910099,-6.78177848602246E-15));
#39897=DIRECTION('center_axis',(-0.515038074910086,0.857167300702093,-5.90654095760951E-15));
#39898=DIRECTION('ref_axis',(-2.77102527463854E-15,-8.5557679050281E-15,
-1.));
#39899=DIRECTION('center_axis',(-1.,-6.7618653731838E-14,2.77102527463912E-15));
#39900=DIRECTION('ref_axis',(2.7710252746386E-15,7.63556647558329E-15,1.));
#39901=DIRECTION('',(-1.,-6.7618653731838E-14,2.77102527463912E-15));
#39902=DIRECTION('',(1.,6.7618653731838E-14,-2.77102527463912E-15));
#39903=DIRECTION('center_axis',(-6.7618653731838E-14,1.,-8.55576790502791E-15));
#39904=DIRECTION('ref_axis',(-2.77102527463854E-15,-8.5557679050281E-15,
-1.));
#39905=DIRECTION('',(1.,6.7618653731838E-14,-2.77102527463912E-15));
#39906=DIRECTION('',(-2.77102527463854E-15,-8.5557679050281E-15,-1.));
#39907=DIRECTION('center_axis',(-2.77102527463854E-15,-8.5557679050281E-15,
-1.));
#39908=DIRECTION('ref_axis',(6.7618653731838E-14,-1.,8.55576790502791E-15));
#39909=DIRECTION('center_axis',(-3.95128286645425E-13,-2.33583808290282E-13,
-1.));
#39910=DIRECTION('ref_axis',(0.880460531975146,0.474119448698367,-4.58641487869712E-13));
#39911=DIRECTION('center_axis',(2.77102527463854E-15,8.5557679050281E-15,
1.));
#39912=DIRECTION('ref_axis',(-6.7618653731838E-14,1.,-8.55576790502791E-15));
#39913=DIRECTION('center_axis',(-4.70892792007641E-13,-2.56506629572123E-13,
1.));
#39914=DIRECTION('ref_axis',(0.856355995328812,0.516385911179227,5.3570827522798E-13));
#39915=DIRECTION('center_axis',(-1.,-6.7618653731838E-14,2.77102527463912E-15));
#39916=DIRECTION('ref_axis',(-2.77102527463854E-15,-8.5557679050281E-15,
-1.));
#39917=DIRECTION('',(1.,6.7618653731838E-14,-2.77102527463912E-15));
#39918=DIRECTION('',(-1.,-6.7618653731838E-14,2.77102527463912E-15));
#39919=DIRECTION('center_axis',(-2.77102527463854E-15,-8.5557679050281E-15,
-1.));
#39920=DIRECTION('ref_axis',(6.7618653731838E-14,-1.,8.55576790502791E-15));
#39921=DIRECTION('',(1.,6.7618653731838E-14,-2.77102527463912E-15));
#39922=DIRECTION('',(-1.,-6.7618653731838E-14,2.77102527463912E-15));
#39923=DIRECTION('center_axis',(2.59167743232149E-16,-1.01673529621644E-14,
-1.));
#39924=DIRECTION('ref_axis',(0.88885275239948,-0.458192955589529,4.88897146616111E-15));
#39925=DIRECTION('center_axis',(2.77102527463854E-15,8.5557679050281E-15,
1.));
#39926=DIRECTION('ref_axis',(-6.7618653731838E-14,1.,-8.55576790502791E-15));
#39927=DIRECTION('center_axis',(-1.02909387888083E-15,8.10142695923282E-15,
1.));
#39928=DIRECTION('ref_axis',(0.88885275239942,0.458192955589646,-2.7973038362239E-15));
#39929=DIRECTION('',(-1.,-6.7618653731838E-14,2.77102527463912E-15));
#39930=DIRECTION('',(1.,6.7618653731838E-14,-2.77102527463912E-15));
#39931=DIRECTION('center_axis',(-2.77102527463854E-15,-8.5557679050281E-15,
-1.));
#39932=DIRECTION('ref_axis',(6.7618653731838E-14,-1.,8.55576790502791E-15));
#39933=DIRECTION('center_axis',(5.00248153014182E-16,-2.81970907598089E-15,
-1.));
#39934=DIRECTION('ref_axis',(0.856355995328885,-0.516385911179105,1.88444854544628E-15));
#39935=DIRECTION('center_axis',(2.77102527463854E-15,8.5557679050281E-15,
1.));
#39936=DIRECTION('ref_axis',(-6.7618653731838E-14,1.,-8.55576790502791E-15));
#39937=DIRECTION('center_axis',(5.53379700565215E-13,-3.04189065102847E-13,
1.));
#39938=DIRECTION('ref_axis',(0.880460531975183,-0.474119448698298,-6.31450937390529E-13));
#39939=DIRECTION('',(1.,6.7618653731838E-14,-2.77102527463912E-15));
#39940=DIRECTION('center_axis',(6.7618653731838E-14,-1.,8.55576790502791E-15));
#39941=DIRECTION('ref_axis',(2.77102527463854E-15,8.5557679050281E-15,1.));
#39942=DIRECTION('',(2.77102527463854E-15,8.5557679050281E-15,1.));
#39943=DIRECTION('center_axis',(6.7618653731838E-14,-1.,8.55576790502791E-15));
#39944=DIRECTION('ref_axis',(2.77102527463854E-15,8.5557679050281E-15,1.));
#39945=DIRECTION('center_axis',(-6.74540619515736E-14,1.,-8.39117612476355E-15));
#39946=DIRECTION('ref_axis',(1.47128018848125E-14,-8.39117612476256E-15,
-1.));
#39947=DIRECTION('center_axis',(-6.7618653731838E-14,1.,-8.55576790502791E-15));
#39948=DIRECTION('ref_axis',(-2.77102527463854E-15,-8.5557679050281E-15,
-1.));
#39949=DIRECTION('center_axis',(0.515038074909993,0.857167300702149,-1.91875610040794E-14));
#39950=DIRECTION('ref_axis',(-2.80848657939479E-15,-2.06973404938391E-14,
-1.));
#39951=DIRECTION('',(0.857167300702153,-0.515038074909987,2.03131397634296E-15));
#39952=DIRECTION('',(-2.77102527463854E-15,-8.5557679050281E-15,-1.));
#39953=DIRECTION('',(0.857167300702159,-0.515038074909977,2.03131397634286E-15));
#39954=DIRECTION('center_axis',(2.77102527463854E-15,8.5557679050281E-15,
1.));
#39955=DIRECTION('ref_axis',(-6.7618653731838E-14,1.,-8.55576790502791E-15));
#39956=DIRECTION('',(0.515038074909973,0.857167300702161,-8.76090800356383E-15));
#39957=DIRECTION('',(0.857167300702151,-0.51503807490999,2.031313976343E-15));
#39958=DIRECTION('center_axis',(2.77102527463854E-15,8.5557679050281E-15,
1.));
#39959=DIRECTION('ref_axis',(-6.7618653731838E-14,1.,-8.55576790502791E-15));
#39960=DIRECTION('',(0.857167300702156,-0.515038074909982,2.03131397634291E-15));
#39961=DIRECTION('',(0.515038074909941,0.857167300702181,-8.76090800356391E-15));
#39962=DIRECTION('center_axis',(0.515038074909987,0.857167300702153,-8.7609080035638E-15));
#39963=DIRECTION('ref_axis',(-2.77102527463854E-15,-8.5557679050281E-15,
-1.));
#39964=DIRECTION('',(-2.77102527463854E-15,-8.5557679050281E-15,-1.));
#39965=DIRECTION('',(0.857167300702151,-0.51503807490999,2.031313976343E-15));
#39966=DIRECTION('center_axis',(-2.77102527463854E-15,-8.5557679050281E-15,
-1.));
#39967=DIRECTION('ref_axis',(6.7618653731838E-14,-1.,8.55576790502791E-15));
#39968=DIRECTION('',(-0.515038074909973,-0.857167300702161,8.76090800356383E-15));
#39969=DIRECTION('',(0.857167300702159,-0.515038074909977,2.03131397634286E-15));
#39970=DIRECTION('center_axis',(0.515038074909993,0.857167300702149,-8.76090800356378E-15));
#39971=DIRECTION('ref_axis',(-2.77102527463854E-15,-8.5557679050281E-15,
-1.));
#39972=DIRECTION('',(-2.77102527463854E-15,-8.5557679050281E-15,-1.));
#39973=DIRECTION('',(0.857167300702153,-0.515038074909987,2.03131397634296E-15));
#39974=DIRECTION('center_axis',(-2.77102527463854E-15,-8.5557679050281E-15,
-1.));
#39975=DIRECTION('ref_axis',(6.7618653731838E-14,-1.,8.55576790502791E-15));
#39976=DIRECTION('',(-0.515038074909941,-0.857167300702181,8.76090800356391E-15));
#39977=DIRECTION('',(0.857167300702156,-0.515038074909982,2.03131397634291E-15));
#39978=DIRECTION('center_axis',(-0.515038074910012,-0.857167300702138,8.76090800356374E-15));
#39979=DIRECTION('ref_axis',(2.77102527463854E-15,8.5557679050281E-15,1.));
#39980=DIRECTION('',(2.77102527463854E-15,8.5557679050281E-15,1.));
#39981=DIRECTION('',(0.857167300702159,-0.515038074909977,2.03131397634286E-15));
#39982=DIRECTION('center_axis',(-2.77102527463854E-15,-8.5557679050281E-15,
-1.));
#39983=DIRECTION('ref_axis',(6.7618653731838E-14,-1.,8.55576790502791E-15));
#39984=DIRECTION('',(-0.515038074909971,-0.857167300702162,8.76090800356383E-15));
#39985=DIRECTION('',(0.857167300702144,-0.515038074910001,2.03131397634311E-15));
#39986=DIRECTION('center_axis',(-0.51503807491001,-0.857167300702139,8.76090800356374E-15));
#39987=DIRECTION('ref_axis',(2.77102527463854E-15,8.5557679050281E-15,1.));
#39988=DIRECTION('',(2.77102527463854E-15,8.5557679050281E-15,1.));
#39989=DIRECTION('',(0.857167300702144,-0.515038074910001,2.03131397634311E-15));
#39990=DIRECTION('center_axis',(2.77102527463854E-15,8.5557679050281E-15,
1.));
#39991=DIRECTION('ref_axis',(-6.7618653731838E-14,1.,-8.55576790502791E-15));
#39992=DIRECTION('',(0.515038074909971,0.857167300702162,-8.76090800356383E-15));
#39993=DIRECTION('',(0.857167300702159,-0.515038074909977,2.03131397634286E-15));
#39994=DIRECTION('center_axis',(-6.7618653731838E-14,1.,-8.55576790502791E-15));
#39995=DIRECTION('ref_axis',(-2.77102527463854E-15,-8.5557679050281E-15,
-1.));
#39996=DIRECTION('',(-6.7618653731838E-14,1.,-8.55576790502791E-15));
#39997=DIRECTION('center_axis',(-6.6659342535235E-14,1.,-7.59645670842486E-15));
#39998=DIRECTION('ref_axis',(-1.,-6.6659342535235E-14,-2.79201063973172E-15));
#39999=DIRECTION('center_axis',(6.7618653731838E-14,-1.,8.55576790502791E-15));
#40000=DIRECTION('ref_axis',(2.77102527463854E-15,8.5557679050281E-15,1.));
#40001=DIRECTION('center_axis',(0.857167300702162,-0.515038074909972,2.03131397634281E-15));
#40002=DIRECTION('ref_axis',(2.77102527463854E-15,8.5557679050281E-15,1.));
#40003=DIRECTION('',(2.77102527463854E-15,8.5557679050281E-15,1.));
#40004=DIRECTION('center_axis',(-0.515038074910012,-0.857167300702138,8.76090800356374E-15));
#40005=DIRECTION('ref_axis',(2.77102527463854E-15,8.5557679050281E-15,1.));
#40006=DIRECTION('center_axis',(-7.09168149328414E-14,1.,0.));
#40007=DIRECTION('ref_axis',(0.,-8.86460186660509E-15,-1.));
#40008=DIRECTION('center_axis',(0.515038074910022,-0.857167300702132,-5.09723557356589E-14));
#40009=DIRECTION('ref_axis',(0.765900867954176,0.460199669632626,0.449012387955011));
#40010=DIRECTION('center_axis',(-3.34893569076932E-13,-1.94333589280781E-13,
1.));
#40011=DIRECTION('ref_axis',(0.808168976755105,0.588950681305834,3.85103492850293E-13));
#40012=DIRECTION('center_axis',(-0.515038074910272,0.857167300701981,-9.75530354987259E-14));
#40013=DIRECTION('ref_axis',(0.854456218440534,0.513409092344432,0.079471219107103));
#40014=DIRECTION('center_axis',(5.41438285992961E-14,6.29175671824922E-14,
1.));
#40015=DIRECTION('ref_axis',(0.534642392050907,0.84507840619796,-8.21178634335555E-14));
#40016=DIRECTION('center_axis',(-0.515038074910461,0.857167300701868,-5.90654095760654E-15));
#40017=DIRECTION('ref_axis',(0.853796957819265,0.513012968599682,-0.0885914717515699));
#40018=DIRECTION('center_axis',(4.86017780500163E-14,4.58060313724332E-14,
-1.));
#40019=DIRECTION('ref_axis',(0.813525514740932,0.581529222709832,6.61763323248973E-14));
#40020=DIRECTION('center_axis',(-0.515038074909955,0.857167300702172,-1.78183517834286E-14));
#40021=DIRECTION('ref_axis',(0.765900867954212,0.460199669632583,-0.449012387954995));
#40022=DIRECTION('center_axis',(-3.40435619625912E-13,-2.11445125090658E-13,
-1.));
#40023=DIRECTION('ref_axis',(0.899424938883873,0.437075255892783,-3.9861371853221E-13));
#40024=DIRECTION('center_axis',(0.515038074910064,-0.857167300702106,4.90124063835157E-14));
#40025=DIRECTION('ref_axis',(0.854456218440668,0.513409092344217,-0.0794712191070439));
#40026=DIRECTION('center_axis',(-2.77102527463854E-15,-8.5557679050281E-15,
-1.));
#40027=DIRECTION('ref_axis',(0.997159343857257,0.0753209330675436,-3.4075821663865E-15));
#40028=DIRECTION('center_axis',(0.857167300702092,0.515038074910088,-6.78177848602238E-15));
#40029=DIRECTION('ref_axis',(-2.77102527463854E-15,-8.5557679050281E-15,
-1.));
#40030=DIRECTION('',(-0.515038074910087,0.857167300702093,-5.90654095760951E-15));
#40031=DIRECTION('',(-2.77102527463854E-15,-8.5557679050281E-15,-1.));
#40032=DIRECTION('',(-0.515038074910099,0.857167300702085,-5.90654095760941E-15));
#40033=DIRECTION('',(2.77102527463854E-15,8.5557679050281E-15,1.));
#40034=DIRECTION('',(-0.515038074910089,0.857167300702092,-5.90654095760949E-15));
#40035=DIRECTION('',(2.77102527463854E-15,8.5557679050281E-15,1.));
#40036=DIRECTION('',(0.515038074910089,-0.857167300702092,5.90654095760949E-15));
#40037=DIRECTION('',(2.77102527463854E-15,8.5557679050281E-15,1.));
#40038=DIRECTION('',(0.515038074910057,-0.857167300702111,5.90654095760974E-15));
#40039=DIRECTION('',(-2.77102527463854E-15,-8.5557679050281E-15,-1.));
#40040=DIRECTION('center_axis',(-0.515038074910083,0.857167300702095,-5.90654095760954E-15));
#40041=DIRECTION('ref_axis',(-2.77102527463854E-15,-8.5557679050281E-15,
-1.));
#40042=DIRECTION('',(0.857167300702109,0.515038074910059,-6.78177848602218E-15));
#40043=DIRECTION('center_axis',(-2.77102527463854E-15,-8.5557679050281E-15,
-1.));
#40044=DIRECTION('ref_axis',(6.7618653731838E-14,-1.,8.55576790502791E-15));
#40045=DIRECTION('',(0.857167300702093,0.515038074910086,-6.78177848602236E-15));
#40046=DIRECTION('center_axis',(0.515038074910109,-0.85716730070208,5.90654095760933E-15));
#40047=DIRECTION('ref_axis',(2.77102527463854E-15,8.5557679050281E-15,1.));
#40048=DIRECTION('',(0.857167300702082,0.515038074910104,-6.78177848602249E-15));
#40049=DIRECTION('center_axis',(-2.77102527463854E-15,-8.5557679050281E-15,
-1.));
#40050=DIRECTION('ref_axis',(6.7618653731838E-14,-1.,8.55576790502791E-15));
#40051=DIRECTION('',(0.857167300702081,0.515038074910106,-6.7817784860225E-15));
#40052=DIRECTION('center_axis',(0.515038074910096,-0.857167300702087,5.90654095760943E-15));
#40053=DIRECTION('ref_axis',(2.77102527463854E-15,8.5557679050281E-15,1.));
#40054=DIRECTION('',(0.857167300702081,0.515038074910106,-6.7817784860225E-15));
#40055=DIRECTION('center_axis',(2.77102527463854E-15,8.5557679050281E-15,
1.));
#40056=DIRECTION('ref_axis',(-6.7618653731838E-14,1.,-8.55576790502791E-15));
#40057=DIRECTION('',(0.857167300702082,0.515038074910104,-6.78177848602249E-15));
#40058=DIRECTION('center_axis',(0.51503807491008,-0.857167300702097,5.90654095760956E-15));
#40059=DIRECTION('ref_axis',(2.77102527463854E-15,8.5557679050281E-15,1.));
#40060=DIRECTION('',(0.857167300702093,0.515038074910086,-6.78177848602236E-15));
#40061=DIRECTION('center_axis',(2.77102527463854E-15,8.5557679050281E-15,
1.));
#40062=DIRECTION('ref_axis',(-6.7618653731838E-14,1.,-8.55576790502791E-15));
#40063=DIRECTION('',(0.857167300702109,0.515038074910059,-6.78177848602218E-15));
#40064=DIRECTION('center_axis',(-0.515038074910084,0.857167300702095,-5.90654095760953E-15));
#40065=DIRECTION('ref_axis',(-2.77102527463854E-15,-8.5557679050281E-15,
-1.));
#40066=DIRECTION('',(0.857167300702087,0.515038074910096,-6.78177848602243E-15));
#40067=DIRECTION('center_axis',(2.77102527463854E-15,8.5557679050281E-15,
1.));
#40068=DIRECTION('ref_axis',(-6.7618653731838E-14,1.,-8.55576790502791E-15));
#40069=DIRECTION('center_axis',(-2.77102527463854E-15,-8.5557679050281E-15,
-1.));
#40070=DIRECTION('ref_axis',(6.7618653731838E-14,-1.,8.55576790502791E-15));
#40071=DIRECTION('center_axis',(-2.77102527463854E-15,-8.5557679050281E-15,
-1.));
#40072=DIRECTION('ref_axis',(-1.,-6.6598517921482E-14,2.77102527463911E-15));
#40073=DIRECTION('center_axis',(-2.77102527463854E-15,-8.5557679050281E-15,
-1.));
#40074=DIRECTION('ref_axis',(1.,6.78710947856367E-14,-2.77102527463912E-15));
#40075=DIRECTION('center_axis',(0.809016994374993,-0.58778525229241,1.31600269666953E-14));
#40076=DIRECTION('ref_axis',(-0.58778525229241,-0.809016994374993,8.55052942525792E-15));
#40077=DIRECTION('',(-0.809016994374993,0.587785252292411,-1.31600269666953E-14));
#40078=DIRECTION('center_axis',(-0.809016994375011,0.587785252292386,-4.7527885634039E-14));
#40079=DIRECTION('ref_axis',(-0.587785252292386,-0.809016994375011,-1.03345964395218E-13));
#40080=DIRECTION('center_axis',(-0.809016994375011,0.587785252292386,-4.7527885634039E-14));
#40081=DIRECTION('ref_axis',(-0.587785252292386,-0.809016994375011,-1.03345964395218E-13));
#40082=DIRECTION('center_axis',(6.7618653731838E-14,-1.,8.55576790502791E-15));
#40083=DIRECTION('ref_axis',(2.77102527463854E-15,8.5557679050281E-15,1.));
#40084=DIRECTION('center_axis',(-6.7618653731838E-14,1.,-8.55576790502791E-15));
#40085=DIRECTION('ref_axis',(-0.999999999999964,-6.76186560146574E-14,-2.66816709635331E-7));
#40086=DIRECTION('center_axis',(-6.7618653731838E-14,1.,-8.55576790502791E-15));
#40087=DIRECTION('ref_axis',(-0.999999999999964,-6.76186560146574E-14,-2.66816709635331E-7));
#40088=DIRECTION('center_axis',(-6.7618653731838E-14,1.,-8.55576790502791E-15));
#40089=DIRECTION('ref_axis',(1.,6.7618653731838E-14,-2.77102527463912E-15));
#40090=DIRECTION('',(6.7618653731838E-14,-1.,8.55576790502791E-15));
#40091=DIRECTION('center_axis',(6.76186537327884E-14,-1.,4.25205660328949E-15));
#40092=DIRECTION('ref_axis',(1.,6.76186537327884E-14,-2.77102527463912E-15));
#40093=DIRECTION('center_axis',(6.76186537327884E-14,-1.,4.25205660328949E-15));
#40094=DIRECTION('ref_axis',(1.,6.76186537327884E-14,-2.77102527463912E-15));
#40095=DIRECTION('center_axis',(0.8660254037839,0.500000000000933,-6.67766223488626E-15));
#40096=DIRECTION('ref_axis',(-2.77102527463854E-15,-8.5557679050281E-15,
-1.));
#40097=DIRECTION('center_axis',(-0.866025403783983,-0.500000000000789,1.25096941532722E-12));
#40098=DIRECTION('ref_axis',(5.94980265416061E-7,-1.03053354726044E-6,0.999999999999292));
#40099=DIRECTION('center_axis',(-0.866025403783983,-0.500000000000789,1.25096941532722E-12));
#40100=DIRECTION('ref_axis',(5.94980265416061E-7,-1.03053354726044E-6,0.999999999999292));
#40101=DIRECTION('center_axis',(-0.866025403784387,-0.500000000000089,4.3675291105943E-14));
#40102=DIRECTION('ref_axis',(-0.500000000000089,0.866025403784387,-6.02399971731799E-15));
#40103=DIRECTION('',(0.866025403784387,0.500000000000089,-4.3675291105943E-14));
#40104=DIRECTION('center_axis',(0.8660254037844,0.500000000000067,-1.42864757407154E-14));
#40105=DIRECTION('ref_axis',(-0.500000000000067,0.8660254037844,6.88713418504579E-15));
#40106=DIRECTION('center_axis',(1.36653725312799E-8,7.88970643311003E-9,
-1.));
#40107=DIRECTION('ref_axis',(0.49999999636864,-0.866025405881005,0.));
#40108=DIRECTION('center_axis',(-0.809016994376835,0.587785252289875,-2.78714765756024E-15));
#40109=DIRECTION('ref_axis',(-2.77102527463854E-15,-8.5557679050281E-15,
-1.));
#40110=DIRECTION('center_axis',(0.809016982702078,-0.587785268358799,-1.07442107896218E-9));
#40111=DIRECTION('ref_axis',(-2.68991140209819E-13,-1.82828450322239E-9,
1.));
#40112=DIRECTION('center_axis',(0.809016982702078,-0.587785268358799,-1.07442107896218E-9));
#40113=DIRECTION('ref_axis',(-2.68991140209819E-13,-1.82828450322239E-9,
1.));
#40114=DIRECTION('center_axis',(-0.587785268327129,-0.809016982725088,-1.31521403548603E-9));
#40115=DIRECTION('ref_axis',(-4.97129381068598E-15,1.6256975880891E-9,-1.));
#40116=DIRECTION('center_axis',(-1.,-2.90861433570666E-10,4.9713238625083E-15));
#40117=DIRECTION('ref_axis',(4.97129381117057E-15,1.03318399277558E-10,
1.));
#40118=DIRECTION('center_axis',(-2.94928246063151E-15,-8.30841608127262E-15,
-1.));
#40119=DIRECTION('ref_axis',(6.8138088415828E-14,-1.,7.50144092651318E-15));
#40120=DIRECTION('center_axis',(-2.77102527463857E-15,-8.1650678567722E-15,
-1.));
#40121=DIRECTION('ref_axis',(-1.,-6.65985179156601E-14,2.77102527463911E-15));
#40122=DIRECTION('center_axis',(-2.77102527463857E-15,-8.1650678567722E-15,
-1.));
#40123=DIRECTION('ref_axis',(-1.,-6.65985179156601E-14,2.77102527463911E-15));
#40124=DIRECTION('center_axis',(1.,6.75911083482698E-14,-2.94928246063208E-15));
#40125=DIRECTION('ref_axis',(-6.75911083482698E-14,1.,-7.81400096511789E-15));
#40126=DIRECTION('center_axis',(-2.77102527463854E-15,-8.5557679050281E-15,
-1.));
#40127=DIRECTION('ref_axis',(1.,6.89554556095436E-14,-2.77102527463913E-15));
#40128=DIRECTION('center_axis',(2.77102527463854E-15,8.56804070208913E-15,
1.));
#40129=DIRECTION('ref_axis',(-1.,-6.75495870696371E-14,2.77102527463912E-15));
#40130=DIRECTION('',(-2.77102527463854E-15,-8.56804070208913E-15,-1.));
#40131=DIRECTION('center_axis',(2.77102527463854E-15,8.5557679050281E-15,
1.));
#40132=DIRECTION('ref_axis',(-6.7618653731838E-14,1.,-8.55576790502791E-15));
#40133=DIRECTION('center_axis',(-2.77102527463854E-15,-8.5557679050281E-15,
-1.));
#40134=DIRECTION('ref_axis',(6.7618653731838E-14,-1.,8.55576790502791E-15));
#40135=DIRECTION('center_axis',(-2.77102527463854E-15,-8.5557679050281E-15,
-1.));
#40136=DIRECTION('ref_axis',(-1.,-6.55943646399812E-14,2.7710252746391E-15));
#40137=DIRECTION('center_axis',(2.77102527463854E-15,8.5680407190582E-15,
1.));
#40138=DIRECTION('ref_axis',(1.,6.75429236703742E-14,-2.77102527463912E-15));
#40139=DIRECTION('',(-2.77102527463854E-15,-8.5680407190582E-15,-1.));
#40140=DIRECTION('center_axis',(-2.77102527463854E-15,-8.5557679050281E-15,
-1.));
#40141=DIRECTION('ref_axis',(0.813826036051037,0.581108581114973,-7.22696266269622E-15));
#40142=DIRECTION('center_axis',(-2.77102527463854E-15,-8.5557679050281E-15,
-1.));
#40143=DIRECTION('ref_axis',(0.813826036051037,0.581108581114973,-7.22696266269622E-15));
#40144=DIRECTION('center_axis',(-6.7618653731838E-14,1.,-8.55576790502791E-15));
#40145=DIRECTION('ref_axis',(-2.77102527463854E-15,-8.5557679050281E-15,
-1.));
#40146=DIRECTION('center_axis',(-6.54569677098685E-14,1.,-5.02820377450251E-15));
#40147=DIRECTION('ref_axis',(-0.504155551068663,-3.73429150937775E-14,-0.8636128648455));
#40148=DIRECTION('',(-2.77102527463854E-15,-8.5557679050281E-15,-1.));
#40149=DIRECTION('',(-1.,-6.7618653731838E-14,2.77102527463912E-15));
#40150=DIRECTION('',(-2.77102527463854E-15,-8.5557679050281E-15,-1.));
#40151=DIRECTION('center_axis',(-2.77102527463854E-15,-8.5557679050281E-15,
-1.));
#40152=DIRECTION('ref_axis',(6.7618653731838E-14,-1.,8.55576790502791E-15));
#40153=DIRECTION('',(-6.7618653731838E-14,1.,-8.55576790502791E-15));
#40154=DIRECTION('',(1.,6.7618653731838E-14,-2.77102527463912E-15));
#40155=DIRECTION('',(0.707106781186496,0.707106781186599,-8.00925226644011E-15));
#40156=DIRECTION('',(-6.7618653731838E-14,1.,-8.55576790502791E-15));
#40157=DIRECTION('',(1.,6.7618653731838E-14,-2.77102527463912E-15));
#40158=DIRECTION('',(6.7618653731838E-14,-1.,8.55576790502791E-15));
#40159=DIRECTION('',(0.707106781186597,-0.707106781186498,4.0904307413668E-15));
#40160=DIRECTION('',(1.,6.90094127104307E-14,-2.77102527463913E-15));
#40161=DIRECTION('',(6.7618653731838E-14,-1.,8.55576790502791E-15));
#40162=DIRECTION('',(-1.,-6.7618653731838E-14,2.77102527463912E-15));
#40163=DIRECTION('',(-0.707106781186496,-0.707106781186599,8.00925226644011E-15));
#40164=DIRECTION('',(6.7618653731838E-14,-1.,8.55576790502791E-15));
#40165=DIRECTION('',(-1.,-6.7618653731838E-14,2.77102527463912E-15));
#40166=DIRECTION('',(-6.7618653731838E-14,1.,-8.55576790502791E-15));
#40167=DIRECTION('',(-0.707106781186595,0.7071067811865,-4.09043074136683E-15));
#40168=DIRECTION('center_axis',(0.707106781186496,0.707106781186599,-8.19011459861798E-15));
#40169=DIRECTION('ref_axis',(-2.76568749322768E-15,-8.8168836495273E-15,
-1.));
#40170=DIRECTION('center_axis',(0.70710678118651,0.707106781186585,2.01699480869601E-13));
#40171=DIRECTION('ref_axis',(-0.0672249759424576,0.0672249759427345,-0.995470544626527));
#40172=DIRECTION('',(-2.77102527463816E-15,-1.41116436776427E-14,-1.));
#40173=DIRECTION('center_axis',(-6.7618653731838E-14,1.,-8.55576790502791E-15));
#40174=DIRECTION('ref_axis',(-2.77102527463854E-15,-8.5557679050281E-15,
-1.));
#40175=DIRECTION('',(2.77102527463854E-15,8.5557679050281E-15,1.));
#40176=DIRECTION('',(-1.,-6.7618653731838E-14,2.77102527463912E-15));
#40177=DIRECTION('',(-2.77102527463854E-15,-8.5557679050281E-15,-1.));
#40178=DIRECTION('',(1.,6.7618653731838E-14,-2.77102527463912E-15));
#40179=DIRECTION('',(2.77102527463854E-15,8.5557679050281E-15,1.));
#40180=DIRECTION('',(-1.,-6.7618653731838E-14,2.77102527463912E-15));
#40181=DIRECTION('center_axis',(6.7618653731838E-14,-1.,8.55576790502791E-15));
#40182=DIRECTION('ref_axis',(2.77102527463854E-15,8.5557679050281E-15,1.));
#40183=DIRECTION('',(2.77102527463854E-15,8.5557679050281E-15,1.));
#40184=DIRECTION('',(1.,6.7618653731838E-14,-2.77102527463912E-15));
#40185=DIRECTION('',(2.77102527463854E-15,8.5557679050281E-15,1.));
#40186=DIRECTION('',(1.,6.7618653731838E-14,-2.77102527463912E-15));
#40187=DIRECTION('',(2.77102527463854E-15,8.5557679050281E-15,1.));
#40188=DIRECTION('',(-1.,-6.7618653731838E-14,2.77102527463912E-15));
#40189=DIRECTION('center_axis',(-2.77102527463854E-15,-8.5557679050281E-15,
-1.));
#40190=DIRECTION('ref_axis',(6.7618653731838E-14,-1.,8.55576790502791E-15));
#40191=DIRECTION('',(-1.,-6.7618653731838E-14,2.77102527463912E-15));
#40192=DIRECTION('center_axis',(7.2574015725158E-16,-8.55576790502786E-15,
-1.));
#40193=DIRECTION('ref_axis',(-5.97509315100852E-14,1.,-8.5557679050279E-15));
#40194=DIRECTION('',(1.,6.7618653731838E-14,-2.77102527463912E-15));
#40195=DIRECTION('center_axis',(4.22250558914198E-15,-8.55576790502776E-15,
-1.));
#40196=DIRECTION('ref_axis',(7.8983141385481E-14,-1.,8.5557679050281E-15));
#40197=DIRECTION('center_axis',(-6.91127211940769E-15,-8.55576790502838E-15,
-1.));
#40198=DIRECTION('ref_axis',(0.811429434660002,0.584450402144912,-1.06084316213848E-14));
#40199=DIRECTION('',(1.,6.7618653731838E-14,-2.77102527463912E-15));
#40200=DIRECTION('center_axis',(9.18710863590449E-15,8.55576790502796E-15,
1.));
#40201=DIRECTION('ref_axis',(9.5991471980432E-14,1.,-8.55576790502884E-15));
#40202=DIRECTION('',(-1.,-6.7618653731838E-14,2.77102527463912E-15));
#40203=DIRECTION('center_axis',(-2.8074595126898E-15,-8.5557679050281E-15,
-1.));
#40204=DIRECTION('ref_axis',(-5.53799747202225E-14,1.,-8.55576790502794E-15));
#40205=DIRECTION('center_axis',(2.77102527463854E-15,8.5557679050281E-15,
1.));
#40206=DIRECTION('ref_axis',(-1.86639376853759E-14,1.,-8.55576790502804E-15));
#40207=DIRECTION('',(2.77102527463854E-15,8.5557679050281E-15,1.));
#40208=DIRECTION('',(2.77102527463854E-15,8.5557679050281E-15,1.));
#40209=DIRECTION('center_axis',(-6.7618653731838E-14,1.,-8.55576790502791E-15));
#40210=DIRECTION('ref_axis',(-2.77102527463854E-15,-8.5557679050281E-15,
-1.));
#40211=DIRECTION('',(-1.,-6.7618653731838E-14,2.77102527463912E-15));
#40212=DIRECTION('',(2.77102527463854E-15,8.5557679050281E-15,1.));
#40213=DIRECTION('center_axis',(-2.8074595126898E-15,-8.5557679050281E-15,
-1.));
#40214=DIRECTION('ref_axis',(6.58702710158929E-14,-1.,8.55576790502791E-15));
#40215=DIRECTION('center_axis',(6.26779070652866E-15,8.55576790502833E-15,
1.));
#40216=DIRECTION('ref_axis',(7.72347586695359E-14,-1.,8.55576790502785E-15));
#40217=DIRECTION('',(2.77102527463854E-15,8.5557679050281E-15,1.));
#40218=DIRECTION('center_axis',(6.7618653731838E-14,-1.,8.55576790502791E-15));
#40219=DIRECTION('ref_axis',(2.77102527463854E-15,8.5557679050281E-15,1.));
#40220=DIRECTION('',(1.,6.7618653731838E-14,-2.77102527463912E-15));
#40221=DIRECTION('center_axis',(-2.77102527463854E-15,-8.5557679050281E-15,
-1.));
#40222=DIRECTION('ref_axis',(6.7618653731838E-14,-1.,8.55576790502791E-15));
#40223=DIRECTION('',(-1.,-6.7618653731838E-14,2.77102527463912E-15));
#40224=DIRECTION('center_axis',(7.257401572517E-16,-8.55576790502786E-15,
-1.));
#40225=DIRECTION('ref_axis',(-6.41218882999477E-14,1.,-8.55576790502791E-15));
#40226=DIRECTION('',(1.,6.7618653731838E-14,-2.77102527463912E-15));
#40227=DIRECTION('center_axis',(-2.77102527463854E-15,-8.5557679050281E-15,
-1.));
#40228=DIRECTION('ref_axis',(6.84928450898106E-14,-1.,8.55576790502791E-15));
#40229=DIRECTION('center_axis',(-5.4767989042709E-15,-1.05258846015543E-14,
-1.));
#40230=DIRECTION('ref_axis',(1.,6.07633997852702E-14,-5.47679890427154E-15));
#40231=DIRECTION('center_axis',(9.18710863590508E-15,8.55576790502853E-15,
1.));
#40232=DIRECTION('ref_axis',(6.44106120512047E-14,-1.,8.55576790502794E-15));
#40233=DIRECTION('center_axis',(-2.80745343291974E-15,-8.5557679050281E-15,
-1.));
#40234=DIRECTION('ref_axis',(-6.7618653731838E-14,1.,-8.55576790502791E-15));
#40235=DIRECTION('center_axis',(2.77102527463854E-15,8.5557679050281E-15,
1.));
#40236=DIRECTION('ref_axis',(-6.67444623738654E-14,1.,-8.55576790502791E-15));
#40237=DIRECTION('',(2.77102527463854E-15,8.5557679050281E-15,1.));
#40238=DIRECTION('',(2.77102527463854E-15,8.5557679050281E-15,1.));
#40239=DIRECTION('center_axis',(-6.7618653731838E-14,1.,-8.55576790502791E-15));
#40240=DIRECTION('ref_axis',(-2.77102527463854E-15,-8.5557679050281E-15,
-1.));
#40241=DIRECTION('',(-1.,-6.7618653731838E-14,2.77102527463912E-15));
#40242=DIRECTION('',(2.77102527463854E-15,8.5557679050281E-15,1.));
#40243=DIRECTION('center_axis',(-2.8074592087013E-15,-8.5557679050281E-15,
-1.));
#40244=DIRECTION('ref_axis',(6.7618653731838E-14,-1.,8.55576790502791E-15));
#40245=DIRECTION('center_axis',(6.2677907065288E-15,8.55576790502833E-15,
1.));
#40246=DIRECTION('ref_axis',(6.7618653731838E-14,-1.,8.55576790502791E-15));
#40247=DIRECTION('',(2.77102527463854E-15,8.5557679050281E-15,1.));
#40248=DIRECTION('center_axis',(6.7618653731838E-14,-1.,8.55576790502791E-15));
#40249=DIRECTION('ref_axis',(2.77102527463854E-15,8.5557679050281E-15,1.));
#40250=DIRECTION('',(1.,6.7618653731838E-14,-2.77102527463912E-15));
#40251=DIRECTION('center_axis',(-2.77102527463854E-15,-8.5557679050281E-15,
-1.));
#40252=DIRECTION('ref_axis',(6.7618653731838E-14,-1.,8.55576790502791E-15));
#40253=DIRECTION('center_axis',(2.77102527463839E-15,1.08315670797044E-14,
1.));
#40254=DIRECTION('ref_axis',(1.,9.26524446532782E-14,-2.77102527463939E-15));
#40255=DIRECTION('center_axis',(-2.77102527463854E-15,-8.5557679050281E-15,
-1.));
#40256=DIRECTION('ref_axis',(1.,6.7618653731838E-14,-2.77102527463912E-15));
#40257=DIRECTION('',(-2.77102527463854E-15,-8.5557679050281E-15,-1.));
#40258=DIRECTION('center_axis',(2.77102527463885E-15,4.00416955567546E-15,
1.));
#40259=DIRECTION('ref_axis',(1.,9.26524446532782E-14,-2.77102527463922E-15));
#40260=DIRECTION('center_axis',(2.77102527463885E-15,4.00416955567546E-15,
1.));
#40261=DIRECTION('ref_axis',(1.,9.26524446532782E-14,-2.77102527463922E-15));
#40262=DIRECTION('center_axis',(1.53398371455475E-14,1.40986148553614E-14,
-1.));
#40263=DIRECTION('ref_axis',(-0.813826036051091,0.581108581114896,-4.29113278354576E-15));
#40264=DIRECTION('',(0.575461908797923,-0.410905818312039,-0.707106781186522));
#40265=DIRECTION('center_axis',(2.77102527463854E-15,8.5557679050281E-15,
1.));
#40266=DIRECTION('ref_axis',(-0.813826036051116,0.581108581114861,-2.71669763258241E-15));
#40267=DIRECTION('center_axis',(-2.77102527463854E-15,-8.5557679050281E-15,
-1.));
#40268=DIRECTION('ref_axis',(6.7618653731838E-14,-1.,8.55576790502791E-15));
#40269=DIRECTION('center_axis',(2.77102527463839E-15,1.08315670797045E-14,
1.));
#40270=DIRECTION('ref_axis',(1.,6.7618653731838E-14,-2.77102527463912E-15));
#40271=DIRECTION('center_axis',(-2.77102527463854E-15,-8.5557679050281E-15,
-1.));
#40272=DIRECTION('ref_axis',(1.,6.7618653731838E-14,-2.77102527463912E-15));
#40273=DIRECTION('',(-2.77102527463854E-15,-8.5557679050281E-15,-1.));
#40274=DIRECTION('center_axis',(2.77102527463885E-15,4.00416955567534E-15,
1.));
#40275=DIRECTION('ref_axis',(1.,6.7618653731838E-14,-2.77102527463912E-15));
#40276=DIRECTION('center_axis',(2.77102527463885E-15,4.00416955567534E-15,
1.));
#40277=DIRECTION('ref_axis',(1.,6.7618653731838E-14,-2.77102527463912E-15));
#40278=DIRECTION('center_axis',(-4.42416735431458E-15,-5.558773389224E-15,
-1.));
#40279=DIRECTION('ref_axis',(-0.813826036051113,0.581108581114866,3.7025166383754E-16));
#40280=DIRECTION('',(0.575461908797911,-0.410905818312022,-0.707106781186542));
#40281=DIRECTION('center_axis',(2.77102527463854E-15,8.5557679050281E-15,
1.));
#40282=DIRECTION('ref_axis',(-0.813826036051116,0.581108581114862,-2.71669763258241E-15));
#40283=DIRECTION('center_axis',(-2.77102527463854E-15,-8.5557679050281E-15,
-1.));
#40284=DIRECTION('ref_axis',(6.7618653731838E-14,-1.,8.55576790502791E-15));
#40285=DIRECTION('center_axis',(2.77102527463839E-15,1.08315670797045E-14,
1.));
#40286=DIRECTION('ref_axis',(1.,5.39638586837799E-14,-2.77102527463897E-15));
#40287=DIRECTION('center_axis',(-2.77102527463854E-15,-8.5557679050281E-15,
-1.));
#40288=DIRECTION('ref_axis',(1.,6.7618653731838E-14,-2.77102527463912E-15));
#40289=DIRECTION('',(-2.77102527463854E-15,-8.5557679050281E-15,-1.));
#40290=DIRECTION('center_axis',(2.77102527463885E-15,4.00416955567533E-15,
1.));
#40291=DIRECTION('ref_axis',(1.,5.39638586837799E-14,-2.77102527463906E-15));
#40292=DIRECTION('center_axis',(2.77102527463885E-15,4.00416955567533E-15,
1.));
#40293=DIRECTION('ref_axis',(1.,5.39638586837799E-14,-2.77102527463906E-15));
#40294=DIRECTION('center_axis',(-3.54887986328151E-14,-8.22998747375855E-15,
-1.));
#40295=DIRECTION('ref_axis',(-0.813826036051127,0.581108581114846,2.40991919720918E-14));
#40296=DIRECTION('',(0.575461908797904,-0.410905818312013,-0.707106781186553));
#40297=DIRECTION('center_axis',(2.77102527463854E-15,8.5557679050281E-15,
1.));
#40298=DIRECTION('ref_axis',(-0.813826036051116,0.581108581114862,-2.71669763258241E-15));
#40299=DIRECTION('center_axis',(-2.77102527463854E-15,-8.5557679050281E-15,
-1.));
#40300=DIRECTION('ref_axis',(6.7618653731838E-14,-1.,8.55576790502791E-15));
#40301=DIRECTION('center_axis',(2.77102527463839E-15,1.08315670797045E-14,
1.));
#40302=DIRECTION('ref_axis',(1.,6.7618653731838E-14,-2.77102527463912E-15));
#40303=DIRECTION('center_axis',(-2.77102527463854E-15,-8.5557679050281E-15,
-1.));
#40304=DIRECTION('ref_axis',(1.,6.7618653731838E-14,-2.77102527463912E-15));
#40305=DIRECTION('',(-2.77102527463854E-15,-8.5557679050281E-15,-1.));
#40306=DIRECTION('center_axis',(2.77102527463885E-15,4.00416955567534E-15,
1.));
#40307=DIRECTION('ref_axis',(1.,6.7618653731838E-14,-2.77102527463912E-15));
#40308=DIRECTION('center_axis',(2.77102527463885E-15,4.00416955567534E-15,
1.));
#40309=DIRECTION('ref_axis',(1.,6.7618653731838E-14,-2.77102527463912E-15));
#40310=DIRECTION('center_axis',(-1.05735999988311E-15,-6.40139923879278E-15,
-1.));
#40311=DIRECTION('ref_axis',(-0.813826036051111,0.581108581114868,-2.8594009314208E-15));
#40312=DIRECTION('',(0.575461908797912,-0.410905818312024,-0.70710678118654));
#40313=DIRECTION('center_axis',(2.77102527463854E-15,8.5557679050281E-15,
1.));
#40314=DIRECTION('ref_axis',(-0.813826036051116,0.581108581114861,-2.71669763258241E-15));
#40315=DIRECTION('center_axis',(3.09929612963862E-15,8.6194655394995E-15,
1.));
#40316=DIRECTION('ref_axis',(0.813826036051036,0.581108581114974,-7.53113327336009E-15));
#40317=DIRECTION('',(0.0142032227504033,0.0101417431418033,-0.999847695156391));
#40318=DIRECTION('center_axis',(-2.87643042720314E-15,-8.58953731699573E-15,
-1.));
#40319=DIRECTION('ref_axis',(0.813826036051037,0.581108581114972,-7.33236781526082E-15));
#40320=DIRECTION('center_axis',(-2.77102527463854E-15,-8.5557679050281E-15,
-1.));
#40321=DIRECTION('ref_axis',(6.7618653731838E-14,-1.,8.55576790502791E-15));
#40322=DIRECTION('center_axis',(2.77102527463854E-15,8.5557679050281E-15,
1.));
#40323=DIRECTION('ref_axis',(-1.,-5.54559913600458E-14,2.77102527463901E-15));
#40324=DIRECTION('center_axis',(2.7710252746384E-15,1.05828783003268E-14,
1.));
#40325=DIRECTION('ref_axis',(1.,6.64679041229712E-14,-2.77102527463911E-15));
#40326=DIRECTION('center_axis',(-2.7710252746384E-15,-1.05828783003268E-14,
-1.));
#40327=DIRECTION('ref_axis',(-1.,-6.80361564334454E-14,2.77102527463912E-15));
#40328=DIRECTION('center_axis',(2.7710252746384E-15,1.05828783003268E-14,
1.));
#40329=DIRECTION('ref_axis',(1.,7.16728745224354E-14,-2.77102527463916E-15));
#40330=DIRECTION('center_axis',(-2.77102527463852E-15,-8.8665914989739E-15,
-1.));
#40331=DIRECTION('ref_axis',(-1.,-6.68051934319591E-14,2.77102527463911E-15));
#40332=DIRECTION('center_axis',(2.77102527463854E-15,8.56804086924424E-15,
1.));
#40333=DIRECTION('ref_axis',(-1.,-6.76736001032872E-14,2.77102527463912E-15));
#40334=DIRECTION('',(-2.77102527463854E-15,-8.56804086924424E-15,-1.));
#40335=DIRECTION('center_axis',(-2.77102527463852E-15,-8.8665914989739E-15,
-1.));
#40336=DIRECTION('ref_axis',(-1.,-6.68051935153285E-14,2.77102527463911E-15));
#40337=DIRECTION('center_axis',(-2.77102527463854E-15,-8.5557679050281E-15,
-1.));
#40338=DIRECTION('ref_axis',(6.7618653731838E-14,-1.,8.55576790502791E-15));
#40339=DIRECTION('center_axis',(-2.77102527463852E-15,-8.89443768051384E-15,
-1.));
#40340=DIRECTION('ref_axis',(-1.,-6.69412911079351E-14,2.77102527463911E-15));
#40341=DIRECTION('center_axis',(2.77102527463854E-15,8.56804054497893E-15,
1.));
#40342=DIRECTION('ref_axis',(-1.,-6.75587848041088E-14,2.77102527463912E-15));
#40343=DIRECTION('',(2.77102527463854E-15,8.56804054497893E-15,1.));
#40344=DIRECTION('center_axis',(-2.77102527463852E-15,-8.89443768051384E-15,
-1.));
#40345=DIRECTION('ref_axis',(-1.,-6.69412911079351E-14,2.77102527463911E-15));
#40346=DIRECTION('center_axis',(-2.77102527463854E-15,-8.5557679050281E-15,
-1.));
#40347=DIRECTION('ref_axis',(6.7618653731838E-14,-1.,8.55576790502791E-15));
#40348=DIRECTION('center_axis',(-2.77102527463845E-15,-9.91373506304373E-15,
-1.));
#40349=DIRECTION('ref_axis',(-1.,-6.57708935439301E-14,2.7710252746391E-15));
#40350=DIRECTION('center_axis',(2.77102527463854E-15,8.56804088631084E-15,
1.));
#40351=DIRECTION('ref_axis',(-1.,-6.74986252505169E-14,2.77102527463912E-15));
#40352=DIRECTION('',(-2.77102527463854E-15,-8.56804088631084E-15,-1.));
#40353=DIRECTION('center_axis',(-2.77102527463845E-15,-9.91373506304373E-15,
-1.));
#40354=DIRECTION('ref_axis',(-1.,-6.60304235712797E-14,2.7710252746391E-15));
#40355=DIRECTION('center_axis',(-2.77102527463854E-15,-8.5557679050281E-15,
-1.));
#40356=DIRECTION('ref_axis',(6.7618653731838E-14,-1.,8.55576790502791E-15));
#40357=DIRECTION('center_axis',(-2.77102527463844E-15,-9.983019101718E-15,
-1.));
#40358=DIRECTION('ref_axis',(-1.,-6.60243977496101E-14,2.7710252746391E-15));
#40359=DIRECTION('center_axis',(2.77102527463854E-15,8.55745189714029E-15,
1.));
#40360=DIRECTION('ref_axis',(-1.,-6.74925013484086E-14,2.77102527463912E-15));
#40361=DIRECTION('',(2.77102527463854E-15,8.55745189714029E-15,1.));
#40362=DIRECTION('center_axis',(-2.77102527463854E-15,-8.5557679050281E-15,
-1.));
#40363=DIRECTION('ref_axis',(6.7618653731838E-14,-1.,8.55576790502791E-15));
#40364=DIRECTION('center_axis',(-2.77102527463854E-15,-8.5557679050281E-15,
-1.));
#40365=DIRECTION('ref_axis',(-1.,-6.35644329412406E-14,2.77102527463908E-15));
#40366=DIRECTION('center_axis',(-2.77102527463854E-15,-8.5557679050281E-15,
-1.));
#40367=DIRECTION('ref_axis',(-1.,-7.07975313971927E-14,2.77102527463915E-15));
#40368=DIRECTION('center_axis',(2.77102527463857E-15,8.11729798613651E-15,
1.));
#40369=DIRECTION('ref_axis',(-1.,-6.7618653731838E-14,2.77102527463912E-15));
#40370=DIRECTION('',(2.77102527463857E-15,8.11729798613651E-15,1.));
#40371=DIRECTION('center_axis',(2.77102527463854E-15,8.5557679050281E-15,
1.));
#40372=DIRECTION('ref_axis',(-1.,-6.7618653731838E-14,2.77102527463912E-15));
#40373=DIRECTION('',(2.77102527463854E-15,8.5557679050281E-15,1.));
#40374=DIRECTION('center_axis',(-2.77102527463833E-15,-1.17346455703829E-14,
-1.));
#40375=DIRECTION('ref_axis',(-1.,-7.07975313971927E-14,2.77102527463916E-15));
#40376=DIRECTION('center_axis',(-2.77102527463854E-15,-8.5557679050281E-15,
-1.));
#40377=DIRECTION('ref_axis',(6.7618653731838E-14,-1.,8.55576790502791E-15));
#40378=DIRECTION('center_axis',(-2.77102527463854E-15,-8.5557679050281E-15,
-1.));
#40379=DIRECTION('ref_axis',(1.,6.66050985341886E-14,-2.77102527463911E-15));
#40380=DIRECTION('center_axis',(2.77102527463854E-15,8.5557679050281E-15,
1.));
#40381=DIRECTION('ref_axis',(1.,7.16728745224354E-14,-2.77102527463915E-15));
#40382=DIRECTION('',(-2.77102527463854E-15,-8.5557679050281E-15,-1.));
#40383=DIRECTION('center_axis',(-2.77102527463854E-15,-8.5557679050281E-15,
-1.));
#40384=DIRECTION('ref_axis',(6.7618653731838E-14,-1.,8.55576790502791E-15));
#40385=DIRECTION('center_axis',(2.77102527463854E-15,8.5557679050281E-15,
1.));
#40386=DIRECTION('ref_axis',(1.,6.7618653731838E-14,-2.77102527463912E-15));
#40387=DIRECTION('center_axis',(-2.77102527463854E-15,-8.5557679050281E-15,
-1.));
#40388=DIRECTION('ref_axis',(1.,6.7618653731838E-14,-2.77102527463912E-15));
#40389=DIRECTION('center_axis',(2.77102527463833E-15,1.17346455703829E-14,
1.));
#40390=DIRECTION('ref_axis',(1.,6.7618653731838E-14,-2.77102527463912E-15));
#40391=DIRECTION('',(-2.77102527463854E-15,-8.5557679050281E-15,-1.));
#40392=DIRECTION('center_axis',(-2.77102527463854E-15,-8.5557679050281E-15,
-1.));
#40393=DIRECTION('ref_axis',(6.7618653731838E-14,-1.,8.55576790502791E-15));
#40394=DIRECTION('center_axis',(-2.77102527463854E-15,-8.5557679050281E-15,
-1.));
#40395=DIRECTION('ref_axis',(6.7618653731838E-14,-1.,8.55576790502791E-15));
#40396=DIRECTION('center_axis',(-2.77102527463833E-15,-1.17346455703829E-14,
-1.));
#40397=DIRECTION('ref_axis',(-1.,-6.90135324843597E-14,2.77102527463914E-15));
#40398=DIRECTION('center_axis',(2.77102527463854E-15,8.56804061665863E-15,
1.));
#40399=DIRECTION('ref_axis',(-1.,-6.64947506794674E-14,2.77102527463911E-15));
#40400=DIRECTION('center_axis',(-2.77102527463854E-15,-8.5557679050281E-15,
-1.));
#40401=DIRECTION('ref_axis',(-1.,-6.94133515893739E-14,2.77102527463913E-15));
#40402=DIRECTION('',(2.77102527463854E-15,8.56804061665863E-15,1.));
#40403=DIRECTION('center_axis',(-2.77102527463854E-15,-8.5557679050281E-15,
-1.));
#40404=DIRECTION('ref_axis',(6.7618653731838E-14,-1.,8.55576790502791E-15));
#40405=DIRECTION('center_axis',(-2.77102527463854E-15,-8.5557679050281E-15,
-1.));
#40406=DIRECTION('ref_axis',(-1.,-6.80361569771588E-14,2.77102527463912E-15));
#40407=DIRECTION('center_axis',(2.77102527463854E-15,8.56804073271148E-15,
1.));
#40408=DIRECTION('ref_axis',(-1.,-6.7618653731838E-14,2.77102527463912E-15));
#40409=DIRECTION('',(2.77102527463854E-15,8.56804073271148E-15,1.));
#40410=DIRECTION('center_axis',(-2.77102527463854E-15,-8.56804074636475E-15,
-1.));
#40411=DIRECTION('ref_axis',(1.,6.8335345472937E-14,-2.77102527463912E-15));
#40412=DIRECTION('center_axis',(2.77102527463854E-15,8.5557679050281E-15,
1.));
#40413=DIRECTION('ref_axis',(1.,6.66124823430948E-14,-2.77102527463911E-15));
#40414=DIRECTION('',(-2.77102527463854E-15,-8.56804074636475E-15,-1.));
#40415=DIRECTION('center_axis',(-2.77102527463854E-15,-8.5557679050281E-15,
-1.));
#40416=DIRECTION('ref_axis',(6.7618653731838E-14,-1.,8.55576790502791E-15));
#40417=DIRECTION('center_axis',(2.77102527463854E-15,8.5557679050281E-15,
1.));
#40418=DIRECTION('ref_axis',(1.,6.85355210440792E-14,-2.77102527463913E-15));
#40419=DIRECTION('center_axis',(-2.77102527463854E-15,-8.56804073953811E-15,
-1.));
#40420=DIRECTION('ref_axis',(1.,6.53708478165727E-14,-2.7710252746391E-15));
#40421=DIRECTION('center_axis',(2.77102527463833E-15,1.17346455703829E-14,
1.));
#40422=DIRECTION('ref_axis',(1.,6.89353399596176E-14,-2.77102527463913E-15));
#40423=DIRECTION('',(-2.77102527463854E-15,-8.56804073953811E-15,-1.));
#40424=DIRECTION('center_axis',(-2.77102527463854E-15,-8.5557679050281E-15,
-1.));
#40425=DIRECTION('ref_axis',(6.7618653731838E-14,-1.,8.55576790502791E-15));
#40426=DIRECTION('center_axis',(6.7618653731838E-14,-1.,8.55576790502791E-15));
#40427=DIRECTION('ref_axis',(2.77102527463854E-15,8.5557679050281E-15,1.));
#40428=DIRECTION('',(9.05427566006634E-15,8.55576790502852E-15,1.));
#40429=DIRECTION('',(1.,6.7618653731838E-14,-2.77102527463912E-15));
#40430=DIRECTION('',(-2.77102527463854E-15,-8.5557679050281E-15,-1.));
#40431=DIRECTION('',(2.77102527463854E-15,8.5557679050281E-15,1.));
#40432=DIRECTION('',(1.,6.7618653731838E-14,-2.77102527463912E-15));
#40433=DIRECTION('center_axis',(-3.71186709412393E-15,-8.55576790502816E-15,
-1.));
#40434=DIRECTION('ref_axis',(6.7618653731838E-14,-1.,8.55576790502791E-15));
#40435=DIRECTION('',(9.05427566006634E-15,8.55576790502852E-15,1.));
#40436=DIRECTION('center_axis',(3.64505808662706E-15,-8.55576790502766E-15,
-1.));
#40437=DIRECTION('ref_axis',(-8.68669038156344E-14,1.,-8.55576790502798E-15));
#40438=DIRECTION('center_axis',(-5.97906695527122E-15,-8.55576790502831E-15,
-1.));
#40439=DIRECTION('ref_axis',(-4.99744244883579E-14,1.,-8.55576790502801E-15));
#40440=DIRECTION('center_axis',(-6.7618653731838E-14,1.,-8.55576790502791E-15));
#40441=DIRECTION('ref_axis',(-2.77102527463854E-15,-8.5557679050281E-15,
-1.));
#40442=DIRECTION('',(2.77102527463854E-15,8.5557679050281E-15,1.));
#40443=DIRECTION('',(-1.,-6.7618653731838E-14,2.77102527463912E-15));
#40444=DIRECTION('',(-1.,-6.7618653731838E-14,2.77102527463912E-15));
#40445=DIRECTION('',(2.77102527463854E-15,8.5557679050281E-15,1.));
#40446=DIRECTION('center_axis',(-2.77102527463854E-15,-8.5557679050281E-15,
-1.));
#40447=DIRECTION('ref_axis',(6.7618653731838E-14,-1.,8.55576790502791E-15));
#40448=DIRECTION('center_axis',(-5.97906695527179E-15,-8.55576790502831E-15,
-1.));
#40449=DIRECTION('ref_axis',(-6.44106120512047E-14,1.,-8.55576790502793E-15));
#40450=DIRECTION('center_axis',(-2.77102527463854E-15,-8.5557679050281E-15,
-1.));
#40451=DIRECTION('ref_axis',(6.92226745721546E-14,-1.,8.5557679050279E-15));
#40452=DIRECTION('center_axis',(2.77102527463854E-15,8.5557679050281E-15,
1.));
#40453=DIRECTION('ref_axis',(-1.,-4.55530009807148E-14,2.77102527463893E-15));
#40454=DIRECTION('center_axis',(-2.63111778409163E-15,-9.17043370360255E-15,
-1.));
#40455=DIRECTION('ref_axis',(-6.7618653731838E-14,1.,-9.17043370360237E-15));
#40456=DIRECTION('center_axis',(-2.77102527463854E-15,-8.5557679050281E-15,
-1.));
#40457=DIRECTION('ref_axis',(6.92226745721546E-14,-1.,8.5557679050279E-15));
#40458=DIRECTION('center_axis',(-2.80745897018724E-15,-8.5557679050281E-15,
-1.));
#40459=DIRECTION('ref_axis',(6.7618653731838E-14,-1.,8.55576790502791E-15));
#40460=DIRECTION('center_axis',(-2.80745897018724E-15,-8.5557679050281E-15,
-1.));
#40461=DIRECTION('ref_axis',(-2.43100910432985E-14,1.,-8.55576790502803E-15));
#40462=DIRECTION('center_axis',(4.3701640599445E-16,-8.55576790502817E-15,
-1.));
#40463=DIRECTION('ref_axis',(5.63905078496234E-14,-1.,8.55576790502819E-15));
#40464=DIRECTION('center_axis',(-2.77102527463854E-15,-8.5557679050281E-15,
-1.));
#40465=DIRECTION('ref_axis',(6.7618653731838E-14,-1.,8.55576790502791E-15));
#40466=DIRECTION('center_axis',(2.77102527463854E-15,8.5557679050281E-15,
1.));
#40467=DIRECTION('ref_axis',(-1.,-6.92565555623126E-14,2.77102527463913E-15));
#40468=DIRECTION('center_axis',(2.75460319106607E-15,8.53296808841364E-15,
1.));
#40469=DIRECTION('ref_axis',(0.811429434660075,-0.58445040214481,2.7519305207226E-15));
#40470=DIRECTION('center_axis',(-7.66431182155099E-14,1.52787649784829E-14,
-1.));
#40471=DIRECTION('ref_axis',(0.811429434660079,-0.584450402144805,-7.11201624201471E-14));
#40472=DIRECTION('center_axis',(1.71148062915242E-14,-8.55576790502675E-15,
-1.));
#40473=DIRECTION('ref_axis',(0.811429434660073,-0.584450402144813,1.88878795861987E-14));
#40474=DIRECTION('center_axis',(2.77102527463854E-15,8.56804068897833E-15,
1.));
#40475=DIRECTION('ref_axis',(-1.,-6.7618653731838E-14,2.77102527463912E-15));
#40476=DIRECTION('',(-2.77102527463854E-15,-8.56804068897833E-15,-1.));
#40477=DIRECTION('center_axis',(-2.77102527463799E-15,-1.6687780537331E-14,
-1.));
#40478=DIRECTION('ref_axis',(-1.,-6.52077354570261E-14,2.77102527463908E-15));
#40479=DIRECTION('center_axis',(2.77102527463854E-15,8.5557679050281E-15,
1.));
#40480=DIRECTION('ref_axis',(-6.7618653731838E-14,1.,-8.55576790502791E-15));
#40481=DIRECTION('center_axis',(-6.99630283644434E-14,1.,0.));
#40482=DIRECTION('ref_axis',(0.,-9.99471833777773E-15,-1.));
#40483=DIRECTION('center_axis',(-1.,-6.7618653731838E-14,2.77102527463912E-15));
#40484=DIRECTION('ref_axis',(7.02309329852463E-15,-0.144413862398959,-0.989517375464936));
#40485=DIRECTION('center_axis',(7.15738251412779E-14,-1.,4.29833232732464E-15));
#40486=DIRECTION('ref_axis',(0.504155551068649,3.23722461609332E-14,-0.863612864845509));
#40487=DIRECTION('center_axis',(-0.707106781186504,-0.707106781186591,-2.23509189115751E-13));
#40488=DIRECTION('ref_axis',(0.067224975942765,-0.0672249759424421,-0.995470544626526));
#40489=DIRECTION('center_axis',(-1.,-6.7618653731838E-14,2.77102527463912E-15));
#40490=DIRECTION('ref_axis',(-2.00277979389365E-14,0.256579164383079,-0.966523218761185));
#40491=DIRECTION('center_axis',(6.7618653731838E-14,-1.,8.55576790502791E-15));
#40492=DIRECTION('ref_axis',(0.144413862399064,1.29898995316941E-15,-0.98951737546492));
#40493=DIRECTION('center_axis',(1.,6.7618653731838E-14,-2.77102527463912E-15));
#40494=DIRECTION('ref_axis',(-3.64834127106881E-14,0.504155551068691,-0.863612864845484));
#40495=DIRECTION('center_axis',(0.707106781186603,-0.707106781186492,-9.33092817933997E-15));
#40496=DIRECTION('ref_axis',(0.0672249759425836,0.0672249759426073,-0.995470544626527));
#40497=DIRECTION('center_axis',(6.86644901853775E-14,-1.,1.10717869485878E-14));
#40498=DIRECTION('ref_axis',(-0.256579164383157,-2.83190166735466E-14,-0.966523218761164));
#40499=DIRECTION('center_axis',(1.,6.76186537318372E-14,-8.87945683687985E-14));
#40500=DIRECTION('ref_axis',(-9.76288392034752E-14,0.144413862399098,-0.989517375464915));
#40501=DIRECTION('center_axis',(1.,1.01085420245098E-13,7.77415841192694E-14));
#40502=DIRECTION('ref_axis',(1.01075458772354E-13,-0.256579164383133,-0.96652321876117));
#40503=DIRECTION('center_axis',(-6.7618653731838E-14,1.,-8.55576790502791E-15));
#40504=DIRECTION('ref_axis',(-0.14441386239907,-1.82311519581102E-14,-0.989517375464919));
#40505=DIRECTION('center_axis',(-1.,-6.7618653731838E-14,2.77102527463912E-15));
#40506=DIRECTION('ref_axis',(3.16972265587057E-14,-0.504155551068665,-0.863612864845499));
#40507=DIRECTION('center_axis',(-0.7071067811866,0.707106781186495,-2.2386518306794E-13));
#40508=DIRECTION('ref_axis',(-0.0672249759424351,-0.0672249759427602,-0.995470544626527));
#40509=DIRECTION('center_axis',(-6.7618653731838E-14,1.,-8.55576790502791E-15));
#40510=DIRECTION('ref_axis',(0.256579164383152,9.08018933668768E-15,-0.966523218761165));
#40511=DIRECTION('center_axis',(2.77102527463854E-15,8.5557679050281E-15,
1.));
#40512=DIRECTION('ref_axis',(-6.7618653731838E-14,1.,-8.55576790502791E-15));
#40513=DIRECTION('center_axis',(1.71148062915315E-14,-8.55576790502675E-15,
-1.));
#40514=DIRECTION('ref_axis',(-0.811429434660146,0.584450402144712,-1.8887879586205E-14));
#40515=DIRECTION('center_axis',(-2.77102527463799E-15,-1.6687780537331E-14,
-1.));
#40516=DIRECTION('ref_axis',(-1.,-6.84069885735319E-14,2.77102527463913E-15));
#40517=DIRECTION('center_axis',(2.77102527463863E-15,7.29513229243521E-15,
1.));
#40518=DIRECTION('ref_axis',(-1.,-6.90562041476608E-14,2.77102527463913E-15));
#40519=DIRECTION('',(-2.77102527463863E-15,-7.29513229243521E-15,-1.));
#40520=DIRECTION('center_axis',(2.75459778662046E-15,8.53296058508019E-15,
1.));
#40521=DIRECTION('ref_axis',(-0.811429434660145,0.584450402144713,-2.75193052072158E-15));
#40522=DIRECTION('center_axis',(-1.27139410577239E-14,-5.34772622439547E-15,
-1.));
#40523=DIRECTION('ref_axis',(-0.81142943466015,0.584450402144707,7.19098526236367E-15));
#40524=DIRECTION('center_axis',(-6.99630283644434E-14,1.,0.));
#40525=DIRECTION('ref_axis',(0.,-9.99471833777773E-15,-1.));
#40526=DIRECTION('center_axis',(-1.,-4.27399845701664E-14,3.45511976547096E-13));
#40527=DIRECTION('ref_axis',(-3.35717857973925E-13,-0.144413862399068,-0.98951737546492));
#40528=DIRECTION('center_axis',(6.77586799616196E-14,-1.,1.15647158182159E-14));
#40529=DIRECTION('ref_axis',(0.504155551068638,2.41734772768401E-14,-0.863612864845515));
#40530=DIRECTION('center_axis',(-0.707106781186505,-0.70710678118659,-2.46996567226803E-13));
#40531=DIRECTION('ref_axis',(0.0672249759428265,-0.0672249759424707,-0.99547054462652));
#40532=DIRECTION('center_axis',(-1.,-3.41518872186049E-14,-7.77415841192225E-14));
#40533=DIRECTION('ref_axis',(6.63763834298554E-14,0.256579164382971,-0.966523218761213));
#40534=DIRECTION('center_axis',(6.7618653731838E-14,-1.,8.55576790502791E-15));
#40535=DIRECTION('ref_axis',(0.144413862399062,1.29898995316927E-15,-0.989517375464921));
#40536=DIRECTION('center_axis',(1.,1.01085420245101E-13,-8.32836346685738E-14));
#40537=DIRECTION('ref_axis',(-1.22887594079545E-13,0.504155551068567,-0.863612864845557));
#40538=DIRECTION('center_axis',(0.707106781186596,-0.707106781186499,6.38249639743397E-13));
#40539=DIRECTION('ref_axis',(0.0672249759431773,0.0672249759422879,-0.995470544626509));
#40540=DIRECTION('center_axis',(6.58951814592576E-14,-1.,6.32142250125411E-15));
#40541=DIRECTION('ref_axis',(-0.256579164383186,-2.3017132218756E-14,-0.966523218761156));
#40542=DIRECTION('center_axis',(1.,6.7618653731838E-14,-2.77102527463912E-15));
#40543=DIRECTION('ref_axis',(-1.25070486127466E-14,0.144413862399052,-0.989517375464922));
#40544=DIRECTION('center_axis',(-6.7618653731838E-14,1.,-8.55576790502791E-15));
#40545=DIRECTION('ref_axis',(-0.504155551068567,-4.14791908661042E-14,-0.863612864845557));
#40546=DIRECTION('center_axis',(0.707106781186503,0.707106781186592,7.20099469180332E-13));
#40547=DIRECTION('ref_axis',(-0.0672249759422375,0.0672249759432429,-0.995470544626508));
#40548=DIRECTION('center_axis',(1.,3.41518872185722E-14,-8.32836346685755E-14));
#40549=DIRECTION('ref_axis',(-7.17329039653535E-14,-0.256579164383119,-0.966523218761174));
#40550=DIRECTION('center_axis',(-6.7618653731838E-14,1.,2.19717498174569E-15));
#40551=DIRECTION('ref_axis',(-0.144413862399068,-7.59092813426568E-15,-0.98951737546492));
#40552=DIRECTION('center_axis',(-1.,-1.01085420245114E-13,-7.77415841193218E-14));
#40553=DIRECTION('ref_axis',(1.18101407927591E-13,-0.504155551068541,-0.863612864845571));
#40554=DIRECTION('center_axis',(-0.707106781186599,0.707106781186496,-9.97176130514017E-14));
#40555=DIRECTION('ref_axis',(-0.0672249759425231,-0.0672249759426732,-0.995470544626527));
#40556=DIRECTION('center_axis',(-6.65728172782997E-14,1.,-1.10717869485855E-14));
#40557=DIRECTION('ref_axis',(0.256579164382955,6.38005866889998E-15,-0.966523218761218));
#40558=DIRECTION('center_axis',(-6.69476735228678E-14,1.,-8.81842604587865E-15));
#40559=DIRECTION('ref_axis',(-2.77102527463852E-15,-8.81842604587884E-15,
-1.));
#40560=DIRECTION('',(-2.77102527463854E-15,-8.5557679050281E-15,-1.));
#40561=DIRECTION('',(-1.,-6.69232742425416E-14,2.77102527463911E-15));
#40562=DIRECTION('',(-2.77102527463854E-15,-8.5557679050281E-15,-1.));
#40563=DIRECTION('center_axis',(1.,6.7618653731838E-14,-2.77102527463912E-15));
#40564=DIRECTION('ref_axis',(6.7618653731838E-14,-1.,8.55576790502791E-15));
#40565=DIRECTION('',(-2.77102527463854E-15,-8.5557679050281E-15,-1.));
#40566=DIRECTION('',(-6.7618653731838E-14,1.,-8.55576790502791E-15));
#40567=DIRECTION('center_axis',(6.68518192073007E-14,-1.,8.85594863742873E-15));
#40568=DIRECTION('ref_axis',(2.77102527463852E-15,8.85594863742892E-15,
1.));
#40569=DIRECTION('',(-2.7710252746385E-15,-9.17308743531861E-15,-1.));
#40570=DIRECTION('',(1.,6.68239343154993E-14,-2.77102527463911E-15));
#40571=DIRECTION('center_axis',(0.707106781186592,-0.707106781186503,4.09043074136686E-15));
#40572=DIRECTION('ref_axis',(2.77102527463854E-15,8.5557679050281E-15,1.));
#40573=DIRECTION('',(-2.77102527463854E-15,-8.5557679050281E-15,-1.));
#40574=DIRECTION('',(0.707106781186499,0.707106781186596,-8.00925226644009E-15));
#40575=DIRECTION('center_axis',(1.,6.7618653731838E-14,-2.77102527463912E-15));
#40576=DIRECTION('ref_axis',(6.7618653731838E-14,-1.,8.55576790502791E-15));
#40577=DIRECTION('',(-2.77102527463854E-15,-8.5557679050281E-15,-1.));
#40578=DIRECTION('',(-6.7618653731838E-14,1.,-8.55576790502791E-15));
#40579=DIRECTION('center_axis',(6.7618653731838E-14,-1.,8.55576790502791E-15));
#40580=DIRECTION('ref_axis',(2.77102527463854E-15,8.5557679050281E-15,1.));
#40581=DIRECTION('',(-2.77102527463854E-15,-8.5557679050281E-15,-1.));
#40582=DIRECTION('',(1.,6.7618653731838E-14,-2.77102527463912E-15));
#40583=DIRECTION('center_axis',(-1.,-6.7618653731838E-14,2.77102527463912E-15));
#40584=DIRECTION('ref_axis',(-6.7618653731838E-14,1.,-8.55576790502791E-15));
#40585=DIRECTION('',(-2.77102527463854E-15,-8.5557679050281E-15,-1.));
#40586=DIRECTION('',(6.7618653731838E-14,-1.,8.55576790502791E-15));
#40587=DIRECTION('center_axis',(-0.7071067811865,-0.707106781186595,8.19011459861795E-15));
#40588=DIRECTION('ref_axis',(2.76568749322768E-15,8.8168836495273E-15,1.));
#40589=DIRECTION('',(-2.77102527463854E-15,-8.5557679050281E-15,-1.));
#40590=DIRECTION('',(0.707106781186594,-0.707106781186501,4.09043074136684E-15));
#40591=DIRECTION('center_axis',(6.96315943587485E-14,-1.,8.5557679050279E-15));
#40592=DIRECTION('ref_axis',(2.77102527463854E-15,8.5557679050281E-15,1.));
#40593=DIRECTION('',(-2.77102527463849E-15,-9.3534957749956E-15,-1.));
#40594=DIRECTION('',(1.,6.97047921997271E-14,-2.77102527463914E-15));
#40595=DIRECTION('center_axis',(-1.,-6.7618653731838E-14,2.77102527463912E-15));
#40596=DIRECTION('ref_axis',(-6.7618653731838E-14,1.,-8.55576790502791E-15));
#40597=DIRECTION('',(-2.77102527463854E-15,-8.5557679050281E-15,-1.));
#40598=DIRECTION('',(6.7618653731838E-14,-1.,8.55576790502791E-15));
#40599=DIRECTION('center_axis',(-6.7618653731838E-14,1.,-8.55576790502791E-15));
#40600=DIRECTION('ref_axis',(-2.77102527463854E-15,-8.5557679050281E-15,
-1.));
#40601=DIRECTION('',(-2.77102527463854E-15,-8.5557679050281E-15,-1.));
#40602=DIRECTION('',(-1.,-6.7618653731838E-14,2.77102527463912E-15));
#40603=DIRECTION('center_axis',(-0.707106781186592,0.707106781186503,-4.09043074136686E-15));
#40604=DIRECTION('ref_axis',(-2.77102527463854E-15,-8.5557679050281E-15,
-1.));
#40605=DIRECTION('',(-2.77102527463854E-15,-8.5557679050281E-15,-1.));
#40606=DIRECTION('',(-0.707106781186497,-0.707106781186598,8.00925226644011E-15));
#40607=DIRECTION('center_axis',(-1.,-6.7618653731838E-14,2.77102527463912E-15));
#40608=DIRECTION('ref_axis',(-6.7618653731838E-14,1.,-8.55576790502791E-15));
#40609=DIRECTION('',(-2.77102527463854E-15,-8.5557679050281E-15,-1.));
#40610=DIRECTION('',(6.7618653731838E-14,-1.,8.55576790502791E-15));
#40611=DIRECTION('center_axis',(-6.7618653731838E-14,1.,-8.55576790502791E-15));
#40612=DIRECTION('ref_axis',(-2.77102527463854E-15,-8.5557679050281E-15,
-1.));
#40613=DIRECTION('',(-2.77102527463854E-15,-8.5557679050281E-15,-1.));
#40614=DIRECTION('',(-1.,-6.7618653731838E-14,2.77102527463912E-15));
#40615=DIRECTION('center_axis',(1.,6.7618653731838E-14,-2.77102527463912E-15));
#40616=DIRECTION('ref_axis',(6.7618653731838E-14,-1.,8.55576790502791E-15));
#40617=DIRECTION('',(-2.77102527463854E-15,-8.5557679050281E-15,-1.));
#40618=DIRECTION('',(-6.7618653731838E-14,1.,-8.55576790502791E-15));
#40619=DIRECTION('center_axis',(0.707106781186493,0.707106781186602,-8.00925226644013E-15));
#40620=DIRECTION('ref_axis',(-2.77102527463854E-15,-8.5557679050281E-15,
-1.));
#40621=DIRECTION('',(-0.707106781186595,0.7071067811865,-4.09043074136683E-15));
#40622=DIRECTION('center_axis',(-2.77102527463854E-15,-8.5557679050281E-15,
-1.));
#40623=DIRECTION('ref_axis',(6.7618653731838E-14,-1.,8.55576790502791E-15));
#40624=DIRECTION('center_axis',(1.,6.7618653731838E-14,-2.77102527463912E-15));
#40625=DIRECTION('ref_axis',(6.7618653731838E-14,-1.,8.55576790502791E-15));
#40626=DIRECTION('',(-2.77102527463854E-15,-8.5557679050281E-15,-1.));
#40627=DIRECTION('center_axis',(6.7618653731838E-14,-1.,8.81842604587865E-15));
#40628=DIRECTION('ref_axis',(2.77102527463852E-15,8.81842604587884E-15,
1.));
#40629=DIRECTION('',(-2.77102527463854E-15,-8.5557679050281E-15,-1.));
#40630=DIRECTION('center_axis',(0.707106781186593,-0.707106781186502,4.29713054957012E-15));
#40631=DIRECTION('ref_axis',(2.7691954317893E-15,8.84625573427986E-15,1.));
#40632=DIRECTION('',(-2.77102527463854E-15,-8.5557679050281E-15,-1.));
#40633=DIRECTION('center_axis',(1.,6.7618653731838E-14,-2.77102527463912E-15));
#40634=DIRECTION('ref_axis',(6.7618653731838E-14,-1.,8.55576790502791E-15));
#40635=DIRECTION('',(-2.77102527463854E-15,-8.5557679050281E-15,-1.));
#40636=DIRECTION('center_axis',(6.7618653731838E-14,-1.,8.55576790502791E-15));
#40637=DIRECTION('ref_axis',(2.77102527463854E-15,8.5557679050281E-15,1.));
#40638=DIRECTION('',(-2.77102527463854E-15,-8.5557679050281E-15,-1.));
#40639=DIRECTION('center_axis',(-1.,-6.7618653731838E-14,2.77102527463912E-15));
#40640=DIRECTION('ref_axis',(-6.7618653731838E-14,1.,-8.55576790502791E-15));
#40641=DIRECTION('',(-2.77102527463854E-15,-8.5557679050281E-15,-1.));
#40642=DIRECTION('center_axis',(-0.707106781186495,-0.7071067811866,8.00925226644012E-15));
#40643=DIRECTION('ref_axis',(2.77102527463854E-15,8.5557679050281E-15,1.));
#40644=DIRECTION('',(-2.77102527463854E-15,-8.5557679050281E-15,-1.));
#40645=DIRECTION('center_axis',(6.89606141497783E-14,-1.,8.55576790502791E-15));
#40646=DIRECTION('ref_axis',(2.77102527463854E-15,8.5557679050281E-15,1.));
#40647=DIRECTION('',(-2.77102527463854E-15,-8.5557679050281E-15,-1.));
#40648=DIRECTION('center_axis',(-1.,-6.7618653731838E-14,2.77102527463912E-15));
#40649=DIRECTION('ref_axis',(-6.7618653731838E-14,1.,-8.55576790502791E-15));
#40650=DIRECTION('',(-2.77102527463854E-15,-8.5557679050281E-15,-1.));
#40651=DIRECTION('center_axis',(-6.7618653731838E-14,1.,-8.81842604587865E-15));
#40652=DIRECTION('ref_axis',(-2.77102527463852E-15,-8.81842604587884E-15,
-1.));
#40653=DIRECTION('',(-2.7710252746385E-15,-9.0959224940323E-15,-1.));
#40654=DIRECTION('center_axis',(-0.70710678118659,0.707106781186505,-4.09043074136688E-15));
#40655=DIRECTION('ref_axis',(-2.77102527463854E-15,-8.5557679050281E-15,
-1.));
#40656=DIRECTION('',(-2.77102527463854E-15,-8.5557679050281E-15,-1.));
#40657=DIRECTION('center_axis',(-1.,-6.7618653731838E-14,2.77102527463912E-15));
#40658=DIRECTION('ref_axis',(-6.7618653731838E-14,1.,-8.55576790502791E-15));
#40659=DIRECTION('',(-2.77102527463854E-15,-8.5557679050281E-15,-1.));
#40660=DIRECTION('center_axis',(-6.7618653731838E-14,1.,-8.55576790502791E-15));
#40661=DIRECTION('ref_axis',(-2.77102527463854E-15,-8.5557679050281E-15,
-1.));
#40662=DIRECTION('',(-2.77102527463854E-15,-8.5557679050281E-15,-1.));
#40663=DIRECTION('center_axis',(1.,6.7618653731838E-14,-2.77102527463912E-15));
#40664=DIRECTION('ref_axis',(6.7618653731838E-14,-1.,8.55576790502791E-15));
#51564=CARTESIAN_POINT('',(0.,0.,0.));
#51565=CARTESIAN_POINT('Ctrl Pts',(376.666251396868,288.32128221579,765.992900062209));
#51566=CARTESIAN_POINT('Ctrl Pts',(377.036265302848,287.705475663881,765.992900062209));
#51567=CARTESIAN_POINT('Ctrl Pts',(377.036265302848,287.705475663881,766.71132055189));
#51568=CARTESIAN_POINT('Ctrl Pts',(377.036265302848,287.705475663881,767.429741041571));
#51569=CARTESIAN_POINT('Ctrl Pts',(376.666251396868,288.32128221579,767.429741041571));
#51570=CARTESIAN_POINT('Ctrl Pts',(376.296237490887,288.937088767699,767.429741041571));
#51571=CARTESIAN_POINT('Ctrl Pts',(376.296237490887,288.937088767699,766.71132055189));
#51572=CARTESIAN_POINT('Ctrl Pts',(376.296237490887,288.937088767699,765.992900062209));
#51573=CARTESIAN_POINT('Ctrl Pts',(376.666251396868,288.32128221579,765.992900062209));
#51574=CARTESIAN_POINT('Ctrl Pts',(376.526601659817,288.237372188339,764.062778007165));
#51575=CARTESIAN_POINT('Ctrl Pts',(377.890701913367,285.967128124481,764.062778007165));
#51576=CARTESIAN_POINT('Ctrl Pts',(377.890701913367,285.967128124481,766.71132055189));
#51577=CARTESIAN_POINT('Ctrl Pts',(377.890701913367,285.967128124481,769.359863096615));
#51578=CARTESIAN_POINT('Ctrl Pts',(376.526601659817,288.237372188339,769.359863096615));
#51579=CARTESIAN_POINT('Ctrl Pts',(375.162501406266,290.507616252197,769.359863096615));
#51580=CARTESIAN_POINT('Ctrl Pts',(375.162501406266,290.507616252197,766.71132055189));
#51581=CARTESIAN_POINT('Ctrl Pts',(375.162501406266,290.507616252197,764.062778007165));
#51582=CARTESIAN_POINT('Ctrl Pts',(376.526601659817,288.237372188339,764.062778007165));
#51583=CARTESIAN_POINT('Ctrl Pts',(375.41696096813,287.570632795434,762.621920551886));
#51584=CARTESIAN_POINT('Ctrl Pts',(377.523157671666,284.065332835937,762.621920551886));
#51585=CARTESIAN_POINT('Ctrl Pts',(377.523157671666,284.065332835938,766.71132055189));
#51586=CARTESIAN_POINT('Ctrl Pts',(377.523157671666,284.065332835938,770.800720551895));
#51587=CARTESIAN_POINT('Ctrl Pts',(375.41696096813,287.570632795435,770.800720551895));
#51588=CARTESIAN_POINT('Ctrl Pts',(373.310764264593,291.075932754932,770.800720551895));
#51589=CARTESIAN_POINT('Ctrl Pts',(373.310764264593,291.075932754932,766.71132055189));
#51590=CARTESIAN_POINT('Ctrl Pts',(373.310764264593,291.075932754931,762.621920551885));
#51591=CARTESIAN_POINT('Ctrl Pts',(375.41696096813,287.570632795434,762.621920551886));
#51592=CARTESIAN_POINT('',(375.855511656978,288.426790399602,763.84112055189));
#51593=CARTESIAN_POINT('',(376.137009774756,288.003281767113,763.84112055189));
#51594=CARTESIAN_POINT('Ctrl Pts',(376.137009774756,288.003281767113,763.84112055189));
#51595=CARTESIAN_POINT('Ctrl Pts',(376.052798999814,288.143432032042,763.84112055189));
#51596=CARTESIAN_POINT('Ctrl Pts',(375.958586636255,288.286094900754,763.84112055189));
#51597=CARTESIAN_POINT('Ctrl Pts',(375.855511656978,288.426790399602,763.84112055189));
#51598=CARTESIAN_POINT('',(375.416960968133,287.570632795437,762.621920551891));
#51599=CARTESIAN_POINT('Ctrl Pts',(376.137009774756,288.003281767113,763.84112055189));
#51600=CARTESIAN_POINT('Ctrl Pts',(375.844583511719,287.827574341685,763.177184192262));
#51601=CARTESIAN_POINT('Ctrl Pts',(375.41696096813,287.570632795434,762.621920551886));
#51602=CARTESIAN_POINT('',(373.310764264593,291.075932754932,766.71132055189));
#51603=CARTESIAN_POINT('Origin',(375.416960968131,287.570632795441,766.71132055189));
#51604=CARTESIAN_POINT('Origin',(375.416960968131,287.570632795441,766.71132055189));
#51605=CARTESIAN_POINT('',(376.378790341087,287.555908422089,763.84112055189));
#51606=CARTESIAN_POINT('Ctrl Pts',(376.378790341087,287.555908422089,763.84112055189));
#51607=CARTESIAN_POINT('Ctrl Pts',(376.302954360659,287.712970762643,763.84112055189));
#51608=CARTESIAN_POINT('Ctrl Pts',(376.221220549696,287.863131502187,763.84112055189));
#51609=CARTESIAN_POINT('Ctrl Pts',(376.137009774756,288.003281767113,763.84112055189));
#51610=CARTESIAN_POINT('',(376.927890738919,287.885841227039,766.20332055189));
#51611=CARTESIAN_POINT('Ctrl Pts',(376.378790341087,287.555908422089,763.84112055189));
#51612=CARTESIAN_POINT('Ctrl Pts',(376.413152024135,287.576555004236,763.918679595973));
#51613=CARTESIAN_POINT('Ctrl Pts',(376.445439414504,287.595955225601,763.995893204523));
#51614=CARTESIAN_POINT('Ctrl Pts',(376.629084043068,287.7063000508,764.460067136705));
#51615=CARTESIAN_POINT('Ctrl Pts',(376.756707472439,287.782983943575,764.903522004224));
#51616=CARTESIAN_POINT('Ctrl Pts',(376.88357350055,287.859212743759,765.639972564748));
#51617=CARTESIAN_POINT('Ctrl Pts',(376.913676025362,287.877300165452,765.925478638303));
#51618=CARTESIAN_POINT('Ctrl Pts',(376.927890738919,287.885841227039,766.20332055189));
#51619=CARTESIAN_POINT('',(377.59541328164,285.531107824361,766.20332055189));
#51620=CARTESIAN_POINT('Ctrl Pts',(376.927890738919,287.885841227039,766.20332055189));
#51621=CARTESIAN_POINT('Ctrl Pts',(377.056775189666,287.639143162358,766.20332055189));
#51622=CARTESIAN_POINT('Ctrl Pts',(377.173719163355,287.37632927026,766.20332055189));
#51623=CARTESIAN_POINT('Ctrl Pts',(377.426153214203,286.668839131006,766.20332055189));
#51624=CARTESIAN_POINT('Ctrl Pts',(377.526925926107,286.212040226457,766.20332055189));
#51625=CARTESIAN_POINT('Ctrl Pts',(377.582348545998,285.703820684751,766.20332055189));
#51626=CARTESIAN_POINT('Ctrl Pts',(377.589829103932,285.618235482969,766.20332055189));
#51627=CARTESIAN_POINT('Ctrl Pts',(377.59541328164,285.531107824361,766.20332055189));
#51628=CARTESIAN_POINT('',(377.59541328164,285.531107824371,767.21932055189));
#51629=CARTESIAN_POINT('Ctrl Pts',(377.59541328164,285.531107824371,766.20332055189));
#51630=CARTESIAN_POINT('Ctrl Pts',(377.609032781063,285.539291245225,766.377007671755));
#51631=CARTESIAN_POINT('Ctrl Pts',(377.615272057358,285.543040180642,766.547816572197));
#51632=CARTESIAN_POINT('Ctrl Pts',(377.615272057358,285.543040180642,766.71132055189));
#51633=CARTESIAN_POINT('Ctrl Pts',(377.615272057358,285.543040180642,766.874824531583));
#51634=CARTESIAN_POINT('Ctrl Pts',(377.609032781063,285.539291245225,767.045633432026));
#51635=CARTESIAN_POINT('Ctrl Pts',(377.59541328164,285.531107824371,767.21932055189));
#51636=CARTESIAN_POINT('',(376.927890738919,287.885841227039,767.21932055189));
#51637=CARTESIAN_POINT('Ctrl Pts',(377.59541328164,285.531107824371,767.21932055189));
#51638=CARTESIAN_POINT('Ctrl Pts',(377.589829103932,285.618235482975,767.21932055189));
#51639=CARTESIAN_POINT('Ctrl Pts',(377.582348545998,285.703820684754,767.219320551891));
#51640=CARTESIAN_POINT('Ctrl Pts',(377.526925926107,286.212040226456,767.21932055189));
#51641=CARTESIAN_POINT('Ctrl Pts',(377.426153214203,286.668839131006,767.21932055189));
#51642=CARTESIAN_POINT('Ctrl Pts',(377.173719163355,287.37632927026,767.21932055189));
#51643=CARTESIAN_POINT('Ctrl Pts',(377.056775189666,287.639143162358,767.21932055189));
#51644=CARTESIAN_POINT('Ctrl Pts',(376.927890738919,287.885841227039,767.21932055189));
#51645=CARTESIAN_POINT('',(376.378790341087,287.555908422089,769.58152055189));
#51646=CARTESIAN_POINT('Ctrl Pts',(376.927890738919,287.885841227039,767.21932055189));
#51647=CARTESIAN_POINT('Ctrl Pts',(376.913676025362,287.877300165452,767.497162465477));
#51648=CARTESIAN_POINT('Ctrl Pts',(376.88357350055,287.859212743759,767.782668539032));
#51649=CARTESIAN_POINT('Ctrl Pts',(376.75670747244,287.782983943575,768.519119099557));
#51650=CARTESIAN_POINT('Ctrl Pts',(376.629084043068,287.7063000508,768.962573967075));
#51651=CARTESIAN_POINT('Ctrl Pts',(376.445439414505,287.595955225601,769.426747899258));
#51652=CARTESIAN_POINT('Ctrl Pts',(376.413152024135,287.576555004236,769.503961507808));
#51653=CARTESIAN_POINT('Ctrl Pts',(376.378790341087,287.555908422089,769.58152055189));
#51654=CARTESIAN_POINT('',(375.855511656978,288.426790399603,769.58152055189));
#51655=CARTESIAN_POINT('Ctrl Pts',(376.378790341087,287.555908422089,769.58152055189));
#51656=CARTESIAN_POINT('Ctrl Pts',(376.302954360659,287.712970762643,769.58152055189));
#51657=CARTESIAN_POINT('Ctrl Pts',(376.221220549696,287.863131502187,769.58152055189));
#51658=CARTESIAN_POINT('Ctrl Pts',(376.137009774756,288.003281767113,769.58152055189));
#51659=CARTESIAN_POINT('Ctrl Pts',(376.052798999814,288.143432032043,769.58152055189));
#51660=CARTESIAN_POINT('Ctrl Pts',(375.958586636254,288.286094900754,769.58152055189));
#51661=CARTESIAN_POINT('Ctrl Pts',(375.855511656978,288.426790399602,769.58152055189));
#51662=CARTESIAN_POINT('',(376.40461205481,288.756723204552,767.21932055189));
#51663=CARTESIAN_POINT('Ctrl Pts',(375.855511656978,288.426790399602,769.58152055189));
#51664=CARTESIAN_POINT('Ctrl Pts',(375.889873340025,288.447436981749,769.50396150781));
#51665=CARTESIAN_POINT('Ctrl Pts',(375.922160730394,288.466837203112,769.426747899263));
#51666=CARTESIAN_POINT('Ctrl Pts',(376.105805358957,288.577182028312,768.962573967082));
#51667=CARTESIAN_POINT('Ctrl Pts',(376.23342878833,288.653865921087,768.519119099562));
#51668=CARTESIAN_POINT('Ctrl Pts',(376.360294816442,288.730094721272,767.782668539035));
#51669=CARTESIAN_POINT('Ctrl Pts',(376.390397341253,288.748182142965,767.497162465479));
#51670=CARTESIAN_POINT('Ctrl Pts',(376.40461205481,288.756723204552,767.21932055189));
#51671=CARTESIAN_POINT('',(374.638888716418,290.451590997326,767.21932055189));
#51672=CARTESIAN_POINT('Ctrl Pts',(376.40461205481,288.756723204552,767.21932055189));
#51673=CARTESIAN_POINT('Ctrl Pts',(376.247298176951,288.986339146055,767.21932055189));
#51674=CARTESIAN_POINT('Ctrl Pts',(376.070149153641,289.212978194765,767.21932055189));
#51675=CARTESIAN_POINT('Ctrl Pts',(375.563983046572,289.768010733646,767.21932055189));
#51676=CARTESIAN_POINT('Ctrl Pts',(375.207963475924,290.071441852646,767.21932055189));
#51677=CARTESIAN_POINT('Ctrl Pts',(374.785251598902,290.358971743954,767.21932055189));
#51678=CARTESIAN_POINT('Ctrl Pts',(374.713196260225,290.40575650301,767.21932055189));
#51679=CARTESIAN_POINT('Ctrl Pts',(374.638888716418,290.451590997326,767.21932055189));
#51680=CARTESIAN_POINT('',(374.638888716425,290.451590997321,766.20332055189));
#51681=CARTESIAN_POINT('Ctrl Pts',(374.638888716425,290.451590997321,767.219320551891));
#51682=CARTESIAN_POINT('Ctrl Pts',(374.652508215849,290.459774418175,767.045633432026));
#51683=CARTESIAN_POINT('Ctrl Pts',(374.658747492148,290.463523353594,766.874824531583));
#51684=CARTESIAN_POINT('Ctrl Pts',(374.658747492148,290.463523353594,766.71132055189));
#51685=CARTESIAN_POINT('Ctrl Pts',(374.658747492147,290.463523353594,766.547816572197));
#51686=CARTESIAN_POINT('Ctrl Pts',(374.652508215849,290.459774418175,766.377007671755));
#51687=CARTESIAN_POINT('Ctrl Pts',(374.638888716425,290.451590997321,766.20332055189));
#51688=CARTESIAN_POINT('',(376.40461205481,288.756723204552,766.20332055189));
#51689=CARTESIAN_POINT('Ctrl Pts',(374.638888716425,290.451590997321,766.20332055189));
#51690=CARTESIAN_POINT('Ctrl Pts',(374.71319626023,290.405756503006,766.20332055189));
#51691=CARTESIAN_POINT('Ctrl Pts',(374.785251598905,290.358971743952,766.20332055189));
#51692=CARTESIAN_POINT('Ctrl Pts',(375.207963475924,290.071441852646,766.20332055189));
#51693=CARTESIAN_POINT('Ctrl Pts',(375.563983046572,289.768010733645,766.20332055189));
#51694=CARTESIAN_POINT('Ctrl Pts',(376.070149153641,289.212978194765,766.20332055189));
#51695=CARTESIAN_POINT('Ctrl Pts',(376.247298176951,288.986339146055,766.20332055189));
#51696=CARTESIAN_POINT('Ctrl Pts',(376.40461205481,288.756723204552,766.20332055189));
#51697=CARTESIAN_POINT('Ctrl Pts',(376.40461205481,288.756723204552,766.20332055189));
#51698=CARTESIAN_POINT('Ctrl Pts',(376.390397341253,288.748182142965,765.925478638302));
#51699=CARTESIAN_POINT('Ctrl Pts',(376.360294816441,288.730094721272,765.639972564745));
#51700=CARTESIAN_POINT('Ctrl Pts',(376.233428788329,288.653865921087,764.903522004218));
#51701=CARTESIAN_POINT('Ctrl Pts',(376.105805358957,288.577182028312,764.460067136698));
#51702=CARTESIAN_POINT('Ctrl Pts',(375.922160730393,288.466837203112,763.995893204517));
#51703=CARTESIAN_POINT('Ctrl Pts',(375.889873340025,288.447436981749,763.91867959597));
#51704=CARTESIAN_POINT('Ctrl Pts',(375.855511656978,288.426790399602,763.841120551891));
#51705=CARTESIAN_POINT('Origin',(376.179793757718,284.535548590652,766.20332055189));
#51706=CARTESIAN_POINT('',(374.764174233796,286.58574918837,766.20332055189));
#51707=CARTESIAN_POINT('',(374.764174233796,286.58574918837,766.20332055189));
#51708=CARTESIAN_POINT('',(375.980797174348,284.560948590652,766.20332055189));
#51709=CARTESIAN_POINT('',(375.980797174348,284.560948590652,766.20332055189));
#51710=CARTESIAN_POINT('',(375.980797174348,284.560948590652,766.20332055189));
#51711=CARTESIAN_POINT('Origin',(376.798034615854,285.051994385647,767.24472055189));
#51712=CARTESIAN_POINT('',(375.980797174348,284.560948590652,767.21932055189));
#51713=CARTESIAN_POINT('',(375.980797174348,284.560948590652,767.21932055189));
#51714=CARTESIAN_POINT('',(375.980797174348,284.560948590652,767.21932055189));
#51715=CARTESIAN_POINT('Origin',(376.179793757718,284.535548590652,767.21932055189));
#51716=CARTESIAN_POINT('',(374.764174233796,286.58574918837,767.21932055189));
#51717=CARTESIAN_POINT('',(374.764174233796,286.58574918837,767.21932055189));
#51718=CARTESIAN_POINT('',(374.764174233796,286.58574918837,767.21932055189));
#51719=CARTESIAN_POINT('Origin',(374.401714623305,284.575195940938,770.826120551892));
#51720=CARTESIAN_POINT('',(373.348616271536,286.327845920685,762.621920551891));
#51721=CARTESIAN_POINT('',(373.348616271535,286.327845920685,770.80072055189));
#51722=CARTESIAN_POINT('Origin',(373.348616271537,286.327845920682,766.711320551889));
#51723=CARTESIAN_POINT('',(373.348616271535,286.327845920685,770.80072055189));
#51724=CARTESIAN_POINT('Origin',(374.382788619834,286.949239358062,766.71132055189));
#51725=CARTESIAN_POINT('',(371.369430483558,289.90946173752,766.71132055189));
#51726=CARTESIAN_POINT('',(372.276591916296,290.454539317553,766.71132055189));
#51727=CARTESIAN_POINT('Ctrl Pts',(371.369430483558,289.90946173752,766.71132055189));
#51728=CARTESIAN_POINT('Ctrl Pts',(371.369430483558,289.90946173752,767.22482239764));
#51729=CARTESIAN_POINT('Ctrl Pts',(371.421402056011,289.820956939152,767.772546668437));
#51730=CARTESIAN_POINT('Ctrl Pts',(371.630749600074,289.459840243892,768.780098710948));
#51731=CARTESIAN_POINT('Ctrl Pts',(371.787896241397,289.187090160201,769.239924587226));
#51732=CARTESIAN_POINT('Ctrl Pts',(372.145703739212,288.554675965553,769.966293840242));
#51733=CARTESIAN_POINT('Ctrl Pts',(372.370204407377,288.152775767151,770.281075771311));
#51734=CARTESIAN_POINT('Ctrl Pts',(372.852983973292,287.267271061198,770.698283099487));
#51735=CARTESIAN_POINT('Ctrl Pts',(373.111025024257,286.783542579163,770.80072055189));
#51736=CARTESIAN_POINT('Ctrl Pts',(373.348616271537,286.327845920683,770.80072055189));
#51737=CARTESIAN_POINT('Ctrl Pts',(373.348616271537,286.327845920683,762.621920551891));
#51738=CARTESIAN_POINT('Ctrl Pts',(373.111002505848,286.783585769154,762.621920551891));
#51739=CARTESIAN_POINT('Ctrl Pts',(372.852938079792,287.267356915581,762.724377271566));
#51740=CARTESIAN_POINT('Ctrl Pts',(372.370121550201,288.152926064257,763.141657334098));
#51741=CARTESIAN_POINT('Ctrl Pts',(372.145607374458,288.554848085829,763.456492730614));
#51742=CARTESIAN_POINT('Ctrl Pts',(371.78782380032,289.18721640002,764.1829137133));
#51743=CARTESIAN_POINT('Ctrl Pts',(371.630703535562,289.459919977806,764.642713966332));
#51744=CARTESIAN_POINT('Ctrl Pts',(371.42139225148,289.820973577177,765.650191762871));
#51745=CARTESIAN_POINT('Ctrl Pts',(371.369430483558,289.90946173752,766.197867412043));
#51746=CARTESIAN_POINT('Ctrl Pts',(371.369430483558,289.90946173752,766.71132055189));
#51747=CARTESIAN_POINT('Origin',(298.461074890948,247.282959303209,725.690320551891));
#51748=CARTESIAN_POINT('',(373.885000951849,285.281359303215,668.66732055189));
#51749=CARTESIAN_POINT('',(376.030529085239,280.683959303215,668.66732055189));
#51750=CARTESIAN_POINT('Origin',(298.461074890937,247.282959303203,668.667320551891));
#51751=CARTESIAN_POINT('',(371.253366994166,290.107359303215,673.49332055189));
#51752=CARTESIAN_POINT('Ctrl Pts',(373.885000951849,285.281359303215,668.66732055189));
#51753=CARTESIAN_POINT('Ctrl Pts',(373.583544656744,285.879727058503,668.66732055189));
#51754=CARTESIAN_POINT('Ctrl Pts',(373.251819248658,286.518714453873,668.784753798678));
#51755=CARTESIAN_POINT('Ctrl Pts',(372.617063345922,287.705592815822,669.271384941794));
#51756=CARTESIAN_POINT('Ctrl Pts',(372.314344533015,288.253640500934,669.640607097597));
#51757=CARTESIAN_POINT('Ctrl Pts',(371.835180640332,289.105328074275,670.492294670938));
#51758=CARTESIAN_POINT('Ctrl Pts',(371.621425700037,289.4764915362,671.022230122432));
#51759=CARTESIAN_POINT('Ctrl Pts',(371.329992690801,289.977829161081,672.209345568074));
#51760=CARTESIAN_POINT('Ctrl Pts',(371.253366994166,290.107359303215,672.867055516681));
#51761=CARTESIAN_POINT('Ctrl Pts',(371.253366994166,290.107359303215,673.49332055189));
#51762=CARTESIAN_POINT('',(371.253366994166,290.107359303215,682.38332055189));
#51763=CARTESIAN_POINT('',(371.253366994166,290.107359303215,673.49332055189));
#51764=CARTESIAN_POINT('',(373.204954482258,286.602159303215,682.38332055189));
#51765=CARTESIAN_POINT('Origin',(298.461074890986,247.282959303229,682.383320551859));
#51766=CARTESIAN_POINT('',(373.204954482258,286.602159303215,686.95532055189));
#51767=CARTESIAN_POINT('Ctrl Pts',(373.204954482258,286.602159303215,686.95532055189));
#51768=CARTESIAN_POINT('Ctrl Pts',(373.356056756597,286.314921256684,686.95532055189));
#51769=CARTESIAN_POINT('Ctrl Pts',(373.5165937577,286.005315992971,686.898068801918));
#51770=CARTESIAN_POINT('Ctrl Pts',(373.811233600901,285.428803143283,686.655970009764));
#51771=CARTESIAN_POINT('Ctrl Pts',(373.945390667172,285.16199362503,686.470955471717));
#51772=CARTESIAN_POINT('Ctrl Pts',(374.143919780962,284.763585698954,686.05428890552));
#51773=CARTESIAN_POINT('Ctrl Pts',(374.226119215438,284.596772075588,685.806126998833));
#51774=CARTESIAN_POINT('Ctrl Pts',(374.335942776093,284.372944317345,685.256268174833));
#51775=CARTESIAN_POINT('Ctrl Pts',(374.363572364748,284.316159303215,684.954479109466));
#51776=CARTESIAN_POINT('Ctrl Pts',(374.363572364748,284.316159303215,684.384161994314));
#51777=CARTESIAN_POINT('Ctrl Pts',(374.335942776093,284.372944317345,684.082372928947));
#51778=CARTESIAN_POINT('Ctrl Pts',(374.226119215438,284.596772075588,683.532514104947));
#51779=CARTESIAN_POINT('Ctrl Pts',(374.143919780962,284.763585698954,683.28435219826));
#51780=CARTESIAN_POINT('Ctrl Pts',(373.945390667172,285.16199362503,682.867685632063));
#51781=CARTESIAN_POINT('Ctrl Pts',(373.811233600901,285.428803143283,682.682671094016));
#51782=CARTESIAN_POINT('Ctrl Pts',(373.5165937577,286.005315992971,682.440572301862));
#51783=CARTESIAN_POINT('Ctrl Pts',(373.356056756597,286.314921256684,682.38332055189));
#51784=CARTESIAN_POINT('Ctrl Pts',(373.204954482258,286.602159303215,682.38332055189));
#51785=CARTESIAN_POINT('',(371.253366994166,290.107359303215,686.95532055189));
#51786=CARTESIAN_POINT('Origin',(298.461074891001,247.282959303238,686.955320551891));
#51787=CARTESIAN_POINT('',(371.253366994166,290.107359303216,777.88732055189));
#51788=CARTESIAN_POINT('',(371.253366994166,290.107359303215,686.95532055189));
#51789=CARTESIAN_POINT('',(373.885000951849,285.281359303216,782.71332055189));
#51790=CARTESIAN_POINT('Ctrl Pts',(371.253366994166,290.107359303216,777.88732055189));
#51791=CARTESIAN_POINT('Ctrl Pts',(371.253366994166,290.107359303216,778.491450416375));
#51792=CARTESIAN_POINT('Ctrl Pts',(371.32472905797,289.986693795228,779.128069862876));
#51793=CARTESIAN_POINT('Ctrl Pts',(371.59833518068,289.516384392817,780.284025646316));
#51794=CARTESIAN_POINT('Ctrl Pts',(371.799607321366,289.167384391968,780.803853655814));
#51795=CARTESIAN_POINT('Ctrl Pts',(372.269123915821,288.335111563991,781.679535597245));
#51796=CARTESIAN_POINT('Ctrl Pts',(372.578867361069,287.775884973468,782.071237654018));
#51797=CARTESIAN_POINT('Ctrl Pts',(373.231303497597,286.5581054402,782.588143904945));
#51798=CARTESIAN_POINT('Ctrl Pts',(373.57365469508,285.899357878152,782.71332055189));
#51799=CARTESIAN_POINT('Ctrl Pts',(373.885000951849,285.281359303216,782.713320551891));
#51800=CARTESIAN_POINT('',(376.03052908524,280.683959303216,782.713320551891));
#51801=CARTESIAN_POINT('Origin',(298.46107489093,247.282959303201,782.71332055193));
#51802=CARTESIAN_POINT('',(376.030529085239,280.683959303215,668.66732055189));
#51803=CARTESIAN_POINT('',(373.348616271535,286.327845920684,721.60092055189));
#51804=CARTESIAN_POINT('',(371.369430483558,289.909461737519,725.69032055189));
#51805=CARTESIAN_POINT('Ctrl Pts',(373.348616271537,286.327845920682,721.60092055189));
#51806=CARTESIAN_POINT('Ctrl Pts',(373.111025024257,286.783542579163,721.60092055189));
#51807=CARTESIAN_POINT('Ctrl Pts',(372.852983973291,287.267271061198,721.703358004293));
#51808=CARTESIAN_POINT('Ctrl Pts',(372.370204407376,288.152775767151,722.120565332469));
#51809=CARTESIAN_POINT('Ctrl Pts',(372.145703739212,288.554675965552,722.435347263539));
#51810=CARTESIAN_POINT('Ctrl Pts',(371.787896241397,289.187090160201,723.161716516554));
#51811=CARTESIAN_POINT('Ctrl Pts',(371.630749600074,289.459840243892,723.621542392832));
#51812=CARTESIAN_POINT('Ctrl Pts',(371.421402056011,289.820956939152,724.629094435343));
#51813=CARTESIAN_POINT('Ctrl Pts',(371.369430483558,289.909461737519,725.17681870614));
#51814=CARTESIAN_POINT('Ctrl Pts',(371.369430483558,289.909461737519,725.69032055189));
#51815=CARTESIAN_POINT('',(373.348616271535,286.327845920685,729.77972055189));
#51816=CARTESIAN_POINT('',(373.348616271535,286.327845920685,729.77972055189));
#51817=CARTESIAN_POINT('Ctrl Pts',(371.369430483558,289.909461737519,725.69032055189));
#51818=CARTESIAN_POINT('Ctrl Pts',(371.369430483558,289.909461737519,726.203773691737));
#51819=CARTESIAN_POINT('Ctrl Pts',(371.42139225148,289.820973577177,726.751449340909));
#51820=CARTESIAN_POINT('Ctrl Pts',(371.630703535562,289.459919977806,727.758927137448));
#51821=CARTESIAN_POINT('Ctrl Pts',(371.78782380032,289.18721640002,728.218727390481));
#51822=CARTESIAN_POINT('Ctrl Pts',(372.145607374458,288.554848085829,728.945148373167));
#51823=CARTESIAN_POINT('Ctrl Pts',(372.3701215502,288.152926064257,729.259983769682));
#51824=CARTESIAN_POINT('Ctrl Pts',(372.852938079792,287.267356915581,729.677263832215));
#51825=CARTESIAN_POINT('Ctrl Pts',(373.111002505848,286.783585769154,729.77972055189));
#51826=CARTESIAN_POINT('Ctrl Pts',(373.348616271537,286.327845920682,729.77972055189));
#51827=CARTESIAN_POINT('Origin',(372.921059816465,286.602159303215,684.66932055189));
#51828=CARTESIAN_POINT('',(371.478547268182,286.602159303215,686.95532055189));
#51829=CARTESIAN_POINT('',(371.478547268182,286.602159303215,686.95532055189));
#51830=CARTESIAN_POINT('',(371.478547268182,286.602159303215,682.38332055189));
#51831=CARTESIAN_POINT('',(371.478547268182,286.602159303215,682.38332055189));
#51832=CARTESIAN_POINT('Ctrl Pts',(371.478547268183,286.602159303215,686.95532055189));
#51833=CARTESIAN_POINT('Ctrl Pts',(371.633224281162,286.314917331796,686.95532055189));
#51834=CARTESIAN_POINT('Ctrl Pts',(371.797603768875,286.005179180258,686.898077083466));
#51835=CARTESIAN_POINT('Ctrl Pts',(372.099402285304,285.428123066717,686.655618593454));
#51836=CARTESIAN_POINT('Ctrl Pts',(372.236875981077,285.160905498426,686.470232722809));
#51837=CARTESIAN_POINT('Ctrl Pts',(372.439838261473,284.762777340855,686.053077926653));
#51838=CARTESIAN_POINT('Ctrl Pts',(372.523732972395,284.596349167931,685.805291976824));
#51839=CARTESIAN_POINT('Ctrl Pts',(372.635876555797,284.372919981108,685.256004081802));
#51840=CARTESIAN_POINT('Ctrl Pts',(372.664126437096,284.316159303215,684.954404613746));
#51841=CARTESIAN_POINT('Ctrl Pts',(372.664126437096,284.316159303215,684.66932055189));
#51842=CARTESIAN_POINT('Ctrl Pts',(372.664126437096,284.316159303215,684.384236490034));
#51843=CARTESIAN_POINT('Ctrl Pts',(372.635876555797,284.372919981108,684.082637021978));
#51844=CARTESIAN_POINT('Ctrl Pts',(372.523732972394,284.596349167931,683.533349126956));
#51845=CARTESIAN_POINT('Ctrl Pts',(372.439838261473,284.762777340855,683.285563177128));
#51846=CARTESIAN_POINT('Ctrl Pts',(372.236875981077,285.160905498426,682.868408380971));
#51847=CARTESIAN_POINT('Ctrl Pts',(372.099402285304,285.428123066717,682.683022510327));
#51848=CARTESIAN_POINT('Ctrl Pts',(371.797603768875,286.005179180258,682.440564020314));
#51849=CARTESIAN_POINT('Ctrl Pts',(371.633224281162,286.314917331796,682.38332055189));
#51850=CARTESIAN_POINT('Ctrl Pts',(371.478547268183,286.602159303215,682.38332055189));
#51851=CARTESIAN_POINT('Origin',(372.92105981647,207.963759303215,684.669320551891));
#51852=CARTESIAN_POINT('',(373.204954482263,207.963759303215,682.383320551891));
#51853=CARTESIAN_POINT('',(373.204954482263,207.963759303215,686.955320551891));
#51854=CARTESIAN_POINT('Ctrl Pts',(373.204954482263,207.963759303215,682.383320551891));
#51855=CARTESIAN_POINT('Ctrl Pts',(373.356056756602,208.250997349746,682.383320551891));
#51856=CARTESIAN_POINT('Ctrl Pts',(373.516593757705,208.56060261346,682.440572301862));
#51857=CARTESIAN_POINT('Ctrl Pts',(373.811233600906,209.137115463147,682.682671094017));
#51858=CARTESIAN_POINT('Ctrl Pts',(373.945390667178,209.4039249814,682.867685632064));
#51859=CARTESIAN_POINT('Ctrl Pts',(374.143919780967,209.802332907476,683.284352198261));
#51860=CARTESIAN_POINT('Ctrl Pts',(374.226119215443,209.969146530842,683.532514104947));
#51861=CARTESIAN_POINT('Ctrl Pts',(374.335942776098,210.192974289085,684.082372928948));
#51862=CARTESIAN_POINT('Ctrl Pts',(374.363572364753,210.249759303215,684.384161994315));
#51863=CARTESIAN_POINT('Ctrl Pts',(374.363572364753,210.249759303215,684.669320551891));
#51864=CARTESIAN_POINT('Ctrl Pts',(374.363572364753,210.249759303215,684.963578716553));
#51865=CARTESIAN_POINT('Ctrl Pts',(374.334175826209,210.189334883116,685.274176295822));
#51866=CARTESIAN_POINT('Ctrl Pts',(374.217956550179,209.952552131374,685.837113369052));
#51867=CARTESIAN_POINT('Ctrl Pts',(374.131115433866,209.776425542292,686.089546516399));
#51868=CARTESIAN_POINT('Ctrl Pts',(373.928262808842,209.369823722155,686.496148336535));
#51869=CARTESIAN_POINT('Ctrl Pts',(373.796344294332,209.107779573834,686.671708057868));
#51870=CARTESIAN_POINT('Ctrl Pts',(373.508153846187,208.544308012748,686.901203447376));
#51871=CARTESIAN_POINT('Ctrl Pts',(373.351837700045,208.24297712921,686.955320551891));
#51872=CARTESIAN_POINT('Ctrl Pts',(373.204954482263,207.963759303215,686.955320551891));
#51873=CARTESIAN_POINT('',(371.478547268188,207.963759303215,686.955320551891));
#51874=CARTESIAN_POINT('',(371.478547268188,207.963759303215,686.955320551891));
#51875=CARTESIAN_POINT('',(371.478547268188,207.963759303215,682.383320551891));
#51876=CARTESIAN_POINT('Ctrl Pts',(371.478547268188,207.963759303215,682.383320551891));
#51877=CARTESIAN_POINT('Ctrl Pts',(371.633224281167,208.251001274634,682.383320551891));
#51878=CARTESIAN_POINT('Ctrl Pts',(371.79760376888,208.560739426172,682.440564020315));
#51879=CARTESIAN_POINT('Ctrl Pts',(372.099402285309,209.137795539713,682.683022510327));
#51880=CARTESIAN_POINT('Ctrl Pts',(372.236875981082,209.405013108004,682.868408380972));
#51881=CARTESIAN_POINT('Ctrl Pts',(372.439838261478,209.803141265575,683.285563177128));
#51882=CARTESIAN_POINT('Ctrl Pts',(372.5237329724,209.969569438499,683.533349126957));
#51883=CARTESIAN_POINT('Ctrl Pts',(372.635876555802,210.192998625322,684.082637021979));
#51884=CARTESIAN_POINT('Ctrl Pts',(372.664126437101,210.249759303215,684.384236490035));
#51885=CARTESIAN_POINT('Ctrl Pts',(372.664126437101,210.249759303215,684.954404613747));
#51886=CARTESIAN_POINT('Ctrl Pts',(372.635876555802,210.192998625322,685.256004081803));
#51887=CARTESIAN_POINT('Ctrl Pts',(372.5237329724,209.969569438499,685.805291976825));
#51888=CARTESIAN_POINT('Ctrl Pts',(372.439838261478,209.803141265575,686.053077926653));
#51889=CARTESIAN_POINT('Ctrl Pts',(372.236875981082,209.405013108004,686.470232722809));
#51890=CARTESIAN_POINT('Ctrl Pts',(372.099402285309,209.137795539713,686.655618593454));
#51891=CARTESIAN_POINT('Ctrl Pts',(371.79760376888,208.560739426172,686.898077083467));
#51892=CARTESIAN_POINT('Ctrl Pts',(371.633224281167,208.251001274634,686.955320551891));
#51893=CARTESIAN_POINT('Ctrl Pts',(371.478547268188,207.963759303215,686.955320551891));
#51894=CARTESIAN_POINT('',(371.478547268188,207.963759303215,682.383320551891));
#51895=CARTESIAN_POINT('Origin',(371.682267445713,209.284559303216,777.887320551891));
#51896=CARTESIAN_POINT('',(373.885000951854,209.284559303216,782.713320551891));
#51897=CARTESIAN_POINT('',(372.174522500194,209.284559303216,782.713320551891));
#51898=CARTESIAN_POINT('',(373.885000951854,209.284559303216,782.713320551891));
#51899=CARTESIAN_POINT('',(369.479533939571,204.458559303216,777.887320551891));
#51900=CARTESIAN_POINT('Ctrl Pts',(369.479533939572,204.458559303216,777.887320551891));
#51901=CARTESIAN_POINT('Ctrl Pts',(369.479533939572,204.458559303216,778.491422612331));
#51902=CARTESIAN_POINT('Ctrl Pts',(369.552676414562,204.579217013025,779.127610628061));
#51903=CARTESIAN_POINT('Ctrl Pts',(369.832513261083,205.048575241124,780.282107787415));
#51904=CARTESIAN_POINT('Ctrl Pts',(370.038186801401,205.396602802461,780.800937575508));
#51905=CARTESIAN_POINT('Ctrl Pts',(370.518643518807,206.22785337804,781.677437375128));
#51906=CARTESIAN_POINT('Ctrl Pts',(370.836280008281,206.787728781571,782.069981441116));
#51907=CARTESIAN_POINT('Ctrl Pts',(371.504957457393,208.006691272921,782.587944800609));
#51908=CARTESIAN_POINT('Ctrl Pts',(371.855654969797,208.665985231776,782.713320551891));
#51909=CARTESIAN_POINT('Ctrl Pts',(372.174522500194,209.284559303216,782.713320551891));
#51910=CARTESIAN_POINT('',(371.253366994172,204.458559303216,777.887320551891));
#51911=CARTESIAN_POINT('',(369.479533939572,204.458559303216,777.887320551891));
#51912=CARTESIAN_POINT('Ctrl Pts',(373.885000951854,209.284559303216,782.713320551891));
#51913=CARTESIAN_POINT('Ctrl Pts',(373.573654695086,208.66656072828,782.713320551891));
#51914=CARTESIAN_POINT('Ctrl Pts',(373.231303497602,208.007813166231,782.588143904945));
#51915=CARTESIAN_POINT('Ctrl Pts',(372.578867361074,206.790033632963,782.071237654019));
#51916=CARTESIAN_POINT('Ctrl Pts',(372.269123915827,206.230807042441,781.679535597245));
#51917=CARTESIAN_POINT('Ctrl Pts',(371.799607321372,205.398534214463,780.803853655815));
#51918=CARTESIAN_POINT('Ctrl Pts',(371.598335180686,205.049534213614,780.284025646317));
#51919=CARTESIAN_POINT('Ctrl Pts',(371.324729057976,204.579224811203,779.128069862876));
#51920=CARTESIAN_POINT('Ctrl Pts',(371.253366994172,204.458559303216,778.491450416376));
#51921=CARTESIAN_POINT('Ctrl Pts',(371.253366994172,204.458559303216,777.887320551891));
#51922=CARTESIAN_POINT('Origin',(371.278766994172,204.458559303215,732.421320551891));
#51923=CARTESIAN_POINT('',(369.479533939571,204.458559303215,686.955320551891));
#51924=CARTESIAN_POINT('',(369.479533939572,204.458559303215,686.955320551891));
#51925=CARTESIAN_POINT('',(371.253366994171,204.458559303215,686.955320551891));
#51926=CARTESIAN_POINT('',(369.479533939571,204.458559303215,686.955320551891));
#51927=CARTESIAN_POINT('',(371.253366994172,204.458559303216,777.887320551891));
#51928=CARTESIAN_POINT('Origin',(371.278766994165,290.107359303215,677.93832055189));
#51929=CARTESIAN_POINT('',(369.479533939565,290.107359303215,682.38332055189));
#51930=CARTESIAN_POINT('',(369.479533939565,290.107359303215,682.38332055189));
#51931=CARTESIAN_POINT('',(369.479533939565,290.107359303215,673.49332055189));
#51932=CARTESIAN_POINT('',(369.479533939565,290.107359303215,673.49332055189));
#51933=CARTESIAN_POINT('',(369.479533939566,290.107359303215,682.38332055189));
#51934=CARTESIAN_POINT('Origin',(374.382788619839,207.616679248369,725.690320551891));
#51935=CARTESIAN_POINT('',(373.34861627154,208.238072685745,721.600920551891));
#51936=CARTESIAN_POINT('',(373.34861627154,208.238072685745,729.779720551891));
#51937=CARTESIAN_POINT('Origin',(373.348616271542,208.238072685748,725.690320551891));
#51938=CARTESIAN_POINT('',(371.369430483564,204.656456868911,725.690320551891));
#51939=CARTESIAN_POINT('Ctrl Pts',(373.348616271542,208.238072685748,729.779720551891));
#51940=CARTESIAN_POINT('Ctrl Pts',(373.111002505853,207.782332837277,729.779720551891));
#51941=CARTESIAN_POINT('Ctrl Pts',(372.852938079797,207.29856169085,729.677263832216));
#51942=CARTESIAN_POINT('Ctrl Pts',(372.370121550206,206.412992542174,729.259983769683));
#51943=CARTESIAN_POINT('Ctrl Pts',(372.145607374464,206.011070520602,728.945148373167));
#51944=CARTESIAN_POINT('Ctrl Pts',(371.787823800326,205.378702206411,728.218727390481));
#51945=CARTESIAN_POINT('Ctrl Pts',(371.630703535568,205.105998628624,727.758927137449));
#51946=CARTESIAN_POINT('Ctrl Pts',(371.421392251486,204.744945029254,726.75144934091));
#51947=CARTESIAN_POINT('Ctrl Pts',(371.369430483564,204.656456868911,726.203773691738));
#51948=CARTESIAN_POINT('Ctrl Pts',(371.369430483564,204.656456868911,725.690320551891));
#51949=CARTESIAN_POINT('',(373.310764264599,203.489985851499,725.690320551891));
#51950=CARTESIAN_POINT('',(372.276591916302,204.111379288878,725.690320551891));
#51951=CARTESIAN_POINT('Origin',(375.416960968136,206.99528581099,725.690320551891));
#51952=CARTESIAN_POINT('Ctrl Pts',(371.369430483564,204.656456868911,725.690320551891));
#51953=CARTESIAN_POINT('Ctrl Pts',(371.369430483564,204.656456868911,725.176818706141));
#51954=CARTESIAN_POINT('Ctrl Pts',(371.421402056017,204.744961667279,724.629094435344));
#51955=CARTESIAN_POINT('Ctrl Pts',(371.63074960008,205.106078362539,723.621542392833));
#51956=CARTESIAN_POINT('Ctrl Pts',(371.787896241403,205.37882844623,723.161716516555));
#51957=CARTESIAN_POINT('Ctrl Pts',(372.145703739218,206.011242640878,722.435347263539));
#51958=CARTESIAN_POINT('Ctrl Pts',(372.370204407382,206.41314283928,722.12056533247));
#51959=CARTESIAN_POINT('Ctrl Pts',(372.852983973297,207.298647545233,721.703358004294));
#51960=CARTESIAN_POINT('Ctrl Pts',(373.111025024262,207.782376027268,721.600920551891));
#51961=CARTESIAN_POINT('Ctrl Pts',(373.348616271542,208.238072685748,721.600920551891));
#51962=CARTESIAN_POINT('Origin',(298.461074890941,247.282959303216,725.690320551891));
#51963=CARTESIAN_POINT('',(376.030529085244,213.881959303216,782.713320551891));
#51964=CARTESIAN_POINT('Origin',(298.461074890966,247.282959303207,782.713320551852));
#51965=CARTESIAN_POINT('Origin',(298.461074890808,247.282959303293,686.955320551891));
#51966=CARTESIAN_POINT('',(371.253366994171,204.458559303215,682.383320551891));
#51967=CARTESIAN_POINT('Origin',(298.461074890893,247.28295930324,682.383320551859));
#51968=CARTESIAN_POINT('',(371.253366994171,204.458559303215,673.493320551891));
#51969=CARTESIAN_POINT('',(371.253366994171,204.458559303215,682.383320551891));
#51970=CARTESIAN_POINT('',(373.885000951854,209.284559303215,668.667320551891));
#51971=CARTESIAN_POINT('Ctrl Pts',(371.253366994171,204.458559303215,673.493320551891));
#51972=CARTESIAN_POINT('Ctrl Pts',(371.253366994171,204.458559303215,672.867055516681));
#51973=CARTESIAN_POINT('Ctrl Pts',(371.329992690807,204.588089445348,672.209345568075));
#51974=CARTESIAN_POINT('Ctrl Pts',(371.621425700043,205.08942707023,671.022230122433));
#51975=CARTESIAN_POINT('Ctrl Pts',(371.835180640338,205.460590532154,670.492294670939));
#51976=CARTESIAN_POINT('Ctrl Pts',(372.314344533021,206.312278105496,669.640607097597));
#51977=CARTESIAN_POINT('Ctrl Pts',(372.617063345927,206.860325790608,669.271384941795));
#51978=CARTESIAN_POINT('Ctrl Pts',(373.251819248663,208.047204152557,668.784753798678));
#51979=CARTESIAN_POINT('Ctrl Pts',(373.58354465675,208.686191547927,668.667320551891));
#51980=CARTESIAN_POINT('Ctrl Pts',(373.885000951854,209.284559303215,668.667320551891));
#51981=CARTESIAN_POINT('',(376.030529085244,213.881959303215,668.667320551891));
#51982=CARTESIAN_POINT('Origin',(298.461074890985,247.282959303195,668.667320551886));
#51983=CARTESIAN_POINT('',(376.030529085244,213.881959303215,668.667320551891));
#51984=CARTESIAN_POINT('',(373.348616271541,208.238072685746,721.600920551891));
#51985=CARTESIAN_POINT('',(373.34861627154,208.238072685745,762.621920551891));
#51986=CARTESIAN_POINT('',(373.34861627154,208.238072685745,770.800720551891));
#51987=CARTESIAN_POINT('',(373.348616271541,208.238072685747,762.621920551891));
#51988=CARTESIAN_POINT('',(371.369430483564,204.656456868912,766.711320551891));
#51989=CARTESIAN_POINT('Ctrl Pts',(371.369430483564,204.656456868912,766.711320551891));
#51990=CARTESIAN_POINT('Ctrl Pts',(371.369430483564,204.656456868912,766.197867412043));
#51991=CARTESIAN_POINT('Ctrl Pts',(371.421392251486,204.744945029254,765.650191762872));
#51992=CARTESIAN_POINT('Ctrl Pts',(371.630703535568,205.105998628625,764.642713966333));
#51993=CARTESIAN_POINT('Ctrl Pts',(371.787823800326,205.378702206411,764.1829137133));
#51994=CARTESIAN_POINT('Ctrl Pts',(372.145607374464,206.011070520602,763.456492730615));
#51995=CARTESIAN_POINT('Ctrl Pts',(372.370121550206,206.412992542174,763.141657334099));
#51996=CARTESIAN_POINT('Ctrl Pts',(372.852938079797,207.29856169085,762.724377271566));
#51997=CARTESIAN_POINT('Ctrl Pts',(373.111002505853,207.782332837278,762.621920551891));
#51998=CARTESIAN_POINT('Ctrl Pts',(373.348616271542,208.238072685749,762.621920551891));
#51999=CARTESIAN_POINT('Ctrl Pts',(373.348616271542,208.238072685749,770.800720551891));
#52000=CARTESIAN_POINT('Ctrl Pts',(373.111025024263,207.782376027268,770.800720551891));
#52001=CARTESIAN_POINT('Ctrl Pts',(372.852983973297,207.298647545233,770.698283099488));
#52002=CARTESIAN_POINT('Ctrl Pts',(372.370204407382,206.41314283928,770.281075771312));
#52003=CARTESIAN_POINT('Ctrl Pts',(372.145703739218,206.011242640879,769.966293840242));
#52004=CARTESIAN_POINT('Ctrl Pts',(371.787896241403,205.37882844623,769.239924587227));
#52005=CARTESIAN_POINT('Ctrl Pts',(371.63074960008,205.106078362539,768.780098710949));
#52006=CARTESIAN_POINT('Ctrl Pts',(371.421402056017,204.744961667279,767.772546668438));
#52007=CARTESIAN_POINT('Ctrl Pts',(371.369430483564,204.656456868912,767.224822397641));
#52008=CARTESIAN_POINT('Ctrl Pts',(371.369430483564,204.656456868912,766.711320551891));
#52009=CARTESIAN_POINT('Origin',(374.401714623309,209.990722665492,729.805120551895));
#52010=CARTESIAN_POINT('Origin',(371.183235802884,209.539164534576,725.690320551891));
#52011=CARTESIAN_POINT('',(374.600804303953,204.137211032768,725.182320551891));
#52012=CARTESIAN_POINT('',(374.600804303953,204.137211032768,726.198320551891));
#52013=CARTESIAN_POINT('Origin',(369.704973520276,207.078922948123,725.690320551891));
#52014=CARTESIAN_POINT('',(376.383495294708,205.82188363143,726.198320551891));
#52015=CARTESIAN_POINT('Origin',(371.183235802884,209.539164534576,726.198320551891));
#52016=CARTESIAN_POINT('',(375.817427244505,206.162011630486,728.560520551891));
#52017=CARTESIAN_POINT('Origin',(370.92159646083,209.10372354582,725.690320551891));
#52018=CARTESIAN_POINT('',(376.340705928614,207.032893607999,728.560520551891));
#52019=CARTESIAN_POINT('Origin',(371.183235802879,209.539164534579,728.560520551891));
#52020=CARTESIAN_POINT('',(376.906773978816,206.692765608943,726.198320551891));
#52021=CARTESIAN_POINT('Origin',(371.444875144938,209.974605523335,725.69032055189));
#52022=CARTESIAN_POINT('',(377.557328869166,209.057694205718,726.198320551891));
#52023=CARTESIAN_POINT('Origin',(371.183235802885,209.539164534576,726.198320551891));
#52024=CARTESIAN_POINT('',(377.557328869166,209.057694205718,725.182320551891));
#52025=CARTESIAN_POINT('Origin',(372.661498085491,211.999406121051,725.690320551891));
#52026=CARTESIAN_POINT('',(376.906773978816,206.692765608943,725.182320551891));
#52027=CARTESIAN_POINT('Origin',(371.183235802886,209.539164534575,725.182320551891));
#52028=CARTESIAN_POINT('',(376.340705928614,207.032893607999,722.820120551891));
#52029=CARTESIAN_POINT('Origin',(371.444875144939,209.974605523334,725.690320551891));
#52030=CARTESIAN_POINT('',(375.817427244505,206.162011630486,722.820120551891));
#52031=CARTESIAN_POINT('Origin',(371.183235802879,209.539164534579,722.820120551889));
#52032=CARTESIAN_POINT('',(376.383495294708,205.82188363143,725.182320551891));
#52033=CARTESIAN_POINT('Origin',(370.92159646083,209.103723545819,725.69032055189));
#52034=CARTESIAN_POINT('Origin',(371.183235802884,209.539164534576,725.182320551891));
#52035=CARTESIAN_POINT('Origin',(377.582728869161,286.21705079407,726.19832055189));
#52036=CARTESIAN_POINT('',(377.557328869161,285.508224400713,726.19832055189));
#52037=CARTESIAN_POINT('',(376.906773978811,287.873152997488,726.19832055189));
#52038=CARTESIAN_POINT('Origin',(371.183235802878,285.026754071854,726.19832055189));
#52039=CARTESIAN_POINT('',(375.980797174348,284.560948590652,726.19832055189));
#52040=CARTESIAN_POINT('',(375.980797174348,284.560948590652,726.19832055189));
#52041=CARTESIAN_POINT('',(374.764174233796,286.58574918837,726.19832055189));
#52042=CARTESIAN_POINT('',(374.764174233796,286.58574918837,726.19832055189));
#52043=CARTESIAN_POINT('',(374.764174233796,286.58574918837,726.19832055189));
#52044=CARTESIAN_POINT('Origin',(376.788427340403,285.046221752173,726.22372055189));
#52045=CARTESIAN_POINT('',(377.557328869161,285.508224400713,725.18232055189));
#52046=CARTESIAN_POINT('Origin',(372.661498085493,282.566512485378,725.69032055189));
#52047=CARTESIAN_POINT('',(375.980797174348,284.560948590652,725.18232055189));
#52048=CARTESIAN_POINT('',(375.980797174348,284.560948590652,725.18232055189));
#52049=CARTESIAN_POINT('',(375.980797174348,284.560948590652,726.19832055189));
#52050=CARTESIAN_POINT('Origin',(374.401714623305,284.575195940938,729.805120551893));
#52051=CARTESIAN_POINT('Origin',(373.348616271537,286.327845920682,725.69032055189));
#52052=CARTESIAN_POINT('Origin',(374.382788619834,286.949239358062,725.69032055189));
#52053=CARTESIAN_POINT('',(373.310764264593,291.075932754932,725.69032055189));
#52054=CARTESIAN_POINT('Origin',(375.416960968131,287.570632795441,725.69032055189));
#52055=CARTESIAN_POINT('',(372.276591916296,290.454539317552,725.69032055189));
#52056=CARTESIAN_POINT('Origin',(374.382788619839,207.61667924837,766.711320551891));
#52057=CARTESIAN_POINT('Origin',(373.348616271542,208.238072685749,766.71132055189));
#52058=CARTESIAN_POINT('',(373.310764264599,203.4899858515,766.711320551891));
#52059=CARTESIAN_POINT('',(372.276591916302,204.111379288879,766.711320551891));
#52060=CARTESIAN_POINT('Origin',(375.416960968136,206.995285810991,766.711320551891));
#52061=CARTESIAN_POINT('Origin',(376.160751551484,206.667365608943,766.203320551891));
#52062=CARTESIAN_POINT('',(377.557328869166,209.057694205718,766.203320551891));
#52063=CARTESIAN_POINT('',(376.906773978816,206.692765608944,766.203320551891));
#52064=CARTESIAN_POINT('Origin',(371.183235802887,209.539164534575,766.20332055189));
#52065=CARTESIAN_POINT('',(375.980797174353,210.00497001578,766.203320551891));
#52066=CARTESIAN_POINT('',(375.980797174353,210.00497001578,766.203320551891));
#52067=CARTESIAN_POINT('',(374.764174233801,207.980169418061,766.203320551891));
#52068=CARTESIAN_POINT('',(374.764174233801,207.980169418061,766.203320551891));
#52069=CARTESIAN_POINT('',(374.764174233801,207.980169418061,766.203320551891));
#52070=CARTESIAN_POINT('Origin',(376.788427340408,209.519696854259,767.244720551891));
#52071=CARTESIAN_POINT('',(377.557328869166,209.057694205718,767.219320551891));
#52072=CARTESIAN_POINT('Origin',(372.661498085491,211.999406121052,766.711320551891));
#52073=CARTESIAN_POINT('',(375.980797174353,210.00497001578,767.219320551891));
#52074=CARTESIAN_POINT('',(375.980797174353,210.00497001578,767.219320551891));
#52075=CARTESIAN_POINT('',(375.980797174353,210.00497001578,766.203320551891));
#52076=CARTESIAN_POINT('Origin',(376.160751551484,206.667365608943,767.219320551891));
#52077=CARTESIAN_POINT('',(376.906773978816,206.692765608944,767.219320551891));
#52078=CARTESIAN_POINT('Origin',(371.183235802884,209.539164534576,767.219320551891));
#52079=CARTESIAN_POINT('',(374.764174233801,207.980169418061,767.219320551891));
#52080=CARTESIAN_POINT('',(374.764174233801,207.980169418061,767.219320551891));
#52081=CARTESIAN_POINT('',(375.980797174353,210.00497001578,767.219320551891));
#52082=CARTESIAN_POINT('Origin',(375.835474106309,207.336467513502,769.606920551891));
#52083=CARTESIAN_POINT('',(376.340705928614,207.032893608,769.581520551891));
#52084=CARTESIAN_POINT('Origin',(371.444875144934,209.974605523338,766.711320551889));
#52085=CARTESIAN_POINT('',(374.764174233801,207.980169418061,769.581520551891));
#52086=CARTESIAN_POINT('',(374.764174233801,207.980169418061,769.581520551891));
#52087=CARTESIAN_POINT('',(374.764174233801,207.980169418061,767.219320551891));
#52088=CARTESIAN_POINT('Origin',(375.290800739153,206.136611630486,769.581520551891));
#52089=CARTESIAN_POINT('',(375.817427244505,206.162011630486,769.581520551891));
#52090=CARTESIAN_POINT('Origin',(371.183235802886,209.539164534575,769.581520551896));
#52091=CARTESIAN_POINT('',(374.240895549693,207.109287440548,769.581520551891));
#52092=CARTESIAN_POINT('',(374.240895549693,207.109287440548,769.581520551891));
#52093=CARTESIAN_POINT('',(374.764174233801,207.980169418061,769.581520551891));
#52094=CARTESIAN_POINT('Origin',(375.3121954222,206.465585535989,769.606920551891));
#52095=CARTESIAN_POINT('',(376.383495294708,205.82188363143,767.219320551891));
#52096=CARTESIAN_POINT('Origin',(370.921596460826,209.103723545823,766.71132055189));
#52097=CARTESIAN_POINT('',(374.240895549693,207.109287440548,767.219320551891));
#52098=CARTESIAN_POINT('',(374.240895549693,207.109287440548,767.219320551891));
#52099=CARTESIAN_POINT('',(374.240895549693,207.109287440548,769.581520551891));
#52100=CARTESIAN_POINT('Origin',(374.703883951924,204.111811032768,767.219320551891));
#52101=CARTESIAN_POINT('',(374.600804303953,204.137211032768,767.219320551891));
#52102=CARTESIAN_POINT('Origin',(371.183235802884,209.539164534577,767.219320551891));
#52103=CARTESIAN_POINT('',(373.02427260914,205.084486842829,767.219320551891));
#52104=CARTESIAN_POINT('',(373.02427260914,205.084486842829,767.219320551891));
#52105=CARTESIAN_POINT('',(374.240895549693,207.109287440548,767.219320551891));
#52106=CARTESIAN_POINT('Origin',(373.831902775195,204.599213681308,767.244720551891));
#52107=CARTESIAN_POINT('',(374.600804303953,204.137211032768,766.203320551891));
#52108=CARTESIAN_POINT('Origin',(369.704973520302,207.07892294808,766.711320551891));
#52109=CARTESIAN_POINT('',(373.02427260914,205.084486842829,766.203320551891));
#52110=CARTESIAN_POINT('',(373.02427260914,205.084486842829,766.203320551891));
#52111=CARTESIAN_POINT('',(373.02427260914,205.084486842829,767.219320551891));
#52112=CARTESIAN_POINT('Origin',(374.703883951924,204.111811032768,766.203320551891));
#52113=CARTESIAN_POINT('',(376.383495294708,205.82188363143,766.203320551891));
#52114=CARTESIAN_POINT('Origin',(371.183235802884,209.539164534576,766.203320551891));
#52115=CARTESIAN_POINT('',(374.240895549693,207.109287440548,766.203320551891));
#52116=CARTESIAN_POINT('',(374.240895549693,207.109287440548,766.203320551891));
#52117=CARTESIAN_POINT('',(373.02427260914,205.084486842829,766.203320551891));
#52118=CARTESIAN_POINT('Origin',(375.3121954222,206.465585535989,766.228720551891));
#52119=CARTESIAN_POINT('',(375.817427244505,206.162011630486,763.841120551891));
#52120=CARTESIAN_POINT('Origin',(370.921596460832,209.103723545819,766.71132055189));
#52121=CARTESIAN_POINT('',(374.240895549693,207.109287440548,763.841120551891));
#52122=CARTESIAN_POINT('',(374.240895549693,207.109287440548,763.841120551891));
#52123=CARTESIAN_POINT('',(374.240895549693,207.109287440548,766.203320551891));
#52124=CARTESIAN_POINT('Origin',(375.290800739153,206.136611630486,763.841120551891));
#52125=CARTESIAN_POINT('',(376.340705928614,207.032893608,763.841120551891));
#52126=CARTESIAN_POINT('Origin',(371.183235802886,209.539164534575,763.841120551891));
#52127=CARTESIAN_POINT('',(374.764174233801,207.980169418061,763.841120551891));
#52128=CARTESIAN_POINT('',(374.764174233801,207.980169418061,763.841120551891));
#52129=CARTESIAN_POINT('',(374.240895549693,207.109287440548,763.841120551891));
#52130=CARTESIAN_POINT('Origin',(375.835474106309,207.336467513502,766.228720551891));
#52131=CARTESIAN_POINT('Origin',(371.44487514494,209.974605523334,766.711320551891));
#52132=CARTESIAN_POINT('',(374.764174233801,207.980169418061,763.841120551891));
#52133=CARTESIAN_POINT('Origin',(374.502534891747,207.544728429305,769.606920551891));
#52134=CARTESIAN_POINT('Origin',(371.183235802883,209.539164534576,766.711320551891));
#52135=CARTESIAN_POINT('Origin',(374.40171462331,209.990722665493,770.826120551895));
#52136=CARTESIAN_POINT('Origin',(371.682267445707,285.281359303215,673.49332055189));
#52137=CARTESIAN_POINT('',(372.174522500188,285.281359303215,668.66732055189));
#52138=CARTESIAN_POINT('Ctrl Pts',(369.479533939566,290.107359303215,673.49332055189));
#52139=CARTESIAN_POINT('Ctrl Pts',(369.479533939566,290.107359303215,672.866062516448));
#52140=CARTESIAN_POINT('Ctrl Pts',(369.558322308944,289.977425390663,672.207866460247));
#52141=CARTESIAN_POINT('Ctrl Pts',(369.857209361088,289.475707577428,671.020898051897));
#52142=CARTESIAN_POINT('Ctrl Pts',(370.076200297233,289.104596282447,670.491562879109));
#52143=CARTESIAN_POINT('Ctrl Pts',(370.566888715326,288.253205154171,669.640171750834));
#52144=CARTESIAN_POINT('Ctrl Pts',(370.877007932881,287.704996235544,669.271056258472));
#52145=CARTESIAN_POINT('Ctrl Pts',(371.526813678761,286.518227155965,668.784638158735));
#52146=CARTESIAN_POINT('Ctrl Pts',(371.866187207677,285.879501788967,668.66732055189));
#52147=CARTESIAN_POINT('Ctrl Pts',(372.174522500189,285.281359303215,668.66732055189));
#52148=CARTESIAN_POINT('',(373.885000951848,285.281359303215,668.66732055189));
#52149=CARTESIAN_POINT('Origin',(428.12807489095,277.381959303219,670.19132055189));
#52150=CARTESIAN_POINT('',(427.36607489095,282.207959303219,670.19132055189));
#52151=CARTESIAN_POINT('',(427.36607489095,277.381959303219,665.36532055189));
#52152=CARTESIAN_POINT('Origin',(427.36607489095,277.381959303219,670.19132055189));
#52153=CARTESIAN_POINT('',(428.89007489095,282.207959303219,670.19132055189));
#52154=CARTESIAN_POINT('',(428.89007489095,282.207959303219,670.19132055189));
#52155=CARTESIAN_POINT('',(428.89007489095,277.381959303219,665.36532055189));
#52156=CARTESIAN_POINT('Origin',(428.89007489095,277.381959303219,670.19132055189));
#52157=CARTESIAN_POINT('',(428.89007489095,277.381959303219,665.36532055189));
#52158=CARTESIAN_POINT('Origin',(428.128074890954,217.158559303219,665.365320551891));
#52159=CARTESIAN_POINT('',(427.366074890954,217.183959303219,665.365320551891));
#52160=CARTESIAN_POINT('',(427.36607489095,277.381959303219,665.36532055189));
#52161=CARTESIAN_POINT('',(428.890074890954,217.183959303219,665.365320551891));
#52162=CARTESIAN_POINT('',(428.89007489095,277.381959303219,665.36532055189));
#52163=CARTESIAN_POINT('',(428.890074890954,217.183959303219,665.365320551891));
#52164=CARTESIAN_POINT('Origin',(428.128074890954,217.183959303219,670.191320551891));
#52165=CARTESIAN_POINT('',(427.366074890954,212.357959303219,670.191320551891));
#52166=CARTESIAN_POINT('Origin',(427.366074890954,217.183959303219,670.191320551891));
#52167=CARTESIAN_POINT('',(428.890074890954,212.357959303219,670.191320551891));
#52168=CARTESIAN_POINT('Origin',(428.890074890954,217.183959303219,670.19132055189));
#52169=CARTESIAN_POINT('',(428.890074890954,212.357959303219,670.191320551891));
#52170=CARTESIAN_POINT('Origin',(428.915474890955,212.357959303219,725.690320551891));
#52171=CARTESIAN_POINT('',(427.366074890955,212.35795930322,781.189320551891));
#52172=CARTESIAN_POINT('',(427.366074890954,212.357959303219,670.191320551891));
#52173=CARTESIAN_POINT('',(428.890074890955,212.35795930322,781.189320551891));
#52174=CARTESIAN_POINT('',(428.890074890954,212.357959303219,670.191320551891));
#52175=CARTESIAN_POINT('',(428.890074890955,212.35795930322,781.189320551891));
#52176=CARTESIAN_POINT('Origin',(428.128074890954,217.18395930322,781.189320551891));
#52177=CARTESIAN_POINT('',(427.366074890954,217.183959375133,786.015320551891));
#52178=CARTESIAN_POINT('Origin',(427.366074890954,217.183959303219,781.189320551891));
#52179=CARTESIAN_POINT('',(428.890074890954,217.183959375133,786.015320551891));
#52180=CARTESIAN_POINT('Origin',(428.890074890954,217.18395930322,781.189320551891));
#52181=CARTESIAN_POINT('',(428.890074890954,217.183959375133,786.015320551891));
#52182=CARTESIAN_POINT('Origin',(428.128074890955,217.158559375133,786.015320551891));
#52183=CARTESIAN_POINT('',(427.36607489095,277.38195930322,786.01532055189));
#52184=CARTESIAN_POINT('',(427.366074890954,217.183959375133,786.015320551891));
#52185=CARTESIAN_POINT('',(428.89007489095,277.38195930322,786.01532055189));
#52186=CARTESIAN_POINT('',(428.890074890954,217.183959375133,786.015320551891));
#52187=CARTESIAN_POINT('',(428.89007489095,277.38195930322,786.01532055189));
#52188=CARTESIAN_POINT('Origin',(428.12807489095,277.381959303219,781.18932055189));
#52189=CARTESIAN_POINT('',(427.36607489095,282.20795930322,781.18932055189));
#52190=CARTESIAN_POINT('Origin',(427.36607489095,277.38195930322,781.18932055189));
#52191=CARTESIAN_POINT('',(428.89007489095,282.20795930322,781.18932055189));
#52192=CARTESIAN_POINT('Origin',(428.89007489095,277.38195930322,781.18932055189));
#52193=CARTESIAN_POINT('',(428.89007489095,282.20795930322,781.18932055189));
#52194=CARTESIAN_POINT('Origin',(428.91547489095,282.207959303219,725.69032055189));
#52195=CARTESIAN_POINT('',(427.36607489095,282.20795930322,781.18932055189));
#52196=CARTESIAN_POINT('',(428.89007489095,282.20795930322,781.18932055189));
#52197=CARTESIAN_POINT('Origin',(427.366074890955,212.332559303219,725.690320566784));
#52198=CARTESIAN_POINT('',(427.36607489095,280.683959303219,668.66732055189));
#52199=CARTESIAN_POINT('',(427.36607489095,280.68395930322,782.71332055189));
#52200=CARTESIAN_POINT('',(427.36607489095,280.683959303219,668.66732055189));
#52201=CARTESIAN_POINT('',(427.366074890955,213.88195930322,782.713320551891));
#52202=CARTESIAN_POINT('',(427.36607489095,280.68395930322,782.71332055189));
#52203=CARTESIAN_POINT('',(427.366074890954,213.881959303219,668.667320551891));
#52204=CARTESIAN_POINT('',(427.366074890954,213.881959303219,668.667320551891));
#52205=CARTESIAN_POINT('',(427.36607489095,280.683959303219,668.66732055189));
#52206=CARTESIAN_POINT('Origin',(428.890074890955,212.332559303219,725.690320566784));
#52207=CARTESIAN_POINT('',(428.890074890954,220.231959303219,679.10672055189));
#52208=CARTESIAN_POINT('Origin',(428.890074890954,220.231959303219,675.017320551891));
#52209=CARTESIAN_POINT('',(428.890074890951,274.33395930322,780.45272055189));
#52210=CARTESIAN_POINT('Origin',(428.89007489095,274.33395930322,776.36332055189));
#52211=CARTESIAN_POINT('',(428.89007489095,279.032959303219,740.16832055189));
#52212=CARTESIAN_POINT('',(428.89007489095,279.032959303219,711.21232055189));
#52213=CARTESIAN_POINT('',(428.89007489095,279.032959303219,740.16832055189));
#52214=CARTESIAN_POINT('',(428.89007489095,275.984959303219,708.16432055189));
#52215=CARTESIAN_POINT('Origin',(428.89007489095,275.984959303219,711.21232055189));
#52216=CARTESIAN_POINT('',(428.890074890954,218.580959303219,708.164320551891));
#52217=CARTESIAN_POINT('',(428.89007489095,275.984959303219,708.16432055189));
#52218=CARTESIAN_POINT('',(428.890074890954,215.532959303219,711.212320551891));
#52219=CARTESIAN_POINT('Origin',(428.890074890954,218.580959303219,711.212320551891));
#52220=CARTESIAN_POINT('',(428.890074890954,215.532959303219,740.168320551891));
#52221=CARTESIAN_POINT('',(428.890074890954,215.532959303219,711.212320551891));
#52222=CARTESIAN_POINT('',(428.890074890954,218.580959303219,743.216320551891));
#52223=CARTESIAN_POINT('Origin',(428.890074890954,218.580959303219,740.168320551891));
#52224=CARTESIAN_POINT('',(428.89007489095,275.984959303219,743.21632055189));
#52225=CARTESIAN_POINT('',(428.890074890954,218.580959303219,743.216320551891));
#52226=CARTESIAN_POINT('Origin',(428.89007489095,275.984959303219,740.16832055189));
#52227=CARTESIAN_POINT('Origin',(429.41077489095,275.984959303219,711.21232055189));
#52228=CARTESIAN_POINT('',(429.93147489095,279.032959303219,711.21232055189));
#52229=CARTESIAN_POINT('',(429.93147489095,279.032959303219,711.21232055189));
#52230=CARTESIAN_POINT('',(429.93147489095,275.984959303219,708.16432055189));
#52231=CARTESIAN_POINT('Origin',(429.93147489095,275.984959303219,711.21232055189));
#52232=CARTESIAN_POINT('',(429.93147489095,275.984959303219,708.16432055189));
#52233=CARTESIAN_POINT('Origin',(429.410774890954,218.555559303219,708.164320551891));
#52234=CARTESIAN_POINT('',(429.931474890954,218.580959303219,708.164320551891));
#52235=CARTESIAN_POINT('',(429.93147489095,275.984959303219,708.16432055189));
#52236=CARTESIAN_POINT('',(429.931474890954,218.580959303219,708.164320551891));
#52237=CARTESIAN_POINT('Origin',(429.410774890954,218.580959303219,711.21232055189));
#52238=CARTESIAN_POINT('',(429.931474890954,215.532959303219,711.212320551891));
#52239=CARTESIAN_POINT('Origin',(429.931474890954,218.580959303219,711.212320551891));
#52240=CARTESIAN_POINT('',(429.931474890954,215.532959303219,711.212320551891));
#52241=CARTESIAN_POINT('Origin',(429.956874890954,215.532959303219,725.690320551891));
#52242=CARTESIAN_POINT('',(429.931474890954,215.532959303219,740.168320551891));
#52243=CARTESIAN_POINT('',(429.931474890954,215.532959303219,711.212320551891));
#52244=CARTESIAN_POINT('',(429.931474890954,215.532959303219,740.168320551891));
#52245=CARTESIAN_POINT('Origin',(429.410774890954,218.580959303219,740.168320551891));
#52246=CARTESIAN_POINT('',(429.931474890954,218.580959303219,743.216320551891));
#52247=CARTESIAN_POINT('Origin',(429.931474890954,218.580959303219,740.168320551891));
#52248=CARTESIAN_POINT('',(429.931474890954,218.580959303219,743.216320551891));
#52249=CARTESIAN_POINT('Origin',(429.410774890954,218.555559303219,743.216320551891));
#52250=CARTESIAN_POINT('',(429.93147489095,275.984959303219,743.21632055189));
#52251=CARTESIAN_POINT('',(429.931474890954,218.580959303219,743.216320551891));
#52252=CARTESIAN_POINT('',(429.93147489095,275.984959303219,743.21632055189));
#52253=CARTESIAN_POINT('Origin',(429.41077489095,275.984959303219,740.16832055189));
#52254=CARTESIAN_POINT('',(429.93147489095,279.032959303219,740.16832055189));
#52255=CARTESIAN_POINT('Origin',(429.93147489095,275.984959303219,740.16832055189));
#52256=CARTESIAN_POINT('',(429.93147489095,279.032959303219,740.16832055189));
#52257=CARTESIAN_POINT('Origin',(429.95687489095,279.032959303219,725.69032055189));
#52258=CARTESIAN_POINT('',(429.93147489095,279.032959303219,740.16832055189));
#52259=CARTESIAN_POINT('Origin',(429.931474890954,215.507559303219,725.690320551891));
#52260=CARTESIAN_POINT('Origin',(426.353194189194,274.333959303219,776.36332055189));
#52261=CARTESIAN_POINT('',(431.404674890951,274.33395930322,780.45272055189));
#52262=CARTESIAN_POINT('Origin',(431.404674890951,274.33395930322,776.36332055189));
#52263=CARTESIAN_POINT('',(432.812646305297,274.33395930322,775.644900062204));
#52264=CARTESIAN_POINT('',(432.162199060962,272.663631664701,773.974572423685));
#52265=CARTESIAN_POINT('Origin',(426.353194189182,274.693169548068,776.004110307046));
#52266=CARTESIAN_POINT('',(432.162199060962,271.945211175015,774.692992913371));
#52267=CARTESIAN_POINT('Origin',(426.353194189229,272.304421419856,774.333782668527));
#52268=CARTESIAN_POINT('',(432.812646305297,273.615538813534,776.36332055189));
#52269=CARTESIAN_POINT('Origin',(426.35319418918,273.974749058382,776.722530796734));
#52270=CARTESIAN_POINT('',(432.162199060962,271.945211175015,778.033648190409));
#52271=CARTESIAN_POINT('Origin',(426.353194189181,273.974749058382,776.004110307047));
#52272=CARTESIAN_POINT('',(432.162199060962,272.663631664701,778.752068680094));
#52273=CARTESIAN_POINT('Origin',(426.353194189236,272.30442141982,778.392858435289));
#52274=CARTESIAN_POINT('',(432.812646305297,274.33395930322,777.081741041575));
#52275=CARTESIAN_POINT('Origin',(426.35319418918,274.693169548067,776.722530796732));
#52276=CARTESIAN_POINT('',(432.162199060961,276.004286941739,778.752068680094));
#52277=CARTESIAN_POINT('Origin',(426.35319418918,273.97474905837,776.722530796732));
#52278=CARTESIAN_POINT('',(432.162199060961,276.722707431424,778.033648190409));
#52279=CARTESIAN_POINT('Origin',(426.35319418923,276.363497186619,778.39285843529));
#52280=CARTESIAN_POINT('',(432.812646305296,275.052379792905,776.36332055189));
#52281=CARTESIAN_POINT('Origin',(426.35319418918,274.693169548057,776.004110307047));
#52282=CARTESIAN_POINT('',(432.162199060961,276.722707431424,774.692992913371));
#52283=CARTESIAN_POINT('Origin',(426.35319418918,274.693169548056,776.722530796733));
#52284=CARTESIAN_POINT('',(432.162199060961,276.004286941739,773.974572423685));
#52285=CARTESIAN_POINT('Origin',(426.353194189222,276.363497186581,774.333782668528));
#52286=CARTESIAN_POINT('Origin',(426.353194189182,273.974749058371,776.004110307047));
#52287=CARTESIAN_POINT('Origin',(430.147374890951,274.33395930322,776.36332055189));
#52288=CARTESIAN_POINT('',(430.147374890951,274.33395930322,780.45272055189));
#52289=CARTESIAN_POINT('Origin',(426.353194189198,220.231959303218,675.01732055189));
#52290=CARTESIAN_POINT('',(431.404674890954,220.231959303219,679.10672055189));
#52291=CARTESIAN_POINT('Origin',(431.404674890954,220.231959303219,675.017320551891));
#52292=CARTESIAN_POINT('',(432.8126463053,220.231959303219,674.298900062205));
#52293=CARTESIAN_POINT('',(432.162199060965,218.5616316647,672.628572423686));
#52294=CARTESIAN_POINT('Origin',(426.353194189186,220.591169548065,674.658110307049));
#52295=CARTESIAN_POINT('',(432.162199060965,217.843211175014,673.346992913372));
#52296=CARTESIAN_POINT('Origin',(426.35319418923,218.202421419857,672.987782668529));
#52297=CARTESIAN_POINT('',(432.8126463053,219.513538813533,675.017320551891));
#52298=CARTESIAN_POINT('Origin',(426.353194189188,219.872749058377,675.376530796737));
#52299=CARTESIAN_POINT('',(432.162199060965,217.843211175015,676.687648190409));
#52300=CARTESIAN_POINT('Origin',(426.353194189187,219.872749058378,674.658110307044));
#52301=CARTESIAN_POINT('',(432.162199060965,218.5616316647,677.406068680095));
#52302=CARTESIAN_POINT('Origin',(426.353194189245,218.202421419855,677.046858435254));
#52303=CARTESIAN_POINT('',(432.8126463053,220.231959303219,675.735741041576));
#52304=CARTESIAN_POINT('Origin',(426.353194189186,220.591169548064,675.376530796731));
#52305=CARTESIAN_POINT('',(432.162199060965,221.902286941738,677.406068680095));
#52306=CARTESIAN_POINT('Origin',(426.353194189186,219.872749058373,675.376530796731));
#52307=CARTESIAN_POINT('',(432.162199060965,222.620707431423,676.687648190409));
#52308=CARTESIAN_POINT('Origin',(426.35319418924,222.261497186587,677.046858435259));
#52309=CARTESIAN_POINT('',(432.8126463053,220.950379792904,675.017320551891));
#52310=CARTESIAN_POINT('Origin',(426.353194189186,220.591169548059,674.658110307044));
#52311=CARTESIAN_POINT('',(432.162199060965,222.620707431423,673.346992913372));
#52312=CARTESIAN_POINT('Origin',(426.353194189186,220.591169548059,675.376530796737));
#52313=CARTESIAN_POINT('',(432.162199060965,221.902286941738,672.628572423686));
#52314=CARTESIAN_POINT('Origin',(426.353194189235,222.26149718658,672.987782668529));
#52315=CARTESIAN_POINT('Origin',(426.353194189186,219.872749058373,674.658110307051));
#52316=CARTESIAN_POINT('Origin',(430.147374890954,220.231959303219,675.017320551891));
#52317=CARTESIAN_POINT('',(430.147374890954,220.231959303219,679.10672055189));
#52318=CARTESIAN_POINT('Origin',(432.232023881687,222.26149718658,672.987782668529));
#52319=CARTESIAN_POINT('',(430.312474890954,222.620707431423,673.346992913372));
#52320=CARTESIAN_POINT('',(430.312474890954,222.620707431423,673.346992913372));
#52321=CARTESIAN_POINT('',(430.312474890954,221.902286941738,672.628572423686));
#52322=CARTESIAN_POINT('',(430.312474890954,222.620707431423,673.346992913372));
#52323=CARTESIAN_POINT('',(430.312474890954,221.902286941738,672.628572423686));
#52324=CARTESIAN_POINT('Origin',(432.8380463053,221.067123122478,673.463736242946));
#52325=CARTESIAN_POINT('',(430.312474890954,220.231959303219,674.298900062205));
#52326=CARTESIAN_POINT('',(430.312474890954,221.902286941738,672.628572423686));
#52327=CARTESIAN_POINT('',(430.312474890954,220.231959303219,674.298900062205));
#52328=CARTESIAN_POINT('Origin',(432.8380463053,219.39679548396,673.463736242946));
#52329=CARTESIAN_POINT('',(430.312474890954,218.5616316647,672.628572423686));
#52330=CARTESIAN_POINT('',(430.312474890954,220.231959303219,674.298900062205));
#52331=CARTESIAN_POINT('',(430.312474890954,218.5616316647,672.628572423686));
#52332=CARTESIAN_POINT('Origin',(432.232023881687,218.202421419857,672.987782668529));
#52333=CARTESIAN_POINT('',(430.312474890954,217.843211175014,673.346992913372));
#52334=CARTESIAN_POINT('',(430.312474890954,218.5616316647,672.628572423686));
#52335=CARTESIAN_POINT('',(430.312474890954,217.843211175014,673.346992913372));
#52336=CARTESIAN_POINT('Origin',(432.8380463053,218.678374994274,674.182156732631));
#52337=CARTESIAN_POINT('',(430.312474890954,219.513538813533,675.017320551891));
#52338=CARTESIAN_POINT('',(430.312474890954,217.843211175014,673.346992913372));
#52339=CARTESIAN_POINT('',(430.312474890954,219.513538813533,675.017320551891));
#52340=CARTESIAN_POINT('Origin',(432.8380463053,218.678374994274,675.85248437115));
#52341=CARTESIAN_POINT('',(430.312474890954,217.843211175014,676.687648190409));
#52342=CARTESIAN_POINT('',(430.312474890954,219.513538813533,675.017320551891));
#52343=CARTESIAN_POINT('',(430.312474890954,217.843211175014,676.687648190409));
#52344=CARTESIAN_POINT('Origin',(432.232023881687,218.202421419857,677.046858435252));
#52345=CARTESIAN_POINT('',(430.312474890954,218.5616316647,677.406068680095));
#52346=CARTESIAN_POINT('',(430.312474890954,217.843211175014,676.687648190409));
#52347=CARTESIAN_POINT('',(430.312474890954,218.5616316647,677.406068680095));
#52348=CARTESIAN_POINT('Origin',(432.8380463053,219.396795483959,676.570904860836));
#52349=CARTESIAN_POINT('',(430.312474890954,220.231959303219,675.735741041576));
#52350=CARTESIAN_POINT('',(430.312474890954,218.5616316647,677.406068680095));
#52351=CARTESIAN_POINT('',(430.312474890954,220.231959303219,675.735741041576));
#52352=CARTESIAN_POINT('Origin',(432.8380463053,221.067123122478,676.570904860836));
#52353=CARTESIAN_POINT('',(430.312474890954,221.902286941738,677.406068680095));
#52354=CARTESIAN_POINT('',(430.312474890954,220.231959303219,675.735741041576));
#52355=CARTESIAN_POINT('',(430.312474890954,221.902286941738,677.406068680095));
#52356=CARTESIAN_POINT('Origin',(432.232023881687,222.261497186581,677.046858435252));
#52357=CARTESIAN_POINT('',(430.312474890954,222.620707431423,676.687648190409));
#52358=CARTESIAN_POINT('',(430.312474890954,221.902286941738,677.406068680095));
#52359=CARTESIAN_POINT('',(430.312474890954,222.620707431423,676.687648190409));
#52360=CARTESIAN_POINT('Origin',(432.8380463053,221.785543612164,675.85248437115));
#52361=CARTESIAN_POINT('',(430.312474890954,220.950379792904,675.017320551891));
#52362=CARTESIAN_POINT('',(430.312474890954,222.620707431423,676.687648190409));
#52363=CARTESIAN_POINT('',(430.312474890954,220.950379792904,675.017320551891));
#52364=CARTESIAN_POINT('Origin',(432.8380463053,221.785543612164,674.182156732631));
#52365=CARTESIAN_POINT('',(430.312474890954,220.950379792904,675.017320551891));
#52366=CARTESIAN_POINT('Origin',(430.312474890954,217.817811175014,675.017320551891));
#52367=CARTESIAN_POINT('Origin',(432.232023881683,276.363497186581,774.333782668528));
#52368=CARTESIAN_POINT('',(430.31247489095,276.722707431424,774.692992913371));
#52369=CARTESIAN_POINT('',(430.31247489095,276.722707431424,774.692992913371));
#52370=CARTESIAN_POINT('',(430.31247489095,276.004286941739,773.974572423685));
#52371=CARTESIAN_POINT('',(430.31247489095,276.722707431424,774.692992913371));
#52372=CARTESIAN_POINT('',(430.31247489095,276.004286941739,773.974572423685));
#52373=CARTESIAN_POINT('Origin',(432.838046305297,275.169123122479,774.809736242944));
#52374=CARTESIAN_POINT('',(430.312474890951,274.33395930322,775.644900062204));
#52375=CARTESIAN_POINT('',(430.31247489095,276.004286941739,773.974572423685));
#52376=CARTESIAN_POINT('',(430.312474890951,274.33395930322,775.644900062204));
#52377=CARTESIAN_POINT('Origin',(432.838046305297,273.49879548396,774.809736242944));
#52378=CARTESIAN_POINT('',(430.312474890951,272.663631664701,773.974572423685));
#52379=CARTESIAN_POINT('',(430.312474890951,274.33395930322,775.644900062204));
#52380=CARTESIAN_POINT('',(430.312474890951,272.663631664701,773.974572423685));
#52381=CARTESIAN_POINT('Origin',(432.232023881684,272.304421419858,774.333782668528));
#52382=CARTESIAN_POINT('',(430.312474890951,271.945211175015,774.692992913371));
#52383=CARTESIAN_POINT('',(430.312474890951,272.663631664701,773.974572423685));
#52384=CARTESIAN_POINT('',(430.312474890951,271.945211175015,774.692992913371));
#52385=CARTESIAN_POINT('Origin',(432.838046305297,272.780374994275,775.528156732631));
#52386=CARTESIAN_POINT('',(430.312474890951,273.615538813534,776.36332055189));
#52387=CARTESIAN_POINT('',(430.312474890951,271.945211175015,774.692992913371));
#52388=CARTESIAN_POINT('',(430.312474890951,273.615538813534,776.36332055189));
#52389=CARTESIAN_POINT('Origin',(432.838046305297,272.780374994275,777.19848437115));
#52390=CARTESIAN_POINT('',(430.312474890951,271.945211175015,778.033648190409));
#52391=CARTESIAN_POINT('',(430.312474890951,273.615538813534,776.36332055189));
#52392=CARTESIAN_POINT('',(430.312474890951,271.945211175015,778.033648190409));
#52393=CARTESIAN_POINT('Origin',(432.232023881684,272.304421419858,778.392858435251));
#52394=CARTESIAN_POINT('',(430.312474890951,272.663631664701,778.752068680094));
#52395=CARTESIAN_POINT('',(430.312474890951,271.945211175015,778.033648190409));
#52396=CARTESIAN_POINT('',(430.312474890951,272.663631664701,778.752068680094));
#52397=CARTESIAN_POINT('Origin',(432.838046305297,273.49879548396,777.916904860835));
#52398=CARTESIAN_POINT('',(430.312474890951,274.33395930322,777.081741041575));
#52399=CARTESIAN_POINT('',(430.312474890951,272.663631664701,778.752068680094));
#52400=CARTESIAN_POINT('',(430.312474890951,274.33395930322,777.081741041575));
#52401=CARTESIAN_POINT('Origin',(432.838046305297,275.169123122479,777.916904860835));
#52402=CARTESIAN_POINT('',(430.31247489095,276.004286941739,778.752068680094));
#52403=CARTESIAN_POINT('',(430.312474890951,274.33395930322,777.081741041575));
#52404=CARTESIAN_POINT('',(430.31247489095,276.004286941739,778.752068680094));
#52405=CARTESIAN_POINT('Origin',(432.232023881683,276.363497186581,778.392858435251));
#52406=CARTESIAN_POINT('',(430.31247489095,276.722707431424,778.033648190409));
#52407=CARTESIAN_POINT('',(430.31247489095,276.004286941739,778.752068680094));
#52408=CARTESIAN_POINT('',(430.31247489095,276.722707431424,778.033648190409));
#52409=CARTESIAN_POINT('Origin',(432.838046305296,275.887543612165,777.19848437115));
#52410=CARTESIAN_POINT('',(430.312474890951,275.052379792905,776.36332055189));
#52411=CARTESIAN_POINT('',(430.31247489095,276.722707431424,778.033648190409));
#52412=CARTESIAN_POINT('',(430.312474890951,275.052379792905,776.36332055189));
#52413=CARTESIAN_POINT('Origin',(432.838046305296,275.887543612165,775.528156732631));
#52414=CARTESIAN_POINT('',(430.312474890951,275.052379792905,776.36332055189));
#52415=CARTESIAN_POINT('Origin',(430.312474890951,271.919811175015,776.36332055189));
#52416=CARTESIAN_POINT('Origin',(374.502534891742,287.021190177127,769.60692055189));
#52417=CARTESIAN_POINT('',(374.764174233796,286.58574918837,763.84112055189));
#52418=CARTESIAN_POINT('',(374.764174233796,286.58574918837,766.20332055189));
#52419=CARTESIAN_POINT('',(374.240895549687,287.456631165884,763.84112055189));
#52420=CARTESIAN_POINT('',(374.764174233796,286.58574918837,763.84112055189));
#52421=CARTESIAN_POINT('',(374.240895549687,287.456631165884,766.20332055189));
#52422=CARTESIAN_POINT('',(374.240895549687,287.456631165884,763.84112055189));
#52423=CARTESIAN_POINT('',(373.024272609134,289.481431763602,766.20332055189));
#52424=CARTESIAN_POINT('',(374.240895549687,287.456631165884,766.20332055189));
#52425=CARTESIAN_POINT('',(373.024272609134,289.481431763602,767.21932055189));
#52426=CARTESIAN_POINT('',(373.024272609134,289.481431763602,766.20332055189));
#52427=CARTESIAN_POINT('',(374.240895549687,287.456631165884,767.21932055189));
#52428=CARTESIAN_POINT('',(373.024272609134,289.481431763602,767.21932055189));
#52429=CARTESIAN_POINT('',(374.240895549687,287.456631165884,769.58152055189));
#52430=CARTESIAN_POINT('',(374.240895549687,287.456631165884,767.21932055189));
#52431=CARTESIAN_POINT('',(374.764174233796,286.58574918837,769.58152055189));
#52432=CARTESIAN_POINT('',(374.240895549687,287.456631165884,769.58152055189));
#52433=CARTESIAN_POINT('',(374.764174233796,286.58574918837,769.58152055189));
#52434=CARTESIAN_POINT('Origin',(375.846032486357,287.235795207705,769.60692055189));
#52435=CARTESIAN_POINT('',(374.764174233796,286.58574918837,769.58152055189));
#52436=CARTESIAN_POINT('Origin',(375.309842945387,286.56034918837,769.58152055189));
#52437=CARTESIAN_POINT('',(374.240895549687,287.456631165884,769.58152055189));
#52438=CARTESIAN_POINT('Origin',(375.322753802249,288.106677185218,769.60692055189));
#52439=CARTESIAN_POINT('',(374.240895549687,287.456631165884,767.21932055189));
#52440=CARTESIAN_POINT('Origin',(374.714442331972,287.431231165884,767.21932055189));
#52441=CARTESIAN_POINT('',(373.024272609134,289.481431763602,767.21932055189));
#52442=CARTESIAN_POINT('Origin',(373.841510050641,289.972477558598,767.24472055189));
#52443=CARTESIAN_POINT('',(373.024272609134,289.481431763602,766.20332055189));
#52444=CARTESIAN_POINT('Origin',(374.714442331972,287.431231165884,766.20332055189));
#52445=CARTESIAN_POINT('',(374.240895549687,287.456631165884,766.20332055189));
#52446=CARTESIAN_POINT('Origin',(375.322753802249,288.106677185218,766.22872055189));
#52447=CARTESIAN_POINT('',(374.240895549687,287.456631165884,763.84112055189));
#52448=CARTESIAN_POINT('Origin',(375.309842945387,286.56034918837,763.84112055189));
#52449=CARTESIAN_POINT('',(374.764174233796,286.58574918837,763.84112055189));
#52450=CARTESIAN_POINT('Origin',(375.846032486357,287.235795207705,766.22872055189));
#52451=CARTESIAN_POINT('Origin',(371.682267445708,285.281359303216,777.88732055189));
#52452=CARTESIAN_POINT('',(372.174522500189,285.281359303216,782.71332055189));
#52453=CARTESIAN_POINT('',(369.479533939566,290.107359303216,777.88732055189));
#52454=CARTESIAN_POINT('Ctrl Pts',(372.174522500189,285.281359303216,782.713320551891));
#52455=CARTESIAN_POINT('Ctrl Pts',(371.855654969792,285.899933374655,782.713320551891));
#52456=CARTESIAN_POINT('Ctrl Pts',(371.504957457388,286.55922733351,782.587944800608));
#52457=CARTESIAN_POINT('Ctrl Pts',(370.836280008275,287.77818982486,782.069981441115));
#52458=CARTESIAN_POINT('Ctrl Pts',(370.518643518802,288.338065228392,781.677437375128));
#52459=CARTESIAN_POINT('Ctrl Pts',(370.038186801395,289.16931580397,780.800937575508));
#52460=CARTESIAN_POINT('Ctrl Pts',(369.832513261077,289.517343365307,780.282107787414));
#52461=CARTESIAN_POINT('Ctrl Pts',(369.552676414556,289.986701593406,779.12761062806));
#52462=CARTESIAN_POINT('Ctrl Pts',(369.479533939566,290.107359303216,778.49142261233));
#52463=CARTESIAN_POINT('Ctrl Pts',(369.479533939566,290.107359303216,777.88732055189));
#52464=CARTESIAN_POINT('',(373.885000951849,285.281359303216,782.71332055189));
#52465=CARTESIAN_POINT('',(369.479533939566,290.107359303216,777.88732055189));
#52466=CARTESIAN_POINT('Origin',(371.278766994166,290.107359303215,732.42132055189));
#52467=CARTESIAN_POINT('',(369.479533939565,290.107359303215,686.95532055189));
#52468=CARTESIAN_POINT('',(369.479533939565,290.107359303215,686.95532055189));
#52469=CARTESIAN_POINT('',(369.479533939566,290.107359303216,777.88732055189));
#52470=CARTESIAN_POINT('Origin',(373.230354482257,288.354759303215,686.95532055189));
#52471=CARTESIAN_POINT('Origin',(298.461074890953,247.282959303211,686.955320551928));
#52472=CARTESIAN_POINT('Origin',(371.342244210912,286.576759303215,682.38332055189));
#52473=CARTESIAN_POINT('Origin',(298.461074890949,247.282959303209,682.383320551846));
#52474=CARTESIAN_POINT('Origin',(371.682267445712,209.284559303215,673.493320551891));
#52475=CARTESIAN_POINT('',(369.479533939571,204.458559303215,673.493320551891));
#52476=CARTESIAN_POINT('',(369.479533939571,204.458559303215,673.493320551891));
#52477=CARTESIAN_POINT('',(372.174522500193,209.284559303215,668.667320551891));
#52478=CARTESIAN_POINT('Ctrl Pts',(372.174522500194,209.284559303215,668.667320551891));
#52479=CARTESIAN_POINT('Ctrl Pts',(371.855654969797,208.665985231775,668.667320551891));
#52480=CARTESIAN_POINT('Ctrl Pts',(371.504957457392,208.00669127292,668.792696303173));
#52481=CARTESIAN_POINT('Ctrl Pts',(370.83628000828,206.78772878157,669.310659662666));
#52482=CARTESIAN_POINT('Ctrl Pts',(370.518643518807,206.227853378039,669.703203728653));
#52483=CARTESIAN_POINT('Ctrl Pts',(370.0381868014,205.39660280246,670.579703528274));
#52484=CARTESIAN_POINT('Ctrl Pts',(369.832513261083,205.048575241123,671.098533316367));
#52485=CARTESIAN_POINT('Ctrl Pts',(369.552676414562,204.579217013024,672.253030475721));
#52486=CARTESIAN_POINT('Ctrl Pts',(369.479533939571,204.458559303215,672.889218491451));
#52487=CARTESIAN_POINT('Ctrl Pts',(369.479533939571,204.458559303215,673.493320551891));
#52488=CARTESIAN_POINT('',(373.885000951854,209.284559303215,668.667320551891));
#52489=CARTESIAN_POINT('Origin',(399.770298695574,209.259159303217,668.667320551891));
#52490=CARTESIAN_POINT('',(376.030529085239,280.683959303215,668.66732055189));
#52491=CARTESIAN_POINT('',(427.366074890954,213.881959303219,668.667320551891));
#52492=CARTESIAN_POINT('Origin',(298.461074890952,247.28295930321,668.66732055189));
#52493=CARTESIAN_POINT('Origin',(399.770298695574,209.259159303218,782.713320551891));
#52494=CARTESIAN_POINT('Origin',(298.461074890953,247.282959303211,782.713320551891));
#52495=CARTESIAN_POINT('',(427.366074890955,213.88195930322,782.713320551891));
#52496=CARTESIAN_POINT('',(376.03052908524,280.683959303216,782.713320551891));
#52497=CARTESIAN_POINT('Origin',(371.342244210917,204.433159303215,686.955320551891));
#52498=CARTESIAN_POINT('Origin',(298.461074890911,247.282959303233,686.955320551891));
#52499=CARTESIAN_POINT('Origin',(371.342244210917,204.433159303215,682.383320551891));
#52500=CARTESIAN_POINT('',(369.479533939571,204.458559303215,682.383320551891));
#52501=CARTESIAN_POINT('Origin',(298.461074890906,247.282959303239,682.383320551943));
#52502=CARTESIAN_POINT('',(369.479533939571,204.458559303215,682.383320551891));
#52503=CARTESIAN_POINT('Origin',(371.278766994171,204.458559303215,677.938320551891));
#52504=CARTESIAN_POINT('',(369.479533939572,204.458559303215,673.493320551891));
#52505=CARTESIAN_POINT('Origin',(427.391474890954,213.881959303219,725.690320551891));
#52506=CARTESIAN_POINT('',(405.141074890954,213.881959303218,736.86632055189));
#52507=CARTESIAN_POINT('Origin',(405.141074890955,213.881959303218,725.690320551891));
#52508=CARTESIAN_POINT('Origin',(427.39147489095,280.683959303219,725.69032055189));
#52509=CARTESIAN_POINT('Origin',(375.3121954222,206.465585535989,725.207720551891));
#52510=CARTESIAN_POINT('',(374.240895549693,207.109287440548,722.820120551891));
#52511=CARTESIAN_POINT('',(374.240895549693,207.109287440548,722.820120551891));
#52512=CARTESIAN_POINT('',(374.240895549692,207.109287440548,725.182320551891));
#52513=CARTESIAN_POINT('',(374.240895549692,207.109287440548,725.182320551891));
#52514=CARTESIAN_POINT('',(374.240895549692,207.109287440548,725.182320551891));
#52515=CARTESIAN_POINT('Origin',(374.703883951924,204.111811032767,725.182320551891));
#52516=CARTESIAN_POINT('',(373.02427260914,205.084486842829,725.182320551891));
#52517=CARTESIAN_POINT('',(373.02427260914,205.084486842829,725.182320551891));
#52518=CARTESIAN_POINT('',(373.02427260914,205.084486842829,725.182320551891));
#52519=CARTESIAN_POINT('Origin',(375.290800739153,206.136611630486,722.820120551891));
#52520=CARTESIAN_POINT('',(374.764174233801,207.980169418061,722.820120551891));
#52521=CARTESIAN_POINT('',(374.764174233801,207.980169418061,722.820120551891));
#52522=CARTESIAN_POINT('',(374.240895549693,207.109287440548,722.820120551891));
#52523=CARTESIAN_POINT('Origin',(373.82220154347,204.605042769408,726.223720551891));
#52524=CARTESIAN_POINT('',(373.02427260914,205.084486842829,726.198320551891));
#52525=CARTESIAN_POINT('',(373.02427260914,205.084486842829,726.198320551891));
#52526=CARTESIAN_POINT('',(373.02427260914,205.084486842829,726.198320551891));
#52527=CARTESIAN_POINT('Origin',(376.408895294708,205.623249236658,726.198320551891));
#52528=CARTESIAN_POINT('',(374.240895549692,207.109287440548,726.198320551891));
#52529=CARTESIAN_POINT('',(374.240895549692,207.109287440548,726.198320551891));
#52530=CARTESIAN_POINT('',(374.240895549692,207.109287440548,726.198320551891));
#52531=CARTESIAN_POINT('Origin',(375.3121954222,206.465585535989,728.585920551891));
#52532=CARTESIAN_POINT('',(374.240895549693,207.109287440548,728.560520551891));
#52533=CARTESIAN_POINT('',(374.240895549693,207.109287440548,728.560520551891));
#52534=CARTESIAN_POINT('',(374.240895549693,207.109287440548,728.560520551891));
#52535=CARTESIAN_POINT('Origin',(375.290800739153,206.136611630486,728.560520551891));
#52536=CARTESIAN_POINT('',(374.764174233801,207.980169418061,728.560520551891));
#52537=CARTESIAN_POINT('',(374.764174233801,207.980169418061,728.560520551891));
#52538=CARTESIAN_POINT('',(374.764174233801,207.980169418061,728.560520551891));
#52539=CARTESIAN_POINT('Origin',(375.835474106309,207.336467513502,728.585920551891));
#52540=CARTESIAN_POINT('',(374.764174233801,207.980169418061,726.198320551891));
#52541=CARTESIAN_POINT('',(374.764174233801,207.980169418061,726.198320551891));
#52542=CARTESIAN_POINT('',(374.764174233801,207.980169418061,726.198320551891));
#52543=CARTESIAN_POINT('Origin',(376.160751551484,206.667365608943,726.198320551891));
#52544=CARTESIAN_POINT('',(375.980797174353,210.00497001578,726.198320551891));
#52545=CARTESIAN_POINT('',(375.980797174353,210.00497001578,726.198320551891));
#52546=CARTESIAN_POINT('',(375.980797174353,210.00497001578,726.198320551891));
#52547=CARTESIAN_POINT('Origin',(376.788427340408,209.519696854259,726.223720551891));
#52548=CARTESIAN_POINT('',(375.980797174353,210.00497001578,725.182320551891));
#52549=CARTESIAN_POINT('',(375.980797174353,210.00497001578,725.182320551891));
#52550=CARTESIAN_POINT('',(375.980797174353,210.00497001578,725.182320551891));
#52551=CARTESIAN_POINT('Origin',(377.582728869166,208.348867812361,725.182320551891));
#52552=CARTESIAN_POINT('',(374.764174233801,207.980169418061,725.182320551891));
#52553=CARTESIAN_POINT('',(374.764174233801,207.980169418061,725.182320551891));
#52554=CARTESIAN_POINT('',(374.764174233801,207.980169418061,725.182320551891));
#52555=CARTESIAN_POINT('Origin',(405.141074890954,216.421959303218,725.69032055189));
#52556=CARTESIAN_POINT('',(405.141074890954,218.961959303218,736.86632055189));
#52557=CARTESIAN_POINT('',(405.141074890954,216.421959303218,736.86632055189));
#52558=CARTESIAN_POINT('Origin',(405.141074890954,218.961959303218,725.690320551891));
#52559=CARTESIAN_POINT('Origin',(416.342474890954,218.961959303218,725.690320551891));
#52560=CARTESIAN_POINT('Origin',(374.502534891747,207.544728429304,728.585920551891));
#52561=CARTESIAN_POINT('',(374.764174233801,207.980169418061,722.820120551891));
#52562=CARTESIAN_POINT('Origin',(375.835474106309,207.336467513502,725.207720551891));
#52563=CARTESIAN_POINT('Origin',(371.183235802879,285.026754071854,725.69032055189));
#52564=CARTESIAN_POINT('',(376.340705928608,287.533024998432,728.56052055189));
#52565=CARTESIAN_POINT('Origin',(371.444875144932,284.591313083098,725.69032055189));
#52566=CARTESIAN_POINT('',(375.8174272445,288.403906975945,728.56052055189));
#52567=CARTESIAN_POINT('Origin',(371.183235802879,285.026754071854,728.560520551888));
#52568=CARTESIAN_POINT('',(376.383495294702,288.744034975002,726.19832055189));
#52569=CARTESIAN_POINT('Origin',(370.921596460824,285.46219506061,725.69032055189));
#52570=CARTESIAN_POINT('',(374.600804303947,290.428707573663,726.19832055189));
#52571=CARTESIAN_POINT('Origin',(371.183235802879,285.026754071854,726.198320551891));
#52572=CARTESIAN_POINT('',(374.600804303947,290.428707573663,725.18232055189));
#52573=CARTESIAN_POINT('Origin',(369.704973520274,287.486995658328,725.69032055189));
#52574=CARTESIAN_POINT('',(376.383495294702,288.744034975002,725.18232055189));
#52575=CARTESIAN_POINT('Origin',(371.183235802879,285.026754071854,725.18232055189));
#52576=CARTESIAN_POINT('',(375.8174272445,288.403906975945,722.82012055189));
#52577=CARTESIAN_POINT('Origin',(370.921596460822,285.462195060611,725.690320551891));
#52578=CARTESIAN_POINT('',(376.340705928608,287.533024998432,722.82012055189));
#52579=CARTESIAN_POINT('Origin',(371.183235802883,285.026754071857,722.820120551892));
#52580=CARTESIAN_POINT('',(376.906773978811,287.873152997488,725.18232055189));
#52581=CARTESIAN_POINT('Origin',(371.444875144934,284.591313083099,725.69032055189));
#52582=CARTESIAN_POINT('Origin',(371.183235802878,285.026754071854,725.18232055189));
#52583=CARTESIAN_POINT('Origin',(374.502534891741,287.021190177127,728.58592055189));
#52584=CARTESIAN_POINT('',(374.764174233796,286.58574918837,725.18232055189));
#52585=CARTESIAN_POINT('',(375.980797174348,284.560948590652,725.18232055189));
#52586=CARTESIAN_POINT('',(374.764174233796,286.58574918837,722.82012055189));
#52587=CARTESIAN_POINT('',(374.764174233796,286.58574918837,725.18232055189));
#52588=CARTESIAN_POINT('',(374.240895549687,287.456631165883,722.82012055189));
#52589=CARTESIAN_POINT('',(374.764174233796,286.58574918837,722.82012055189));
#52590=CARTESIAN_POINT('',(374.240895549687,287.456631165883,725.18232055189));
#52591=CARTESIAN_POINT('',(374.240895549687,287.456631165883,722.82012055189));
#52592=CARTESIAN_POINT('',(373.024272609134,289.481431763602,725.18232055189));
#52593=CARTESIAN_POINT('',(374.240895549687,287.456631165883,725.18232055189));
#52594=CARTESIAN_POINT('',(373.024272609134,289.481431763602,726.19832055189));
#52595=CARTESIAN_POINT('',(373.024272609134,289.481431763602,725.18232055189));
#52596=CARTESIAN_POINT('',(374.240895549687,287.456631165883,726.19832055189));
#52597=CARTESIAN_POINT('',(373.024272609134,289.481431763602,726.19832055189));
#52598=CARTESIAN_POINT('',(374.240895549687,287.456631165883,728.56052055189));
#52599=CARTESIAN_POINT('',(374.240895549687,287.456631165883,726.19832055189));
#52600=CARTESIAN_POINT('',(374.764174233796,286.58574918837,728.56052055189));
#52601=CARTESIAN_POINT('',(374.240895549687,287.456631165883,728.56052055189));
#52602=CARTESIAN_POINT('',(374.764174233796,286.58574918837,728.56052055189));
#52603=CARTESIAN_POINT('Origin',(375.835474106303,287.229451092929,728.58592055189));
#52604=CARTESIAN_POINT('',(374.764174233796,286.58574918837,728.56052055189));
#52605=CARTESIAN_POINT('Origin',(375.290800739148,286.56034918837,728.56052055189));
#52606=CARTESIAN_POINT('',(374.240895549687,287.456631165883,728.56052055189));
#52607=CARTESIAN_POINT('Origin',(375.312195422195,288.100333070442,728.58592055189));
#52608=CARTESIAN_POINT('',(374.240895549687,287.456631165883,726.19832055189));
#52609=CARTESIAN_POINT('Origin',(374.703883951918,287.431231165883,726.19832055189));
#52610=CARTESIAN_POINT('',(373.024272609134,289.481431763602,726.19832055189));
#52611=CARTESIAN_POINT('Origin',(373.831902775189,289.966704925123,726.22372055189));
#52612=CARTESIAN_POINT('',(373.024272609134,289.481431763602,725.18232055189));
#52613=CARTESIAN_POINT('Origin',(376.408895294702,288.942669369774,725.18232055189));
#52614=CARTESIAN_POINT('',(374.240895549687,287.456631165883,725.18232055189));
#52615=CARTESIAN_POINT('Origin',(375.312195422195,288.100333070442,725.20772055189));
#52616=CARTESIAN_POINT('',(374.240895549687,287.456631165883,722.82012055189));
#52617=CARTESIAN_POINT('Origin',(375.290800739148,286.56034918837,722.82012055189));
#52618=CARTESIAN_POINT('',(374.764174233796,286.58574918837,722.82012055189));
#52619=CARTESIAN_POINT('Origin',(375.835474106303,287.229451092929,725.20772055189));
#52620=CARTESIAN_POINT('',(374.764174233796,286.58574918837,725.18232055189));
#52621=CARTESIAN_POINT('Origin',(376.160751551479,284.535548590652,725.18232055189));
#52622=CARTESIAN_POINT('Origin',(298.461074890946,338.240359303211,792.23832055189));
#52623=CARTESIAN_POINT('',(389.393074890952,247.282959303217,792.238320551891));
#52624=CARTESIAN_POINT('Origin',(298.461074890952,247.282959303211,792.238320551891));
#52625=CARTESIAN_POINT('',(215.530074890953,247.282959303205,792.238320551891));
#52626=CARTESIAN_POINT('Origin',(298.461074890953,247.282959303211,792.238320551891));
#52627=CARTESIAN_POINT('Origin',(224.281150396699,301.177829172505,810.450120551891));
#52628=CARTESIAN_POINT('',(222.545282322562,297.337140574242,810.450120551891));
#52629=CARTESIAN_POINT('',(227.397449580236,304.015575862807,810.450120551891));
#52630=CARTESIAN_POINT('Ctrl Pts',(222.545282322562,297.337140574242,810.450120551891));
#52631=CARTESIAN_POINT('Ctrl Pts',(222.545282322562,297.337140574242,810.968455084256));
#52632=CARTESIAN_POINT('Ctrl Pts',(222.602220666962,297.42383385282,811.521290446934));
#52633=CARTESIAN_POINT('Ctrl Pts',(222.83552034229,297.775023669248,812.538200080674));
#52634=CARTESIAN_POINT('Ctrl Pts',(223.01208514873,298.039367523769,813.002280383611));
#52635=CARTESIAN_POINT('Ctrl Pts',(223.423802412012,298.646085838271,813.735127146313));
#52636=CARTESIAN_POINT('Ctrl Pts',(223.686446736859,299.028898397941,814.052768044994));
#52637=CARTESIAN_POINT('Ctrl Pts',(224.269877629636,299.861980569393,814.474016718618));
#52638=CARTESIAN_POINT('Ctrl Pts',(224.590872208263,300.312106479352,814.577620551891));
#52639=CARTESIAN_POINT('Ctrl Pts',(225.200210908629,301.150789249978,814.577620551891));
#52640=CARTESIAN_POINT('Ctrl Pts',(225.52911330855,301.595169791463,814.474016718618));
#52641=CARTESIAN_POINT('Ctrl Pts',(226.141131475408,302.407482092536,814.052768044994));
#52642=CARTESIAN_POINT('Ctrl Pts',(226.424046294948,302.775567275748,813.735127146313));
#52643=CARTESIAN_POINT('Ctrl Pts',(226.873842070279,303.354619931843,813.002280383611));
#52644=CARTESIAN_POINT('Ctrl Pts',(227.070686489865,303.604229784962,812.538200080674));
#52645=CARTESIAN_POINT('Ctrl Pts',(227.332594288776,303.93463458296,811.521290446934));
#52646=CARTESIAN_POINT('Ctrl Pts',(227.397449580236,304.015575862807,810.968455084256));
#52647=CARTESIAN_POINT('Ctrl Pts',(227.397449580236,304.015575862807,810.450120551891));
#52648=CARTESIAN_POINT('',(226.017018470835,305.018517770768,810.450120551891));
#52649=CARTESIAN_POINT('',(226.707234025536,304.517046816788,810.450120551891));
#52650=CARTESIAN_POINT('',(223.590934913942,301.679300225506,806.322620551891));
#52651=CARTESIAN_POINT('Origin',(223.590934841999,301.679300126486,810.450120551891));
#52652=CARTESIAN_POINT('Origin',(223.590934841999,301.679300126486,810.450120551891));
#52653=CARTESIAN_POINT('Ctrl Pts',(227.397449580236,304.015575862807,810.450120551891));
#52654=CARTESIAN_POINT('Ctrl Pts',(227.397449580236,304.015575862807,809.931786019525));
#52655=CARTESIAN_POINT('Ctrl Pts',(227.332594288776,303.93463458296,809.378950656848));
#52656=CARTESIAN_POINT('Ctrl Pts',(227.070686489865,303.604229784962,808.362041023107));
#52657=CARTESIAN_POINT('Ctrl Pts',(226.873842070279,303.354619931843,807.89796072017));
#52658=CARTESIAN_POINT('Ctrl Pts',(226.424046294948,302.775567275748,807.165113957469));
#52659=CARTESIAN_POINT('Ctrl Pts',(226.141131475408,302.407482092536,806.847473058788));
#52660=CARTESIAN_POINT('Ctrl Pts',(225.52911330855,301.595169791463,806.426224385163));
#52661=CARTESIAN_POINT('Ctrl Pts',(225.200210908628,301.150789249978,806.322620551891));
#52662=CARTESIAN_POINT('Ctrl Pts',(224.590872208263,300.312106479352,806.322620551891));
#52663=CARTESIAN_POINT('Ctrl Pts',(224.269877629636,299.861980569393,806.426224385163));
#52664=CARTESIAN_POINT('Ctrl Pts',(223.686446736859,299.028898397941,806.847473058788));
#52665=CARTESIAN_POINT('Ctrl Pts',(223.423802412012,298.646085838271,807.165113957469));
#52666=CARTESIAN_POINT('Ctrl Pts',(223.01208514873,298.039367523769,807.89796072017));
#52667=CARTESIAN_POINT('Ctrl Pts',(222.83552034229,297.775023669248,808.362041023107));
#52668=CARTESIAN_POINT('Ctrl Pts',(222.602220666962,297.42383385282,809.378950656848));
#52669=CARTESIAN_POINT('Ctrl Pts',(222.545282322562,297.337140574242,809.931786019525));
#52670=CARTESIAN_POINT('Ctrl Pts',(222.545282322562,297.337140574242,810.450120551891));
#52671=CARTESIAN_POINT('Origin',(298.461074890959,153.429959303211,810.460151039948));
#52672=CARTESIAN_POINT('',(298.469433631005,153.429959303211,810.450120551892));
#52673=CARTESIAN_POINT('',(298.461074893041,153.429959303211,810.458479291938));
#52674=CARTESIAN_POINT('Origin',(298.461074890959,153.429959303211,810.450120551892));
#52675=CARTESIAN_POINT('Origin',(298.461074890959,153.429959303211,810.450120551892));
#52676=CARTESIAN_POINT('Origin',(298.461074890958,155.591530062517,810.450120551892));
#52677=CARTESIAN_POINT('',(302.588574890958,156.444683407254,810.450120551892));
#52678=CARTESIAN_POINT('',(294.333574890958,156.444683407254,810.450120551892));
#52679=CARTESIAN_POINT('Ctrl Pts',(302.588574890958,156.444683407255,810.450120551892));
#52680=CARTESIAN_POINT('Ctrl Pts',(302.588574890958,156.444683407255,810.968455084257));
#52681=CARTESIAN_POINT('Ctrl Pts',(302.484971036162,156.439790464884,811.521290446935));
#52682=CARTESIAN_POINT('Ctrl Pts',(302.063722397899,156.422109672155,812.538200080675));
#52683=CARTESIAN_POINT('Ctrl Pts',(301.746081537933,156.409576181953,813.002280383612));
#52684=CARTESIAN_POINT('Ctrl Pts',(301.013234775231,156.386042367265,813.735127146314));
#52685=CARTESIAN_POINT('Ctrl Pts',(300.549154448054,156.373514512576,814.052768044995));
#52686=CARTESIAN_POINT('Ctrl Pts',(299.532244739133,156.355846605548,814.474016718619));
#52687=CARTESIAN_POINT('Ctrl Pts',(298.979409348984,156.350959303211,814.577620551892));
#52688=CARTESIAN_POINT('Ctrl Pts',(297.942740432933,156.350959303211,814.577620551892));
#52689=CARTESIAN_POINT('Ctrl Pts',(297.389905042784,156.355846605548,814.474016718619));
#52690=CARTESIAN_POINT('Ctrl Pts',(296.372995333862,156.373514512576,814.052768044995));
#52691=CARTESIAN_POINT('Ctrl Pts',(295.908915006686,156.386042367265,813.735127146314));
#52692=CARTESIAN_POINT('Ctrl Pts',(295.176068243984,156.409576181952,813.002280383612));
#52693=CARTESIAN_POINT('Ctrl Pts',(294.858427384018,156.422109672155,812.538200080675));
#52694=CARTESIAN_POINT('Ctrl Pts',(294.437178745755,156.439790464884,811.521290446935));
#52695=CARTESIAN_POINT('Ctrl Pts',(294.333574890958,156.444683407254,810.968455084257));
#52696=CARTESIAN_POINT('Ctrl Pts',(294.333574890958,156.444683407254,810.450120551892));
#52697=CARTESIAN_POINT('',(294.333574890958,154.738376717779,810.450120550069));
#52698=CARTESIAN_POINT('',(294.333574890958,155.591530062517,810.450120551892));
#52699=CARTESIAN_POINT('',(298.46107489266,154.73837671778,814.577620551892));
#52700=CARTESIAN_POINT('Origin',(298.461074890958,154.73837671778,810.450120551892));
#52701=CARTESIAN_POINT('Origin',(298.461074890958,154.73837671778,810.450120551892));
#52702=CARTESIAN_POINT('Ctrl Pts',(294.333574890958,156.444683407254,810.450120551892));
#52703=CARTESIAN_POINT('Ctrl Pts',(294.333574890958,156.444683407254,809.931786019526));
#52704=CARTESIAN_POINT('Ctrl Pts',(294.437178745755,156.439790464884,809.378950656849));
#52705=CARTESIAN_POINT('Ctrl Pts',(294.858427384018,156.422109672155,808.362041023108));
#52706=CARTESIAN_POINT('Ctrl Pts',(295.176068243984,156.409576181952,807.897960720171));
#52707=CARTESIAN_POINT('Ctrl Pts',(295.908915006686,156.386042367265,807.16511395747));
#52708=CARTESIAN_POINT('Ctrl Pts',(296.372995333862,156.373514512576,806.847473058789));
#52709=CARTESIAN_POINT('Ctrl Pts',(297.389905042784,156.355846605548,806.426224385164));
#52710=CARTESIAN_POINT('Ctrl Pts',(297.942740432933,156.350959303211,806.322620551892));
#52711=CARTESIAN_POINT('Ctrl Pts',(298.979409348984,156.350959303211,806.322620551892));
#52712=CARTESIAN_POINT('Ctrl Pts',(299.532244739133,156.355846605548,806.426224385164));
#52713=CARTESIAN_POINT('Ctrl Pts',(300.549154448054,156.373514512576,806.847473058789));
#52714=CARTESIAN_POINT('Ctrl Pts',(301.013234775231,156.386042367265,807.165113957469));
#52715=CARTESIAN_POINT('Ctrl Pts',(301.746081537933,156.409576181953,807.897960720171));
#52716=CARTESIAN_POINT('Ctrl Pts',(302.063722397899,156.422109672155,808.362041023108));
#52717=CARTESIAN_POINT('Ctrl Pts',(302.484971036162,156.439790464884,809.378950656849));
#52718=CARTESIAN_POINT('Ctrl Pts',(302.588574890958,156.444683407255,809.931786019526));
#52719=CARTESIAN_POINT('Ctrl Pts',(302.588574890958,156.444683407255,810.450120551892));
#52720=CARTESIAN_POINT('Origin',(379.74015711233,294.209459303217,810.460151039946));
#52721=CARTESIAN_POINT('',(379.735977742307,294.21669818444,810.45012055189));
#52722=CARTESIAN_POINT('',(379.744336482353,294.202220421994,810.450120664857));
#52723=CARTESIAN_POINT('Origin',(379.74015711233,294.209459303217,810.45012055189));
#52724=CARTESIAN_POINT('',(379.740157117303,294.209459294603,810.458479291936));
#52725=CARTESIAN_POINT('Ctrl Pts',(379.740157117303,294.209459294603,810.458479291936));
#52726=CARTESIAN_POINT('Ctrl Pts',(379.738425964101,294.212457739905,810.458479296056));
#52727=CARTESIAN_POINT('Ctrl Pts',(379.737201853204,294.214577962173,810.456031077176));
#52728=CARTESIAN_POINT('Ctrl Pts',(379.735977742307,294.21669818444,810.453582858295));
#52729=CARTESIAN_POINT('Ctrl Pts',(379.735977742307,294.21669818444,810.45012055189));
#52730=CARTESIAN_POINT('Origin',(379.74015711233,294.209459303217,810.45012055189));
#52731=CARTESIAN_POINT('Origin',(377.868181922694,293.128673923564,810.45012055189));
#52732=CARTESIAN_POINT('',(375.065579452827,296.276617105315,810.45012055189));
#52733=CARTESIAN_POINT('',(379.193079452828,289.127577397075,810.45012055189));
#52734=CARTESIAN_POINT('Ctrl Pts',(375.065579452827,296.276617105315,810.45012055189));
#52735=CARTESIAN_POINT('Ctrl Pts',(375.065579452827,296.276617105315,810.968455084256));
#52736=CARTESIAN_POINT('Ctrl Pts',(375.121618792617,296.189340006316,811.521290446933));
#52737=CARTESIAN_POINT('Ctrl Pts',(375.347555127411,295.833368380635,812.538200080674));
#52738=CARTESIAN_POINT('Ctrl Pts',(375.517229878308,295.564550071726,813.002280383611));
#52739=CARTESIAN_POINT('Ctrl Pts',(375.904034141026,294.941653065489,813.735127146312));
#52740=CARTESIAN_POINT('Ctrl Pts',(376.14692374503,294.546011640102,814.052768044993));
#52741=CARTESIAN_POINT('Ctrl Pts',(376.670679455809,293.674175952335,814.474016718618));
#52742=CARTESIAN_POINT('Ctrl Pts',(376.951329678863,293.197850111524,814.57762055189));
#52743=CARTESIAN_POINT('Ctrl Pts',(377.469664136889,292.300068494909,814.57762055189));
#52744=CARTESIAN_POINT('Ctrl Pts',(377.741849303983,291.818855351761,814.474016718618));
#52745=CARTESIAN_POINT('Ctrl Pts',(378.235003302126,290.929351756966,814.052768044993));
#52746=CARTESIAN_POINT('Ctrl Pts',(378.456194025299,290.52118247689,813.735127146313));
#52747=CARTESIAN_POINT('Ctrl Pts',(378.802236525283,289.874751655965,813.002280383611));
#52748=CARTESIAN_POINT('Ctrl Pts',(378.950202634352,289.593399856854,812.538200080674));
#52749=CARTESIAN_POINT('Ctrl Pts',(379.145514937821,289.219747438444,811.521290446933));
#52750=CARTESIAN_POINT('Ctrl Pts',(379.193079452828,289.127577397075,810.968455084256));
#52751=CARTESIAN_POINT('Ctrl Pts',(379.193079452828,289.127577397075,810.45012055189));
#52752=CARTESIAN_POINT('',(380.67078439256,289.980730741812,810.45012055189));
#52753=CARTESIAN_POINT('',(379.931931922694,289.554154069444,810.45012055189));
#52754=CARTESIAN_POINT('Origin',(378.60703439256,293.555250595932,810.45012055189));
#52755=CARTESIAN_POINT('Ctrl Pts',(379.193079452828,289.127577397075,810.45012055189));
#52756=CARTESIAN_POINT('Ctrl Pts',(379.193079452828,289.127577397075,809.931786019525));
#52757=CARTESIAN_POINT('Ctrl Pts',(379.145514937821,289.219747438444,809.378950656847));
#52758=CARTESIAN_POINT('Ctrl Pts',(378.950202634352,289.593399856854,808.362041023107));
#52759=CARTESIAN_POINT('Ctrl Pts',(378.802236525283,289.874751655965,807.89796072017));
#52760=CARTESIAN_POINT('Ctrl Pts',(378.456194025299,290.52118247689,807.165113957468));
#52761=CARTESIAN_POINT('Ctrl Pts',(378.235003302126,290.929351756966,806.847473058788));
#52762=CARTESIAN_POINT('Ctrl Pts',(377.741849303983,291.818855351761,806.426224385163));
#52763=CARTESIAN_POINT('Ctrl Pts',(377.469664136889,292.300068494909,806.32262055189));
#52764=CARTESIAN_POINT('Ctrl Pts',(376.951329678863,293.197850111524,806.32262055189));
#52765=CARTESIAN_POINT('Ctrl Pts',(376.670679455809,293.674175952335,806.426224385163));
#52766=CARTESIAN_POINT('Ctrl Pts',(376.14692374503,294.546011640102,806.847473058788));
#52767=CARTESIAN_POINT('Ctrl Pts',(375.904034141026,294.941653065489,807.165113957468));
#52768=CARTESIAN_POINT('Ctrl Pts',(375.517229878308,295.564550071726,807.89796072017));
#52769=CARTESIAN_POINT('Ctrl Pts',(375.347555127411,295.833368380635,808.362041023107));
#52770=CARTESIAN_POINT('Ctrl Pts',(375.121618792617,296.189340006316,809.378950656847));
#52771=CARTESIAN_POINT('Ctrl Pts',(375.065579452827,296.276617105315,809.931786019525));
#52772=CARTESIAN_POINT('Ctrl Pts',(375.065579452827,296.276617105315,810.45012055189));
#52773=CARTESIAN_POINT('Ctrl Pts',(379.744340671372,294.202222954448,810.450120664856));
#52774=CARTESIAN_POINT('Ctrl Pts',(379.744340671258,294.202222954382,810.458479276214));
#52775=CARTESIAN_POINT('Ctrl Pts',(379.740161365609,294.209461724175,810.458479276214));
#52776=CARTESIAN_POINT('Ctrl Pts',(379.735982059961,294.216700493969,810.458479276214));
#52777=CARTESIAN_POINT('Ctrl Pts',(379.735982060075,294.216700494035,810.450120664856));
#52778=CARTESIAN_POINT('Ctrl Pts',(379.735982060189,294.216700494101,810.441762053498));
#52779=CARTESIAN_POINT('Ctrl Pts',(379.740161365838,294.209461724307,810.441762053498));
#52780=CARTESIAN_POINT('Ctrl Pts',(379.744340671486,294.202222954514,810.441762053498));
#52781=CARTESIAN_POINT('Ctrl Pts',(379.744340671372,294.202222954448,810.450120664856));
#52782=CARTESIAN_POINT('Ctrl Pts',(380.878029350219,292.238616625522,810.450120664856));
#52783=CARTESIAN_POINT('Ctrl Pts',(380.87802931912,292.238616607567,812.725856579518));
#52784=CARTESIAN_POINT('Ctrl Pts',(379.740161370053,294.209461726741,812.725856579518));
#52785=CARTESIAN_POINT('Ctrl Pts',(378.602293420985,296.180306845914,812.725856579518));
#52786=CARTESIAN_POINT('Ctrl Pts',(378.602293452084,296.180306863869,810.450120664856));
#52787=CARTESIAN_POINT('Ctrl Pts',(378.602293483183,296.180306881824,808.174384750194));
#52788=CARTESIAN_POINT('Ctrl Pts',(379.74016143225,294.20946176265,808.174384750194));
#52789=CARTESIAN_POINT('Ctrl Pts',(380.878029381317,292.238616643477,808.174384750194));
#52790=CARTESIAN_POINT('Ctrl Pts',(380.878029350219,292.238616625522,810.450120664856));
#52791=CARTESIAN_POINT('Ctrl Pts',(380.670784378444,289.980730588271,810.45012064421));
#52792=CARTESIAN_POINT('Ctrl Pts',(380.670784322041,289.980730555706,814.577620745582));
#52793=CARTESIAN_POINT('Ctrl Pts',(378.607034286343,293.55525050627,814.577620745582));
#52794=CARTESIAN_POINT('Ctrl Pts',(376.543284250646,297.129770456834,814.577620745582));
#52795=CARTESIAN_POINT('Ctrl Pts',(376.54328430705,297.129770489399,810.45012064421));
#52796=CARTESIAN_POINT('Ctrl Pts',(376.543284363453,297.129770521964,806.322620542838));
#52797=CARTESIAN_POINT('Ctrl Pts',(378.607034399151,293.5552505714,806.322620542838));
#52798=CARTESIAN_POINT('Ctrl Pts',(380.670784434848,289.980730620835,806.322620542838));
#52799=CARTESIAN_POINT('Ctrl Pts',(380.670784378444,289.980730588271,810.45012064421));
#52800=CARTESIAN_POINT('Origin',(373.56256640991,290.633173806373,810.450120552221));
#52801=CARTESIAN_POINT('Origin',(222.532402917877,302.448368586612,810.460151039947));
#52802=CARTESIAN_POINT('',(222.527485814252,302.441609100606,810.450120551891));
#52803=CARTESIAN_POINT('',(222.532399041916,302.448371578067,810.441761677343));
#52804=CARTESIAN_POINT('Origin',(222.532399042082,302.44837157828,810.450120559565));
#52805=CARTESIAN_POINT('Origin',(222.532399042082,302.44837157828,810.450120559565));
#52806=CARTESIAN_POINT('Ctrl Pts',(222.532399041916,302.448371578067,810.441761677343));
#52807=CARTESIAN_POINT('Ctrl Pts',(222.537312269244,302.455134055051,810.441761677354));
#52808=CARTESIAN_POINT('Ctrl Pts',(222.537312269244,302.455134055037,810.450120558723));
#52809=CARTESIAN_POINT('Ctrl Pts',(222.537312269244,302.455134055024,810.458479440092));
#52810=CARTESIAN_POINT('Ctrl Pts',(222.532399041916,302.44837157804,810.458479440081));
#52811=CARTESIAN_POINT('Ctrl Pts',(222.527485814588,302.441609101056,810.45847944007));
#52812=CARTESIAN_POINT('Ctrl Pts',(222.527485814588,302.44160910107,810.450120558701));
#52813=CARTESIAN_POINT('Ctrl Pts',(222.527485814588,302.441609101083,810.441761677332));
#52814=CARTESIAN_POINT('Ctrl Pts',(222.532399041916,302.448371578067,810.441761677343));
#52815=CARTESIAN_POINT('Ctrl Pts',(222.532399078261,302.448371555347,808.17438450705));
#52816=CARTESIAN_POINT('Ctrl Pts',(223.870043204029,304.289480669341,808.174384510044));
#52817=CARTESIAN_POINT('Ctrl Pts',(223.870043204029,304.289480665641,810.450120561705));
#52818=CARTESIAN_POINT('Ctrl Pts',(223.870043204029,304.289480661941,812.725856613366));
#52819=CARTESIAN_POINT('Ctrl Pts',(222.532399078261,302.448371547948,812.725856610373));
#52820=CARTESIAN_POINT('Ctrl Pts',(221.194754952494,300.607262433954,812.72585660738));
#52821=CARTESIAN_POINT('Ctrl Pts',(221.194754952494,300.607262437653,810.450120555719));
#52822=CARTESIAN_POINT('Ctrl Pts',(221.194754952494,300.607262441353,808.174384504057));
#52823=CARTESIAN_POINT('Ctrl Pts',(222.532399078261,302.448371555347,808.17438450705));
#52824=CARTESIAN_POINT('Ctrl Pts',(223.59093498133,301.679300175303,806.322620432803));
#52825=CARTESIAN_POINT('Ctrl Pts',(226.017018749623,305.018517872351,806.322620438231));
#52826=CARTESIAN_POINT('Ctrl Pts',(226.017018749623,305.018517865641,810.45012056289));
#52827=CARTESIAN_POINT('Ctrl Pts',(226.017018749623,305.018517858931,814.577620687549));
#52828=CARTESIAN_POINT('Ctrl Pts',(223.59093498133,301.679300161882,814.57762068212));
#52829=CARTESIAN_POINT('Ctrl Pts',(221.164851213037,298.340082464834,814.577620676692));
#52830=CARTESIAN_POINT('Ctrl Pts',(221.164851213037,298.340082471544,810.450120552033));
#52831=CARTESIAN_POINT('Ctrl Pts',(221.164851213037,298.340082478254,806.322620427374));
#52832=CARTESIAN_POINT('Ctrl Pts',(223.59093498133,301.679300175303,806.322620432803));
#52833=CARTESIAN_POINT('Origin',(228.30724165054,298.25270265549,810.441761811954));
#52834=CARTESIAN_POINT('Ctrl Pts',(298.461074893041,153.429954409153,810.458479290597));
#52835=CARTESIAN_POINT('Ctrl Pts',(298.469433631005,153.429954409156,810.458479290597));
#52836=CARTESIAN_POINT('Ctrl Pts',(298.469433631005,153.429954409155,810.450120552633));
#52837=CARTESIAN_POINT('Ctrl Pts',(298.469433631005,153.429954409154,810.441761814669));
#52838=CARTESIAN_POINT('Ctrl Pts',(298.461074893041,153.429954409152,810.441761814669));
#52839=CARTESIAN_POINT('Ctrl Pts',(298.452716155077,153.429954409149,810.441761814669));
#52840=CARTESIAN_POINT('Ctrl Pts',(298.452716155077,153.42995440915,810.450120552633));
#52841=CARTESIAN_POINT('Ctrl Pts',(298.452716155077,153.429954409151,810.458479290597));
#52842=CARTESIAN_POINT('Ctrl Pts',(298.461074893041,153.429954409153,810.458479290597));
#52843=CARTESIAN_POINT('Ctrl Pts',(298.461074893041,153.429954408731,812.725856457163));
#52844=CARTESIAN_POINT('Ctrl Pts',(300.736810797571,153.429954409393,812.725856457163));
#52845=CARTESIAN_POINT('Ctrl Pts',(300.736810797571,153.429954409158,810.450120552633));
#52846=CARTESIAN_POINT('Ctrl Pts',(300.736810797571,153.429954408923,808.174384648103));
#52847=CARTESIAN_POINT('Ctrl Pts',(298.461074893041,153.429954408261,808.174384648103));
#52848=CARTESIAN_POINT('Ctrl Pts',(296.185338988511,153.429954407599,808.174384648103));
#52849=CARTESIAN_POINT('Ctrl Pts',(296.185338988511,153.429954407834,810.450120552633));
#52850=CARTESIAN_POINT('Ctrl Pts',(296.185338988511,153.429954408069,812.725856457163));
#52851=CARTESIAN_POINT('Ctrl Pts',(298.461074893041,153.429954408731,812.725856457163));
#52852=CARTESIAN_POINT('Ctrl Pts',(298.46107489266,154.738376719567,814.577620554443));
#52853=CARTESIAN_POINT('Ctrl Pts',(302.588574894606,154.738376720767,814.577620554443));
#52854=CARTESIAN_POINT('Ctrl Pts',(302.588574894605,154.738376720341,810.450120552497));
#52855=CARTESIAN_POINT('Ctrl Pts',(302.588574894605,154.738376719914,806.322620550552));
#52856=CARTESIAN_POINT('Ctrl Pts',(298.46107489266,154.738376718714,806.322620550552));
#52857=CARTESIAN_POINT('Ctrl Pts',(294.333574890715,154.738376717513,806.322620550552));
#52858=CARTESIAN_POINT('Ctrl Pts',(294.333574890715,154.73837671794,810.450120552497));
#52859=CARTESIAN_POINT('Ctrl Pts',(294.333574890715,154.738376718366,814.577620554443));
#52860=CARTESIAN_POINT('Ctrl Pts',(298.46107489266,154.738376719567,814.577620554443));
#52861=CARTESIAN_POINT('Origin',(298.461074890965,160.568052534774,810.458479291925));
#52862=CARTESIAN_POINT('Origin',(298.461074890952,247.282959303211,836.688320551891));
#52863=CARTESIAN_POINT('',(389.393074890952,247.282959303217,836.688320551891));
#52864=CARTESIAN_POINT('',(298.461074890946,338.214959303211,836.68832055189));
#52865=CARTESIAN_POINT('Origin',(298.461074890952,247.282959303211,836.688320551891));
#52866=CARTESIAN_POINT('Origin',(298.461074890952,247.282959303211,836.688320551891));
#52867=CARTESIAN_POINT('',(298.461074890947,319.164959303212,855.73832055189));
#52868=CARTESIAN_POINT('Origin',(298.461074890947,319.164959303212,836.68832055189));
#52869=CARTESIAN_POINT('Origin',(298.461074890952,247.282959303211,855.738320551891));
#52870=CARTESIAN_POINT('Origin',(298.461074890952,247.282959303211,814.463320551891));
#52871=CARTESIAN_POINT('',(389.393074890952,247.282959303217,814.463320551891));
#52872=CARTESIAN_POINT('Origin',(298.461074890948,319.190359303212,855.73832055189));
#52873=CARTESIAN_POINT('Origin',(298.461074890952,234.811559303209,601.738320551891));
#52874=CARTESIAN_POINT('',(310.907074890952,247.28295930321,601.738320551891));
#52875=CARTESIAN_POINT('Origin',(298.461074890952,247.282959303209,601.738320551891));
#52876=CARTESIAN_POINT('Origin',(298.461074890952,247.28295930321,696.988320551891));
#52877=CARTESIAN_POINT('',(215.530074890952,247.282959303204,601.738320551891));
#52878=CARTESIAN_POINT('',(215.530074890952,247.282959303205,696.988320551891));
#52879=CARTESIAN_POINT('',(230.969667895203,199.091043562764,601.738320551892));
#52880=CARTESIAN_POINT('Origin',(298.461074890952,247.282959303209,601.738320551891));
#52881=CARTESIAN_POINT('Origin',(298.461074890952,247.282959303209,601.738320551891));
#52882=CARTESIAN_POINT('Origin',(328.699774890951,246.571759303211,559.345720551891));
#52883=CARTESIAN_POINT('',(329.398274890951,246.571759303211,557.521862913425));
#52884=CARTESIAN_POINT('',(328.001274890951,246.571759303211,558.102555467932));
#52885=CARTESIAN_POINT('Origin',(330.846074890951,246.571759303211,562.97566630189));
#52886=CARTESIAN_POINT('',(328.001274890951,246.571759303211,559.320320551891));
#52887=CARTESIAN_POINT('',(328.001274890951,246.571759303211,559.320320551891));
#52888=CARTESIAN_POINT('',(329.398274890951,246.571759303211,559.320320551891));
#52889=CARTESIAN_POINT('',(329.398274890951,246.571759303211,559.320320551891));
#52890=CARTESIAN_POINT('',(329.398274890951,246.571759303211,559.320320551891));
#52891=CARTESIAN_POINT('Origin',(330.846074890951,250.153159303211,559.320320551891));
#52892=CARTESIAN_POINT('',(328.001274890951,247.994159303211,559.320320551891));
#52893=CARTESIAN_POINT('',(328.001274890951,246.571759303211,559.320320551891));
#52894=CARTESIAN_POINT('',(329.398274890951,247.994159303211,559.320320551891));
#52895=CARTESIAN_POINT('',(328.001274890951,247.994159303211,559.320320551891));
#52896=CARTESIAN_POINT('',(330.134874890951,248.730759303211,559.320320551891));
#52897=CARTESIAN_POINT('',(329.398274890951,247.994159303211,559.320320551891));
#52898=CARTESIAN_POINT('',(330.134874890951,250.127759303211,559.320320551891));
#52899=CARTESIAN_POINT('',(330.134874890951,248.730759303211,559.320320551891));
#52900=CARTESIAN_POINT('',(331.557274890951,250.127759303211,559.320320551891));
#52901=CARTESIAN_POINT('',(330.134874890951,250.127759303211,559.320320551891));
#52902=CARTESIAN_POINT('',(331.557274890951,248.730759303211,559.320320551891));
#52903=CARTESIAN_POINT('',(331.557274890951,250.127759303211,559.320320551891));
#52904=CARTESIAN_POINT('',(332.293874890951,247.994159303211,559.320320551891));
#52905=CARTESIAN_POINT('',(331.557274890951,248.730759303211,559.320320551891));
#52906=CARTESIAN_POINT('',(333.690874890951,247.994159303211,559.320320551891));
#52907=CARTESIAN_POINT('',(332.293874890951,247.994159303211,559.320320551891));
#52908=CARTESIAN_POINT('',(333.690874890951,246.571759303211,559.320320551891));
#52909=CARTESIAN_POINT('',(333.690874890951,247.994159303211,559.320320551891));
#52910=CARTESIAN_POINT('',(332.293874890951,246.571759303211,559.320320551891));
#52911=CARTESIAN_POINT('',(333.690874890951,246.571759303211,559.320320551891));
#52912=CARTESIAN_POINT('',(331.557274890951,245.835159303211,559.320320551891));
#52913=CARTESIAN_POINT('',(332.293874890951,246.571759303211,559.320320551891));
#52914=CARTESIAN_POINT('',(331.557274890952,244.438159303211,559.320320551891));
#52915=CARTESIAN_POINT('',(331.557274890951,245.835159303211,559.320320551891));
#52916=CARTESIAN_POINT('',(330.134874890952,244.438159303211,559.320320551891));
#52917=CARTESIAN_POINT('',(331.557274890952,244.438159303211,559.320320551891));
#52918=CARTESIAN_POINT('',(330.134874890951,245.835159303211,559.320320551891));
#52919=CARTESIAN_POINT('',(330.134874890952,244.438159303211,559.320320551891));
#52920=CARTESIAN_POINT('',(330.134874890951,245.835159303211,559.320320551891));
#52921=CARTESIAN_POINT('Origin',(329.766574890951,246.203459303211,559.345720551891));
#52922=CARTESIAN_POINT('',(330.134874890951,245.835159303211,557.521862913425));
#52923=CARTESIAN_POINT('Origin',(329.766574890951,246.20345930321,562.975666301901));
#52924=CARTESIAN_POINT('',(330.134874890951,245.835159303211,559.320320551891));
#52925=CARTESIAN_POINT('Origin',(263.586874890952,244.514359303207,576.363720551891));
#52926=CARTESIAN_POINT('',(266.050674890952,244.514359303207,560.082320551891));
#52927=CARTESIAN_POINT('',(266.050674890952,244.514359303207,576.338320551891));
#52928=CARTESIAN_POINT('',(266.050674890952,244.514359303207,560.082320551891));
#52929=CARTESIAN_POINT('',(262.232252516023,244.514359303207,560.082320551891));
#52930=CARTESIAN_POINT('',(266.050674890952,244.514359303207,560.082320551891));
#52931=CARTESIAN_POINT('',(262.232252516023,244.514359303207,559.828320551891));
#52932=CARTESIAN_POINT('',(262.232252516023,244.514359303207,560.082320551891));
#52933=CARTESIAN_POINT('',(261.123074890952,244.514359303206,559.828320551891));
#52934=CARTESIAN_POINT('',(261.123074890952,244.514359303206,559.828320551891));
#52935=CARTESIAN_POINT('',(261.123074890952,244.514359303207,576.338320551891));
#52936=CARTESIAN_POINT('',(261.123074890952,244.514359303206,559.828320551891));
#52937=CARTESIAN_POINT('',(266.050674890952,244.514359303207,576.338320551891));
#52938=CARTESIAN_POINT('Origin',(263.586874890951,250.051559303207,576.363720551891));
#52939=CARTESIAN_POINT('',(262.232252516023,250.051559303207,559.828320551891));
#52940=CARTESIAN_POINT('',(262.232252516023,250.051559303207,560.082320551891));
#52941=CARTESIAN_POINT('',(262.232252516023,250.051559303207,559.828320551891));
#52942=CARTESIAN_POINT('',(266.050674890951,250.051559303207,560.082320551891));
#52943=CARTESIAN_POINT('',(262.232252516023,250.051559303207,560.082320551891));
#52944=CARTESIAN_POINT('',(266.050674890951,250.051559303207,576.338320551891));
#52945=CARTESIAN_POINT('',(266.050674890951,250.051559303207,560.082320551891));
#52946=CARTESIAN_POINT('',(261.123074890951,250.051559303207,576.338320551891));
#52947=CARTESIAN_POINT('',(261.123074890951,250.051559303207,576.338320551891));
#52948=CARTESIAN_POINT('',(261.123074890951,250.051559303206,559.828320551891));
#52949=CARTESIAN_POINT('',(261.123074890951,250.051559303206,559.828320551891));
#52950=CARTESIAN_POINT('',(262.232252516023,250.051559303207,559.828320551891));
#52951=CARTESIAN_POINT('Origin',(333.335274890951,252.388359303211,559.828320551891));
#52952=CARTESIAN_POINT('',(335.799074890951,242.202959303211,559.828320551891));
#52953=CARTESIAN_POINT('',(330.871474890952,242.202959303211,559.828320551891));
#52954=CARTESIAN_POINT('',(335.799074890951,242.202959303211,559.828320551891));
#52955=CARTESIAN_POINT('',(330.871474890951,252.362959303211,559.828320551891));
#52956=CARTESIAN_POINT('Origin',(330.871474890952,247.282959303211,559.828320551891));
#52957=CARTESIAN_POINT('',(335.799074890951,252.362959303212,559.828320551891));
#52958=CARTESIAN_POINT('',(330.871474890951,252.362959303211,559.828320551891));
#52959=CARTESIAN_POINT('Origin',(335.799074890951,247.282959303211,559.828320551891));
#52960=CARTESIAN_POINT('',(334.68989726588,244.514359303211,559.828320551891));
#52961=CARTESIAN_POINT('',(334.689897265879,250.051559303212,559.828320551891));
#52962=CARTESIAN_POINT('Origin',(330.846074890951,247.282959303211,559.828320551891));
#52963=CARTESIAN_POINT('',(335.799074890951,244.514359303211,559.828320551891));
#52964=CARTESIAN_POINT('',(334.68989726588,244.514359303211,559.828320551891));
#52965=CARTESIAN_POINT('',(335.799074890951,250.051559303212,559.828320551891));
#52966=CARTESIAN_POINT('Origin',(335.799074890951,247.282959303211,559.828320551891));
#52967=CARTESIAN_POINT('',(335.799074890951,250.051559303212,559.828320551891));
#52968=CARTESIAN_POINT('Origin',(335.799074890951,247.282959303211,560.082320551891));
#52969=CARTESIAN_POINT('',(335.799074890951,242.202959303211,560.336320551891));
#52970=CARTESIAN_POINT('',(335.799074890951,252.362959303212,560.336320551891));
#52971=CARTESIAN_POINT('Origin',(335.799074890951,247.282959303211,560.336320551891));
#52972=CARTESIAN_POINT('',(335.799074890951,242.202959303211,559.828320551891));
#52973=CARTESIAN_POINT('',(335.799074890951,252.362959303212,559.828320551891));
#52974=CARTESIAN_POINT('Origin',(333.335274890951,252.362959303211,560.361720551891));
#52975=CARTESIAN_POINT('',(330.871474890951,252.362959303211,560.336320551891));
#52976=CARTESIAN_POINT('',(335.799074890951,252.362959303212,560.336320551891));
#52977=CARTESIAN_POINT('',(330.871474890951,252.362959303211,559.828320551891));
#52978=CARTESIAN_POINT('Origin',(330.871474890952,247.282959303211,560.082320551891));
#52979=CARTESIAN_POINT('',(330.871474890952,242.202959303211,560.336320551891));
#52980=CARTESIAN_POINT('Origin',(330.871474890952,247.282959303211,560.336320551891));
#52981=CARTESIAN_POINT('',(330.871474890952,242.202959303211,559.828320551891));
#52982=CARTESIAN_POINT('Origin',(333.335274890952,242.202959303211,560.361720551891));
#52983=CARTESIAN_POINT('',(330.871474890952,242.202959303211,560.336320551891));
#52984=CARTESIAN_POINT('Origin',(263.586874890951,252.388359303207,559.828320551891));
#52985=CARTESIAN_POINT('',(266.050674890952,242.202959303207,559.828320551891));
#52986=CARTESIAN_POINT('',(261.123074890952,242.202959303206,559.828320551891));
#52987=CARTESIAN_POINT('',(266.050674890952,242.202959303207,559.828320551891));
#52988=CARTESIAN_POINT('',(261.123074890951,252.362959303206,559.828320551891));
#52989=CARTESIAN_POINT('Origin',(261.123074890951,247.282959303206,559.828320551891));
#52990=CARTESIAN_POINT('',(266.050674890951,252.362959303207,559.828320551891));
#52991=CARTESIAN_POINT('',(261.123074890951,252.362959303206,559.828320551891));
#52992=CARTESIAN_POINT('Origin',(266.050674890951,247.282959303207,559.828320551891));
#52993=CARTESIAN_POINT('Origin',(266.076074890951,247.282959303207,559.828320551891));
#52994=CARTESIAN_POINT('Origin',(261.123074890951,247.282959303206,559.828320551891));
#52995=CARTESIAN_POINT('Origin',(266.050674890951,247.282959303207,560.082320551891));
#52996=CARTESIAN_POINT('',(266.050674890952,242.202959303207,560.336320551891));
#52997=CARTESIAN_POINT('',(266.050674890951,252.362959303207,560.336320551891));
#52998=CARTESIAN_POINT('Origin',(266.050674890951,247.282959303207,560.336320551891));
#52999=CARTESIAN_POINT('',(266.050674890952,242.202959303207,559.828320551891));
#53000=CARTESIAN_POINT('',(266.050674890951,252.362959303207,559.828320551891));
#53001=CARTESIAN_POINT('Origin',(263.586874890951,252.362959303207,560.361720551891));
#53002=CARTESIAN_POINT('',(261.123074890951,252.362959303206,560.336320551891));
#53003=CARTESIAN_POINT('',(266.050674890951,252.362959303207,560.336320551891));
#53004=CARTESIAN_POINT('',(261.123074890951,252.362959303206,559.828320551891));
#53005=CARTESIAN_POINT('Origin',(261.123074890951,247.282959303206,560.082320551891));
#53006=CARTESIAN_POINT('',(261.123074890952,242.202959303206,560.336320551891));
#53007=CARTESIAN_POINT('Origin',(261.123074890951,247.282959303206,560.336320551891));
#53008=CARTESIAN_POINT('',(261.123074890952,242.202959303206,559.828320551891));
#53009=CARTESIAN_POINT('Origin',(263.586874890952,242.202959303207,560.361720551891));
#53010=CARTESIAN_POINT('',(261.123074890952,242.202959303206,560.336320551891));
#53011=CARTESIAN_POINT('Origin',(245.702070179666,303.970074014487,585.736320551891));
#53012=CARTESIAN_POINT('',(241.799360179667,300.041964014487,585.736320551891));
#53013=CARTESIAN_POINT('Origin',(245.702070179667,300.041964014487,585.736320551891));
#53014=CARTESIAN_POINT('Origin',(245.702070179667,300.041964014487,573.466215551891));
#53015=CARTESIAN_POINT('',(241.799360179667,300.041964014486,561.196110551891));
#53016=CARTESIAN_POINT('',(241.799360179667,300.041964014486,573.466215551891));
#53017=CARTESIAN_POINT('',(248.878197188823,297.774065743884,561.196110551891));
#53018=CARTESIAN_POINT('Origin',(245.702070179667,300.041964014487,561.196110551891));
#53019=CARTESIAN_POINT('Origin',(245.702070179667,300.041964014487,561.196110551891));
#53020=CARTESIAN_POINT('Origin',(245.702070179667,300.041964014486,561.110131551891));
#53021=CARTESIAN_POINT('',(249.57791667636,297.274434396927,560.336320551891));
#53022=CARTESIAN_POINT('',(248.948169137577,297.724102609188,561.110131551891));
#53023=CARTESIAN_POINT('Origin',(245.702070179667,300.041964014487,560.336320551891));
#53024=CARTESIAN_POINT('Origin',(351.220079602236,198.452064591931,585.736320551891));
#53025=CARTESIAN_POINT('',(347.317369602236,194.523954591931,585.736320551891));
#53026=CARTESIAN_POINT('Origin',(351.220079602236,194.523954591931,585.736320551891));
#53027=CARTESIAN_POINT('Origin',(351.220079602236,194.523954591931,573.466215551891));
#53028=CARTESIAN_POINT('',(347.317369602236,194.523954591931,561.196110551891));
#53029=CARTESIAN_POINT('',(347.317369602236,194.523954591931,573.466215551891));
#53030=CARTESIAN_POINT('',(354.396206611393,192.256056321328,561.196110551891));
#53031=CARTESIAN_POINT('Origin',(351.220079602236,194.523954591931,561.196110551891));
#53032=CARTESIAN_POINT('Origin',(351.220079602236,194.523954591931,561.196110551891));
#53033=CARTESIAN_POINT('Origin',(351.220079602236,194.523954591931,561.110131551891));
#53034=CARTESIAN_POINT('',(355.09592609893,191.756424974372,560.336320551891));
#53035=CARTESIAN_POINT('',(354.466178560147,192.206093186633,561.110131551891));
#53036=CARTESIAN_POINT('Origin',(351.220079602236,194.523954591931,560.336320551891));
#53037=CARTESIAN_POINT('Origin',(351.220079602229,303.970074014494,585.73632055189));
#53038=CARTESIAN_POINT('',(347.317369602229,300.041964014494,585.73632055189));
#53039=CARTESIAN_POINT('Origin',(351.220079602229,300.041964014494,585.73632055189));
#53040=CARTESIAN_POINT('Origin',(351.220079602229,300.041964014494,573.46621555189));
#53041=CARTESIAN_POINT('',(347.317369602229,300.041964014493,561.19611055189));
#53042=CARTESIAN_POINT('',(347.317369602229,300.041964014494,573.46621555189));
#53043=CARTESIAN_POINT('',(354.396206611386,297.774065743891,561.19611055189));
#53044=CARTESIAN_POINT('Origin',(351.220079602229,300.041964014494,561.19611055189));
#53045=CARTESIAN_POINT('Origin',(351.220079602229,300.041964014494,561.19611055189));
#53046=CARTESIAN_POINT('Origin',(351.220079602229,300.041964014494,561.11013155189));
#53047=CARTESIAN_POINT('',(355.095926098923,297.274434396934,560.33632055189));
#53048=CARTESIAN_POINT('',(354.46617856014,297.724102609195,561.11013155189));
#53049=CARTESIAN_POINT('Origin',(351.220079602229,300.041964014494,560.33632055189));
#53050=CARTESIAN_POINT('Origin',(245.702070179674,198.452064591924,585.736320551892));
#53051=CARTESIAN_POINT('',(241.799360179674,194.523954591924,585.736320551892));
#53052=CARTESIAN_POINT('Origin',(245.702070179674,194.523954591924,585.736320551892));
#53053=CARTESIAN_POINT('Origin',(245.702070179674,194.523954591924,573.466215551892));
#53054=CARTESIAN_POINT('',(241.799360179674,194.523954591924,561.196110551892));
#53055=CARTESIAN_POINT('',(241.799360179674,194.523954591924,573.466215551892));
#53056=CARTESIAN_POINT('',(248.878197188831,192.256056321321,561.196110551892));
#53057=CARTESIAN_POINT('Origin',(245.702070179674,194.523954591924,561.196110551892));
#53058=CARTESIAN_POINT('Origin',(245.702070179674,194.523954591924,561.196110551892));
#53059=CARTESIAN_POINT('Origin',(245.702070179674,194.523954591924,561.110131551892));
#53060=CARTESIAN_POINT('',(249.577916676367,191.756424974365,560.336320551892));
#53061=CARTESIAN_POINT('',(248.948169137584,192.206093186626,561.110131551892));
#53062=CARTESIAN_POINT('Origin',(245.702070179674,194.523954591924,560.336320551892));
#53063=CARTESIAN_POINT('Origin',(298.461074890952,247.28295930321,597.598120551891));
#53064=CARTESIAN_POINT('',(231.557799298777,199.510995973107,560.336320551892));
#53065=CARTESIAN_POINT('',(231.028481035561,199.133038803798,597.598120551892));
#53066=CARTESIAN_POINT('Origin',(298.461074890951,247.282959303209,560.336320551891));
#53067=CARTESIAN_POINT('Origin',(298.461074890946,329.516684705051,560.33632055189));
#53068=CARTESIAN_POINT('',(307.224074890956,175.45175930321,560.336320551892));
#53069=CARTESIAN_POINT('Origin',(298.461074890956,175.451759303209,560.336320551892));
#53070=CARTESIAN_POINT('',(217.866874890951,247.282959303203,560.336320551891));
#53071=CARTESIAN_POINT('Origin',(226.629874890951,247.282959303204,560.336320551891));
#53072=CARTESIAN_POINT('',(379.055274890951,247.282959303214,560.336320551891));
#53073=CARTESIAN_POINT('Origin',(370.292274890951,247.282959303214,560.336320551891));
#53074=CARTESIAN_POINT('',(289.698074890947,319.114159303208,560.33632055189));
#53075=CARTESIAN_POINT('Origin',(298.461074890947,319.114159303209,560.33632055189));
#53076=CARTESIAN_POINT('',(355.611074890951,247.282959303213,560.336320551891));
#53077=CARTESIAN_POINT('Origin',(298.461074890951,247.282959303209,560.336320551891));
#53078=CARTESIAN_POINT('Origin',(298.461074890951,247.282959303209,558.812320551891));
#53079=CARTESIAN_POINT('',(355.611074890951,247.282959303213,557.288320551891));
#53080=CARTESIAN_POINT('',(355.611074890951,247.282959303213,558.812320551891));
#53081=CARTESIAN_POINT('Origin',(298.461074890951,247.282959303209,557.288320551891));
#53082=CARTESIAN_POINT('Origin',(298.461074890948,304.458359303209,557.288320551891));
#53083=CARTESIAN_POINT('',(350.912074890951,247.282959303212,557.288320551891));
#53084=CARTESIAN_POINT('Origin',(298.461074890951,247.282959303209,557.288320551891));
#53085=CARTESIAN_POINT('Origin',(298.461074890951,247.282959303209,558.812320551891));
#53086=CARTESIAN_POINT('',(350.912074890951,247.282959303212,560.336320551891));
#53087=CARTESIAN_POINT('',(350.912074890951,247.282959303212,558.812320551891));
#53088=CARTESIAN_POINT('Origin',(298.461074890951,247.282959303209,560.336320551891));
#53089=CARTESIAN_POINT('Origin',(298.461074890948,299.759359303209,560.336320551891));
#53090=CARTESIAN_POINT('',(311.542074890951,247.28295930321,560.336320551891));
#53091=CARTESIAN_POINT('Origin',(298.461074890951,247.282959303209,560.336320551891));
#53092=CARTESIAN_POINT('Origin',(298.461074890951,247.282959303209,558.812320551891));
#53093=CARTESIAN_POINT('',(311.542074890951,247.28295930321,557.288320551891));
#53094=CARTESIAN_POINT('',(311.542074890951,247.28295930321,558.812320551891));
#53095=CARTESIAN_POINT('Origin',(298.461074890951,247.282959303209,557.288320551891));
#53096=CARTESIAN_POINT('Origin',(298.46107489095,260.389359303209,557.288320551891));
#53097=CARTESIAN_POINT('',(310.907074890951,247.28295930321,557.288320551891));
#53098=CARTESIAN_POINT('Origin',(298.461074890951,247.282959303209,557.288320551891));
#53099=CARTESIAN_POINT('Origin',(298.461074890951,247.282959303209,579.513320551891));
#53100=CARTESIAN_POINT('',(310.907074890951,247.28295930321,579.513320551891));
#53101=CARTESIAN_POINT('Origin',(298.461074890956,184.240159303209,567.956320551892));
#53102=CARTESIAN_POINT('',(307.224074890956,175.45175930321,567.956320551892));
#53103=CARTESIAN_POINT('Origin',(298.461074890956,175.451759303209,567.956320551892));
#53104=CARTESIAN_POINT('',(301.255074890956,175.451759303209,567.956320551892));
#53105=CARTESIAN_POINT('Origin',(298.461074890956,175.451759303209,567.956320551892));
#53106=CARTESIAN_POINT('Origin',(298.461074890956,175.451759303209,564.146320551892));
#53107=CARTESIAN_POINT('',(307.224074890956,175.45175930321,564.146320551892));
#53108=CARTESIAN_POINT('Origin',(298.461074890956,175.451759303209,571.766320551892));
#53109=CARTESIAN_POINT('',(301.255074890956,175.451759303209,575.576320551892));
#53110=CARTESIAN_POINT('',(301.255074890956,175.451759303209,571.766320551892));
#53111=CARTESIAN_POINT('Origin',(298.461074890956,175.451759303209,575.576320551892));
#53112=CARTESIAN_POINT('Origin',(298.461074890956,178.271159303209,575.576320551892));
#53113=CARTESIAN_POINT('Origin',(298.461074890947,319.114159303209,564.14632055189));
#53114=CARTESIAN_POINT('',(289.698074890947,319.114159303208,567.95632055189));
#53115=CARTESIAN_POINT('Origin',(298.461074890947,319.114159303209,567.95632055189));
#53116=CARTESIAN_POINT('',(289.698074890947,319.114159303208,564.14632055189));
#53117=CARTESIAN_POINT('Origin',(298.461074890946,327.902559303209,567.95632055189));
#53118=CARTESIAN_POINT('',(295.667074890947,319.114159303209,567.95632055189));
#53119=CARTESIAN_POINT('Origin',(298.461074890947,319.114159303209,567.95632055189));
#53120=CARTESIAN_POINT('Origin',(298.461074890947,319.114159303209,571.76632055189));
#53121=CARTESIAN_POINT('',(295.667074890947,319.114159303209,575.57632055189));
#53122=CARTESIAN_POINT('Origin',(298.461074890947,319.114159303209,575.57632055189));
#53123=CARTESIAN_POINT('',(295.667074890947,319.114159303209,571.76632055189));
#53124=CARTESIAN_POINT('Origin',(298.461074890946,321.933559303209,575.57632055189));
#53125=CARTESIAN_POINT('Origin',(370.292274890951,250.102359303214,575.576320551891));
#53126=CARTESIAN_POINT('',(373.086274890951,247.282959303214,575.576320551891));
#53127=CARTESIAN_POINT('Origin',(370.292274890951,247.282959303214,575.576320551891));
#53128=CARTESIAN_POINT('Origin',(370.292274890951,247.282959303214,571.766320551891));
#53129=CARTESIAN_POINT('',(373.086274890951,247.282959303214,567.956320551891));
#53130=CARTESIAN_POINT('Origin',(370.292274890951,247.282959303214,567.956320551891));
#53131=CARTESIAN_POINT('',(373.086274890951,247.282959303214,571.766320551891));
#53132=CARTESIAN_POINT('Origin',(370.292274890951,256.071359303214,567.956320551891));
#53133=CARTESIAN_POINT('',(379.055274890951,247.282959303214,567.956320551891));
#53134=CARTESIAN_POINT('Origin',(370.292274890951,247.282959303214,567.956320551891));
#53135=CARTESIAN_POINT('Origin',(370.292274890951,247.282959303214,564.146320551891));
#53136=CARTESIAN_POINT('',(379.055274890951,247.282959303214,564.146320551891));
#53137=CARTESIAN_POINT('Origin',(226.629874890951,247.282959303204,564.146320551891));
#53138=CARTESIAN_POINT('',(217.866874890951,247.282959303204,567.956320551891));
#53139=CARTESIAN_POINT('Origin',(226.629874890951,247.282959303204,567.956320551891));
#53140=CARTESIAN_POINT('',(217.866874890951,247.282959303204,564.146320551891));
#53141=CARTESIAN_POINT('Origin',(226.629874890951,256.071359303204,567.956320551891));
#53142=CARTESIAN_POINT('',(223.835874890951,247.282959303204,567.956320551891));
#53143=CARTESIAN_POINT('Origin',(226.629874890951,247.282959303204,567.956320551891));
#53144=CARTESIAN_POINT('Origin',(226.629874890951,247.282959303204,571.766320551891));
#53145=CARTESIAN_POINT('',(223.835874890951,247.282959303204,575.576320551891));
#53146=CARTESIAN_POINT('Origin',(226.629874890951,247.282959303204,575.576320551891));
#53147=CARTESIAN_POINT('',(223.835874890951,247.282959303204,571.766320551891));
#53148=CARTESIAN_POINT('Origin',(226.629874890951,250.102359303204,575.576320551891));
#53149=CARTESIAN_POINT('Origin',(333.335274890952,250.051559303212,576.363720551891));
#53150=CARTESIAN_POINT('',(330.871474890952,250.051559303212,560.082320551891));
#53151=CARTESIAN_POINT('',(330.871474890952,250.051559303212,576.338320551891));
#53152=CARTESIAN_POINT('',(330.871474890952,250.051559303212,560.082320551891));
#53153=CARTESIAN_POINT('',(334.689897265879,250.051559303212,560.082320551891));
#53154=CARTESIAN_POINT('',(330.871474890952,250.051559303212,560.082320551891));
#53155=CARTESIAN_POINT('',(334.689897265879,250.051559303212,560.082320551891));
#53156=CARTESIAN_POINT('',(335.799074890951,250.051559303212,576.338320551891));
#53157=CARTESIAN_POINT('',(335.799074890951,250.051559303212,559.828320551891));
#53158=CARTESIAN_POINT('',(330.871474890952,250.051559303212,576.338320551891));
#53159=CARTESIAN_POINT('Origin',(330.871474890952,247.282959303211,568.210320551891));
#53160=CARTESIAN_POINT('',(330.871474890952,244.514359303211,560.082320551891));
#53161=CARTESIAN_POINT('',(330.871474890952,244.514359303211,576.338320551891));
#53162=CARTESIAN_POINT('',(330.871474890952,244.514359303211,560.082320551891));
#53163=CARTESIAN_POINT('Origin',(330.871474890952,247.282959303211,560.082320551891));
#53164=CARTESIAN_POINT('Origin',(330.871474890952,247.282959303211,576.338320551891));
#53165=CARTESIAN_POINT('Origin',(333.335274890952,244.514359303211,576.363720551891));
#53166=CARTESIAN_POINT('',(334.68989726588,244.514359303211,560.082320551891));
#53167=CARTESIAN_POINT('',(334.68989726588,244.514359303211,559.828320551891));
#53168=CARTESIAN_POINT('',(334.68989726588,244.514359303211,560.082320551891));
#53169=CARTESIAN_POINT('',(335.799074890951,244.514359303211,576.338320551891));
#53170=CARTESIAN_POINT('',(335.799074890951,244.514359303211,576.338320551891));
#53171=CARTESIAN_POINT('',(335.799074890951,244.514359303211,559.828320551891));
#53172=CARTESIAN_POINT('Origin',(263.586874890951,250.076959303207,576.338320551891));
#53173=CARTESIAN_POINT('Origin',(261.123074890951,247.282959303207,576.338320551891));
#53174=CARTESIAN_POINT('Origin',(266.050674890951,247.282959303207,576.338320551891));
#53175=CARTESIAN_POINT('',(268.260474890951,247.282959303207,576.338320551891));
#53176=CARTESIAN_POINT('Origin',(266.076074890951,247.282959303207,576.338320551891));
#53177=CARTESIAN_POINT('Origin',(266.050674890951,247.282959303207,568.210320551891));
#53178=CARTESIAN_POINT('Origin',(266.050674890951,247.282959303207,560.082320551891));
#53179=CARTESIAN_POINT('Origin',(261.123074890951,247.282959303206,568.083320551891));
#53180=CARTESIAN_POINT('Origin',(335.799074890951,247.282959303211,568.083320551891));
#53181=CARTESIAN_POINT('Origin',(335.799074890951,247.282959303212,576.338320551891));
#53182=CARTESIAN_POINT('Origin',(333.335274890951,250.076959303212,576.338320551891));
#53183=CARTESIAN_POINT('',(333.030474890951,247.282959303211,576.338320551891));
#53184=CARTESIAN_POINT('Origin',(330.846074890951,247.282959303211,576.338320551891));
#53185=CARTESIAN_POINT('Origin',(330.846074890952,247.282959303211,559.955320551891));
#53186=CARTESIAN_POINT('Origin',(330.846074890952,247.282959303211,559.828320551891));
#53187=CARTESIAN_POINT('Origin',(330.846074890952,247.282959303211,560.082320551891));
#53188=CARTESIAN_POINT('Origin',(330.846074890951,247.282959303211,568.210320551891));
#53189=CARTESIAN_POINT('',(333.030474890951,247.282959303211,560.082320551891));
#53190=CARTESIAN_POINT('',(333.030474890951,247.282959303211,568.210320551891));
#53191=CARTESIAN_POINT('Origin',(330.846074890951,247.282959303211,560.082320551891));
#53192=CARTESIAN_POINT('Origin',(332.39345946167,250.076959303212,560.082320551891));
#53193=CARTESIAN_POINT('Origin',(330.846074890952,247.282959303211,562.975666301891));
#53194=CARTESIAN_POINT('',(333.690874890951,247.994159303211,558.102555467932));
#53195=CARTESIAN_POINT('',(333.690874890951,246.571759303211,558.102555467932));
#53196=CARTESIAN_POINT('Origin',(333.690874890951,247.282959303212,562.975666301898));
#53197=CARTESIAN_POINT('',(332.293874890951,247.994159303211,557.521862913425));
#53198=CARTESIAN_POINT('Origin',(330.846074890952,247.994159303211,562.97566630189));
#53199=CARTESIAN_POINT('',(331.557274890951,248.730759303211,557.521862913425));
#53200=CARTESIAN_POINT('Origin',(331.92557489095,248.36245930321,562.975666301901));
#53201=CARTESIAN_POINT('',(331.557274890951,250.127759303211,558.102555467932));
#53202=CARTESIAN_POINT('Origin',(331.557274890951,247.282959303212,562.975666301888));
#53203=CARTESIAN_POINT('',(330.134874890951,250.127759303211,558.102555467932));
#53204=CARTESIAN_POINT('Origin',(330.846074890951,250.127759303211,562.97566630189));
#53205=CARTESIAN_POINT('',(330.134874890951,248.730759303211,557.521862913425));
#53206=CARTESIAN_POINT('Origin',(330.134874890951,247.282959303212,562.975666301888));
#53207=CARTESIAN_POINT('',(329.398274890951,247.994159303211,557.521862913425));
#53208=CARTESIAN_POINT('Origin',(329.766574890951,248.362459303211,562.975666301901));
#53209=CARTESIAN_POINT('',(328.001274890951,247.994159303211,558.102555467932));
#53210=CARTESIAN_POINT('Origin',(330.846074890951,247.994159303211,562.97566630189));
#53211=CARTESIAN_POINT('Origin',(328.001274890952,247.282959303211,562.975666301889));
#53212=CARTESIAN_POINT('',(330.134874890952,244.438159303211,558.102555467932));
#53213=CARTESIAN_POINT('Origin',(330.134874890951,247.282959303211,562.975666301889));
#53214=CARTESIAN_POINT('',(331.557274890952,244.438159303211,558.102555467932));
#53215=CARTESIAN_POINT('Origin',(330.846074890952,244.438159303211,562.97566630189));
#53216=CARTESIAN_POINT('',(331.557274890951,245.835159303211,557.521862913425));
#53217=CARTESIAN_POINT('Origin',(331.557274890951,247.282959303211,562.975666301889));
#53218=CARTESIAN_POINT('',(332.293874890951,246.571759303211,557.521862913425));
#53219=CARTESIAN_POINT('Origin',(331.925574890951,246.203459303212,562.975666301901));
#53220=CARTESIAN_POINT('Origin',(330.846074890952,246.571759303211,562.97566630189));
#53221=CARTESIAN_POINT('Origin',(264.528690320232,250.076959303207,560.082320551891));
#53222=CARTESIAN_POINT('Origin',(266.076074890951,247.282959303207,560.082320551891));
#53223=CARTESIAN_POINT('',(268.260474890951,247.282959303207,560.082320551891));
#53224=CARTESIAN_POINT('Origin',(266.076074890951,247.282959303207,560.082320551891));
#53225=CARTESIAN_POINT('Origin',(266.076074890951,247.282959303207,568.210320551891));
#53226=CARTESIAN_POINT('',(268.260474890952,247.282959303207,568.210320551891));
#53227=CARTESIAN_POINT('Origin',(266.076074890951,247.282959303207,559.955320551891));
#53228=CARTESIAN_POINT('Origin',(266.076074890952,247.282959303207,559.828320551891));
#53229=CARTESIAN_POINT('Origin',(266.076074890951,247.282959303207,562.975666301891));
#53230=CARTESIAN_POINT('',(268.920874890951,247.994159303207,558.102555467933));
#53231=CARTESIAN_POINT('',(268.920874890951,246.571759303207,558.102555467933));
#53232=CARTESIAN_POINT('Origin',(268.920874890953,247.282959303207,562.975666301892));
#53233=CARTESIAN_POINT('',(267.523874890951,247.994159303207,557.521862913425));
#53234=CARTESIAN_POINT('Origin',(266.076074890953,247.994159303207,562.975666301888));
#53235=CARTESIAN_POINT('',(266.787274890951,248.730759303207,557.521862913425));
#53236=CARTESIAN_POINT('Origin',(267.15557489095,248.362459303206,562.975666301897));
#53237=CARTESIAN_POINT('',(266.787274890951,250.127759303207,558.102555467933));
#53238=CARTESIAN_POINT('Origin',(266.787274890951,247.282959303209,562.975666301886));
#53239=CARTESIAN_POINT('',(265.364874890951,250.127759303207,558.102555467933));
#53240=CARTESIAN_POINT('Origin',(266.076074890951,250.127759303207,562.975666301891));
#53241=CARTESIAN_POINT('',(265.364874890951,248.730759303207,557.521862913425));
#53242=CARTESIAN_POINT('Origin',(265.364874890952,247.282959303207,562.975666301891));
#53243=CARTESIAN_POINT('',(264.628274890951,247.994159303207,557.521862913425));
#53244=CARTESIAN_POINT('Origin',(264.996574890949,248.362459303209,562.975666301889));
#53245=CARTESIAN_POINT('',(263.231274890951,247.994159303207,558.102555467933));
#53246=CARTESIAN_POINT('Origin',(266.076074890952,247.994159303207,562.975666301893));
#53247=CARTESIAN_POINT('',(263.231274890951,246.571759303207,558.102555467933));
#53248=CARTESIAN_POINT('Origin',(263.231274890951,247.282959303207,562.975666301891));
#53249=CARTESIAN_POINT('',(264.628274890951,246.571759303207,557.521862913425));
#53250=CARTESIAN_POINT('Origin',(266.076074890952,246.571759303207,562.975666301892));
#53251=CARTESIAN_POINT('',(265.364874890951,245.835159303207,557.521862913425));
#53252=CARTESIAN_POINT('Origin',(264.996574890949,246.203459303204,562.975666301889));
#53253=CARTESIAN_POINT('',(265.364874890952,244.438159303207,558.102555467933));
#53254=CARTESIAN_POINT('Origin',(265.364874890952,247.282959303207,562.975666301891));
#53255=CARTESIAN_POINT('',(266.787274890952,244.438159303207,558.102555467933));
#53256=CARTESIAN_POINT('Origin',(266.076074890952,244.438159303207,562.975666301891));
#53257=CARTESIAN_POINT('',(266.787274890951,245.835159303207,557.521862913425));
#53258=CARTESIAN_POINT('Origin',(266.787274890951,247.282959303207,562.975666301893));
#53259=CARTESIAN_POINT('',(267.523874890951,246.571759303207,557.521862913425));
#53260=CARTESIAN_POINT('Origin',(267.155574890951,246.203459303207,562.975666301901));
#53261=CARTESIAN_POINT('Origin',(266.076074890954,246.571759303207,562.975666301885));
#53262=CARTESIAN_POINT('Origin',(263.929774890951,246.571759303207,559.345720551891));
#53263=CARTESIAN_POINT('',(263.231274890951,246.571759303207,559.320320551891));
#53264=CARTESIAN_POINT('',(263.231274890951,246.571759303207,559.320320551891));
#53265=CARTESIAN_POINT('',(264.628274890951,246.571759303207,559.320320551891));
#53266=CARTESIAN_POINT('',(264.628274890951,246.571759303207,559.320320551891));
#53267=CARTESIAN_POINT('',(264.628274890951,246.571759303207,559.320320551891));
#53268=CARTESIAN_POINT('Origin',(263.231274890951,248.019559303207,558.659540417467));
#53269=CARTESIAN_POINT('',(263.231274890951,247.994159303207,559.320320551891));
#53270=CARTESIAN_POINT('',(263.231274890951,247.994159303207,559.320320551891));
#53271=CARTESIAN_POINT('',(263.231274890951,246.571759303207,559.320320551891));
#53272=CARTESIAN_POINT('Origin',(263.929774890951,247.994159303207,559.345720551891));
#53273=CARTESIAN_POINT('',(264.628274890951,247.994159303207,559.320320551891));
#53274=CARTESIAN_POINT('',(264.628274890951,247.994159303207,559.320320551891));
#53275=CARTESIAN_POINT('',(263.231274890951,247.994159303207,559.320320551891));
#53276=CARTESIAN_POINT('Origin',(264.996574890951,248.362459303207,559.345720551891));
#53277=CARTESIAN_POINT('',(265.364874890951,248.730759303207,559.320320551891));
#53278=CARTESIAN_POINT('',(265.364874890951,248.730759303207,559.320320551891));
#53279=CARTESIAN_POINT('',(264.628274890951,247.994159303207,559.320320551891));
#53280=CARTESIAN_POINT('Origin',(265.364874890951,250.153159303207,558.421091732658));
#53281=CARTESIAN_POINT('',(265.364874890951,250.127759303207,559.320320551891));
#53282=CARTESIAN_POINT('',(265.364874890951,250.127759303207,559.320320551891));
#53283=CARTESIAN_POINT('',(265.364874890951,248.730759303207,559.320320551891));
#53284=CARTESIAN_POINT('Origin',(266.076074890951,250.127759303207,559.345720551891));
#53285=CARTESIAN_POINT('',(266.787274890951,250.127759303207,559.320320551891));
#53286=CARTESIAN_POINT('',(266.787274890951,250.127759303207,559.320320551891));
#53287=CARTESIAN_POINT('',(265.364874890951,250.127759303207,559.320320551891));
#53288=CARTESIAN_POINT('Origin',(266.787274890951,250.153159303207,558.421091732658));
#53289=CARTESIAN_POINT('',(266.787274890951,248.730759303207,559.320320551891));
#53290=CARTESIAN_POINT('',(266.787274890951,248.730759303207,559.320320551891));
#53291=CARTESIAN_POINT('',(266.787274890951,250.127759303207,559.320320551891));
#53292=CARTESIAN_POINT('Origin',(267.155574890951,248.362459303207,559.345720551891));
#53293=CARTESIAN_POINT('',(267.523874890951,247.994159303207,559.320320551891));
#53294=CARTESIAN_POINT('',(267.523874890951,247.994159303207,559.320320551891));
#53295=CARTESIAN_POINT('',(266.787274890951,248.730759303207,559.320320551891));
#53296=CARTESIAN_POINT('Origin',(268.222374890951,247.994159303207,559.345720551891));
#53297=CARTESIAN_POINT('',(268.920874890951,247.994159303207,559.320320551891));
#53298=CARTESIAN_POINT('',(268.920874890951,247.994159303207,559.320320551891));
#53299=CARTESIAN_POINT('',(267.523874890951,247.994159303207,559.320320551891));
#53300=CARTESIAN_POINT('Origin',(268.920874890951,248.019559303207,558.685625936038));
#53301=CARTESIAN_POINT('',(268.920874890951,246.571759303207,559.320320551891));
#53302=CARTESIAN_POINT('',(268.920874890951,246.571759303207,559.320320551891));
#53303=CARTESIAN_POINT('',(268.920874890951,247.994159303207,559.320320551891));
#53304=CARTESIAN_POINT('Origin',(268.222374890951,246.571759303207,559.345720551891));
#53305=CARTESIAN_POINT('',(267.523874890951,246.571759303207,559.320320551891));
#53306=CARTESIAN_POINT('',(267.523874890951,246.571759303207,559.320320551891));
#53307=CARTESIAN_POINT('',(268.920874890951,246.571759303207,559.320320551891));
#53308=CARTESIAN_POINT('Origin',(267.155574890951,246.203459303207,559.345720551891));
#53309=CARTESIAN_POINT('',(266.787274890951,245.835159303207,559.320320551891));
#53310=CARTESIAN_POINT('',(266.787274890951,245.835159303207,559.320320551891));
#53311=CARTESIAN_POINT('',(267.523874890951,246.571759303207,559.320320551891));
#53312=CARTESIAN_POINT('Origin',(266.787274890951,245.860559303207,558.421091732658));
#53313=CARTESIAN_POINT('',(266.787274890952,244.438159303207,559.320320551891));
#53314=CARTESIAN_POINT('',(266.787274890952,244.438159303207,559.320320551891));
#53315=CARTESIAN_POINT('',(266.787274890951,245.835159303207,559.320320551891));
#53316=CARTESIAN_POINT('Origin',(266.076074890952,244.438159303207,559.345720551891));
#53317=CARTESIAN_POINT('',(265.364874890952,244.438159303207,559.320320551891));
#53318=CARTESIAN_POINT('',(265.364874890952,244.438159303207,559.320320551891));
#53319=CARTESIAN_POINT('',(266.787274890952,244.438159303207,559.320320551891));
#53320=CARTESIAN_POINT('Origin',(265.364874890951,245.860559303207,558.421091732658));
#53321=CARTESIAN_POINT('',(265.364874890951,245.835159303207,559.320320551891));
#53322=CARTESIAN_POINT('',(265.364874890951,245.835159303207,559.320320551891));
#53323=CARTESIAN_POINT('',(265.364874890952,244.438159303207,559.320320551891));
#53324=CARTESIAN_POINT('Origin',(264.996574890951,246.203459303207,559.345720551891));
#53325=CARTESIAN_POINT('',(265.364874890951,245.835159303207,559.320320551891));
#53326=CARTESIAN_POINT('Origin',(266.076074890951,250.153159303207,559.320320551891));
#53327=CARTESIAN_POINT('Origin',(328.001274890951,247.282959303211,559.345720551891));
#53328=CARTESIAN_POINT('',(328.001274890951,247.994159303211,559.320320551891));
#53329=CARTESIAN_POINT('Origin',(328.699774890951,247.994159303211,559.345720551891));
#53330=CARTESIAN_POINT('',(329.398274890951,247.994159303211,559.320320551891));
#53331=CARTESIAN_POINT('Origin',(329.766574890951,248.362459303211,559.345720551891));
#53332=CARTESIAN_POINT('',(330.134874890951,248.730759303211,559.320320551891));
#53333=CARTESIAN_POINT('Origin',(330.134874890951,250.153159303211,558.421091732658));
#53334=CARTESIAN_POINT('',(330.134874890951,250.127759303211,559.320320551891));
#53335=CARTESIAN_POINT('Origin',(330.846074890951,250.127759303211,559.345720551891));
#53336=CARTESIAN_POINT('',(331.557274890951,250.127759303211,559.320320551891));
#53337=CARTESIAN_POINT('Origin',(331.557274890951,250.153159303211,558.421091732658));
#53338=CARTESIAN_POINT('',(331.557274890951,248.730759303211,559.320320551891));
#53339=CARTESIAN_POINT('Origin',(331.925574890951,248.362459303211,559.345720551891));
#53340=CARTESIAN_POINT('',(332.293874890951,247.994159303211,559.320320551891));
#53341=CARTESIAN_POINT('Origin',(332.992374890951,247.994159303211,559.345720551891));
#53342=CARTESIAN_POINT('',(333.690874890951,247.994159303211,559.320320551891));
#53343=CARTESIAN_POINT('Origin',(333.690874890951,248.019559303211,558.685625936038));
#53344=CARTESIAN_POINT('',(333.690874890951,246.571759303211,559.320320551891));
#53345=CARTESIAN_POINT('Origin',(332.992374890951,246.571759303211,559.345720551891));
#53346=CARTESIAN_POINT('',(332.293874890951,246.571759303211,559.320320551891));
#53347=CARTESIAN_POINT('Origin',(331.925574890952,246.203459303211,559.345720551891));
#53348=CARTESIAN_POINT('',(331.557274890951,245.835159303211,559.320320551891));
#53349=CARTESIAN_POINT('Origin',(331.557274890951,245.860559303211,558.421091732658));
#53350=CARTESIAN_POINT('',(331.557274890952,244.438159303211,559.320320551891));
#53351=CARTESIAN_POINT('Origin',(330.846074890952,244.438159303211,559.345720551891));
#53352=CARTESIAN_POINT('',(330.134874890952,244.438159303211,559.320320551891));
#53353=CARTESIAN_POINT('Origin',(330.134874890951,245.860559303211,558.421091732658));
#61759=UNCERTAINTY_MEASURE_WITH_UNIT(LENGTH_MEASURE(0.01),#61812,
'DISTANCE_ACCURACY_VALUE',
'Maximum model space distance between geometric entities at asserted c
onnectivities');
#61780=UNCERTAINTY_MEASURE_WITH_UNIT(LENGTH_MEASURE(0.01),#61812,
'DISTANCE_ACCURACY_VALUE',
'Maximum model space distance between geometric entities at asserted c
onnectivities');
#61790=(
GEOMETRIC_REPRESENTATION_CONTEXT(3)
GLOBAL_UNCERTAINTY_ASSIGNED_CONTEXT((#61759))
GLOBAL_UNIT_ASSIGNED_CONTEXT((#61812,#61814,#61815))
REPRESENTATION_CONTEXT('','3D')
);
#61811=(
GEOMETRIC_REPRESENTATION_CONTEXT(3)
GLOBAL_UNCERTAINTY_ASSIGNED_CONTEXT((#61780))
GLOBAL_UNIT_ASSIGNED_CONTEXT((#61812,#61814,#61815))
REPRESENTATION_CONTEXT('','3D')
);
#61812=(
LENGTH_UNIT()
NAMED_UNIT(*)
SI_UNIT(.MILLI.,.METRE.)
);
#61814=(
NAMED_UNIT(*)
PLANE_ANGLE_UNIT()
SI_UNIT($,.RADIAN.)
);
#61815=(
NAMED_UNIT(*)
SI_UNIT($,.STERADIAN.)
SOLID_ANGLE_UNIT()
);
#61825=SHAPE_DEFINITION_REPRESENTATION(#61855,#61977);
#61855=PRODUCT_DEFINITION_SHAPE('',$,#62008);
#61977=SHAPE_REPRESENTATION('',(#34568),#61790);
#61998=PRODUCT_DEFINITION_CONTEXT('part definition',#62090,'design');
#62008=PRODUCT_DEFINITION('Electric Drive Motor','Electric Drive Motor',
#62038,#61998);
#62038=PRODUCT_DEFINITION_FORMATION('',$,#62101);
#62090=APPLICATION_CONTEXT('Managed model based 3d engineering');
#62091=PRODUCT_CONTEXT('part definition',#62090,'mechanical');
#62101=PRODUCT('Electric Drive Motor','Electric Drive Motor',$,(#62091));
#62136=COLOUR_RGB('Light Blue',0.38,0.62,0.78);
#62137=FILL_AREA_STYLE_COLOUR('',#62136);
#62138=FILL_AREA_STYLE('',(#62137));
#62139=SURFACE_STYLE_FILL_AREA(#62138);
#62140=SURFACE_SIDE_STYLE('',(#62139));
#62141=SURFACE_STYLE_USAGE(.BOTH.,#62140);
#62142=PRESENTATION_STYLE_ASSIGNMENT((#62141));
ENDSEC;
END-ISO-10303-21;
